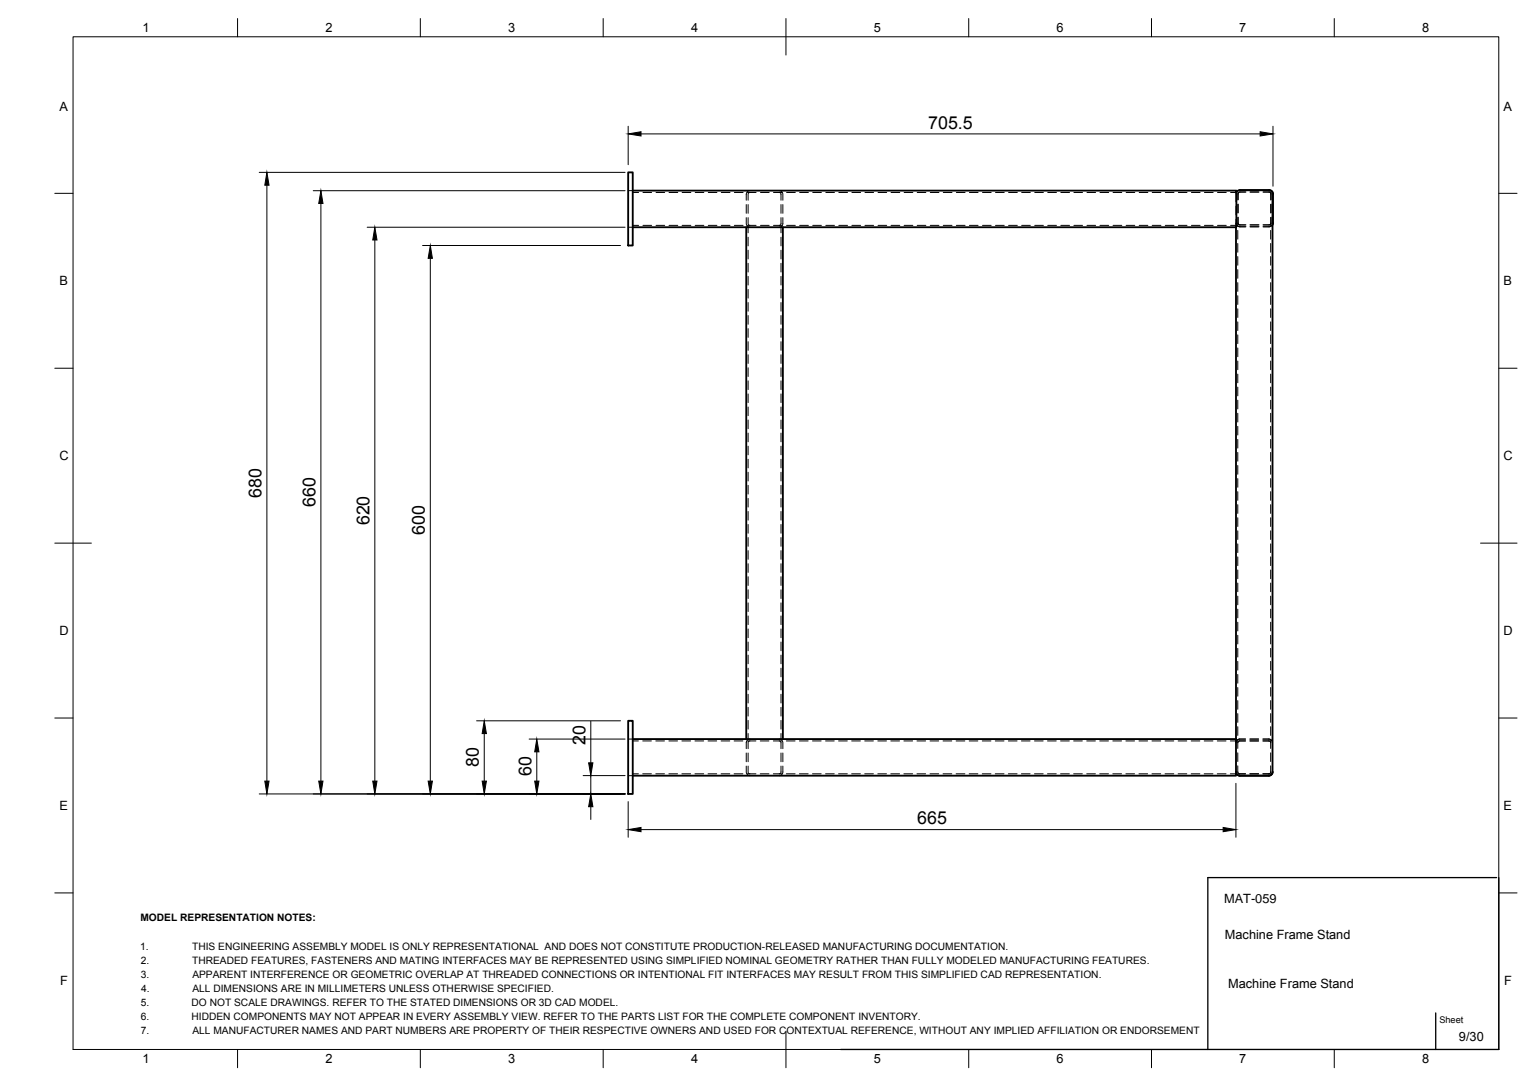
ISO-10303-21;
HEADER;
/* Generated by software containing ST-Developer
 * from STEP Tools, Inc. (www.steptools.com) 
 */

FILE_DESCRIPTION(
/* description */ ('', 'CAx-IF Rec.Pracs.---Representation and Presentation of Product Manufa
cturing Information (PMI)---4.0---2014-10-13'),
/* implementation_level */ '2;1');

FILE_NAME(
/* name */ 'Machine Frame Stand.step',
/* time_stamp */ '2026-10-28T23:00:48+01:00',
/* author */ (''),
/* organization */ (''),
/* preprocessor_version */ 'ST-DEVELOPER v20.2',
/* originating_system */ 'Autodesk Translation Framework v15.17.0.0',
/* authorisation */ '');

FILE_SCHEMA (('AP242_MANAGED_MODEL_BASED_3D_ENGINEERING_MIM_LF { 1 0 10303 442 2 1 4 }'));
ENDSEC;

DATA;
#10=MECHANICAL_DESIGN_GEOMETRIC_PRESENTATION_REPRESENTATION('',(#971,#972,#973,#974,#975,#976,#977,#978,#979,#980,#981,#982,#983,#984,#985),#61811);
#394=ELLIPSE('',#35329,5.65685424949238,4.);
#395=ELLIPSE('',#35330,5.65685424949238,4.);
#396=ELLIPSE('',#35331,5.65685424949238,4.);
#397=ELLIPSE('',#35332,5.65685424949238,4.);
#398=ELLIPSE('',#35333,2.82842712474619,2.);
#399=ELLIPSE('',#35334,2.82842712474619,2.);
#400=ELLIPSE('',#35335,2.82842712474619,2.);
#401=ELLIPSE('',#35336,2.82842712474619,2.);
#402=ELLIPSE('',#35339,2.82842712474716,2.);
#403=ELLIPSE('',#35342,2.82842712474716,2.);
#404=ELLIPSE('',#35344,5.65685424949433,4.);
#405=ELLIPSE('',#35346,5.65685424949433,4.);
#406=ELLIPSE('',#35349,5.65685424949433,4.);
#407=ELLIPSE('',#35350,5.65685424949433,4.);
#408=ELLIPSE('',#35351,2.82842712474716,2.);
#409=ELLIPSE('',#35352,2.82842712474716,2.);
#410=ELLIPSE('',#35363,5.65685424949238,4.);
#411=ELLIPSE('',#35364,5.65685424949238,4.);
#412=ELLIPSE('',#35365,5.65685424949238,4.);
#413=ELLIPSE('',#35366,5.65685424949238,4.);
#414=ELLIPSE('',#35367,2.82842712474619,2.);
#415=ELLIPSE('',#35368,2.82842712474619,2.);
#416=ELLIPSE('',#35369,2.82842712474619,2.);
#417=ELLIPSE('',#35370,2.82842712474619,2.);
#418=ELLIPSE('',#35373,2.82842712474716,2.);
#419=ELLIPSE('',#35376,2.82842712474716,2.);
#420=ELLIPSE('',#35378,5.65685424949433,4.);
#421=ELLIPSE('',#35381,5.65685424949433,4.);
#422=ELLIPSE('',#35384,5.65685424949433,4.);
#423=ELLIPSE('',#35385,5.65685424949433,4.);
#424=ELLIPSE('',#35386,2.82842712474716,2.);
#425=ELLIPSE('',#35387,2.82842712474716,2.);
#426=ELLIPSE('',#35397,5.65685424949043,4.);
#427=ELLIPSE('',#35398,5.65685424949043,4.);
#428=ELLIPSE('',#35399,5.65685424949043,4.);
#429=ELLIPSE('',#35400,5.65685424949043,4.);
#430=ELLIPSE('',#35401,2.82842712474521,2.);
#431=ELLIPSE('',#35402,2.82842712474521,2.);
#432=ELLIPSE('',#35403,2.82842712474521,2.);
#433=ELLIPSE('',#35404,2.82842712474521,2.);
#434=ELLIPSE('',#35407,2.82842712474521,2.);
#435=ELLIPSE('',#35410,2.82842712474521,2.);
#436=ELLIPSE('',#35413,5.65685424949043,4.);
#437=ELLIPSE('',#35416,5.65685424949043,4.);
#438=ELLIPSE('',#35418,5.65685424949043,4.);
#439=ELLIPSE('',#35419,5.65685424949043,4.);
#440=ELLIPSE('',#35420,2.82842712474521,2.);
#441=ELLIPSE('',#35421,2.82842712474521,2.);
#442=ELLIPSE('',#35431,5.65685424949238,4.);
#443=ELLIPSE('',#35432,5.65685424949238,4.);
#444=ELLIPSE('',#35433,5.65685424949238,4.);
#445=ELLIPSE('',#35434,5.65685424949238,4.);
#446=ELLIPSE('',#35435,2.82842712474619,2.);
#447=ELLIPSE('',#35436,2.82842712474619,2.);
#448=ELLIPSE('',#35437,2.82842712474619,2.);
#449=ELLIPSE('',#35438,2.82842712474619,2.);
#450=ELLIPSE('',#35441,2.82842712474619,2.);
#451=ELLIPSE('',#35444,2.82842712474619,2.);
#452=ELLIPSE('',#35447,5.65685424949238,4.);
#453=ELLIPSE('',#35450,5.65685424949238,4.);
#454=ELLIPSE('',#35452,5.65685424949238,4.);
#455=ELLIPSE('',#35453,5.65685424949238,4.);
#456=ELLIPSE('',#35454,2.82842712474619,2.);
#457=ELLIPSE('',#35455,2.82842712474619,2.);
#921=SHAPE_REPRESENTATION_RELATIONSHIP('SRR','None',#61979,#946);
#946=ADVANCED_BREP_SHAPE_REPRESENTATION('',(#1010,#1011,#1012,#1013,#1014,
#1015,#1016,#1017,#1018,#1019,#1020,#1021,#1022,#1023,#1024),#61792);
#971=STYLED_ITEM('',(#62135),#1010);
#972=STYLED_ITEM('',(#62135),#1011);
#973=STYLED_ITEM('',(#62135),#1012);
#974=STYLED_ITEM('',(#62135),#1013);
#975=STYLED_ITEM('',(#62135),#1014);
#976=STYLED_ITEM('',(#62135),#1015);
#977=STYLED_ITEM('',(#62135),#1016);
#978=STYLED_ITEM('',(#62135),#1017);
#979=STYLED_ITEM('',(#62135),#1018);
#980=STYLED_ITEM('',(#62135),#1019);
#981=STYLED_ITEM('',(#62135),#1020);
#982=STYLED_ITEM('',(#62135),#1021);
#983=STYLED_ITEM('',(#62135),#1022);
#984=STYLED_ITEM('',(#62135),#1023);
#985=STYLED_ITEM('',(#62135),#1024);
#1010=MANIFOLD_SOLID_BREP('Body1',#33801);
#1011=MANIFOLD_SOLID_BREP('Body2',#33802);
#1012=MANIFOLD_SOLID_BREP('Body3',#33803);
#1013=MANIFOLD_SOLID_BREP('Body4',#33804);
#1014=MANIFOLD_SOLID_BREP('Body5',#33805);
#1015=MANIFOLD_SOLID_BREP('Body6',#33806);
#1016=MANIFOLD_SOLID_BREP('Body7',#33807);
#1017=MANIFOLD_SOLID_BREP('Body8',#33808);
#1018=MANIFOLD_SOLID_BREP('Body9',#33809);
#1019=MANIFOLD_SOLID_BREP('Body10',#33810);
#1020=MANIFOLD_SOLID_BREP('Body11',#33811);
#1021=MANIFOLD_SOLID_BREP('Body12',#33812);
#1022=MANIFOLD_SOLID_BREP('Body13',#33813);
#1023=MANIFOLD_SOLID_BREP('Body14',#33814);
#1024=MANIFOLD_SOLID_BREP('Body15',#33815);
#1191=CYLINDRICAL_SURFACE('',#35193,2.);
#1192=CYLINDRICAL_SURFACE('',#35197,2.);
#1193=CYLINDRICAL_SURFACE('',#35201,4.);
#1194=CYLINDRICAL_SURFACE('',#35205,4.);
#1195=CYLINDRICAL_SURFACE('',#35209,2.);
#1196=CYLINDRICAL_SURFACE('',#35213,2.);
#1197=CYLINDRICAL_SURFACE('',#35217,4.);
#1198=CYLINDRICAL_SURFACE('',#35221,4.);
#1199=CYLINDRICAL_SURFACE('',#35227,2.);
#1200=CYLINDRICAL_SURFACE('',#35231,2.);
#1201=CYLINDRICAL_SURFACE('',#35235,4.);
#1202=CYLINDRICAL_SURFACE('',#35239,4.);
#1203=CYLINDRICAL_SURFACE('',#35243,2.);
#1204=CYLINDRICAL_SURFACE('',#35247,2.);
#1205=CYLINDRICAL_SURFACE('',#35251,4.);
#1206=CYLINDRICAL_SURFACE('',#35255,4.);
#1207=CYLINDRICAL_SURFACE('',#35261,2.);
#1208=CYLINDRICAL_SURFACE('',#35265,2.);
#1209=CYLINDRICAL_SURFACE('',#35269,4.);
#1210=CYLINDRICAL_SURFACE('',#35273,4.);
#1211=CYLINDRICAL_SURFACE('',#35277,2.);
#1212=CYLINDRICAL_SURFACE('',#35281,2.);
#1213=CYLINDRICAL_SURFACE('',#35285,4.);
#1214=CYLINDRICAL_SURFACE('',#35289,4.);
#1215=CYLINDRICAL_SURFACE('',#35295,2.);
#1216=CYLINDRICAL_SURFACE('',#35299,2.);
#1217=CYLINDRICAL_SURFACE('',#35303,4.);
#1218=CYLINDRICAL_SURFACE('',#35307,4.);
#1219=CYLINDRICAL_SURFACE('',#35311,2.);
#1220=CYLINDRICAL_SURFACE('',#35315,2.);
#1221=CYLINDRICAL_SURFACE('',#35319,4.);
#1222=CYLINDRICAL_SURFACE('',#35323,4.);
#1223=CYLINDRICAL_SURFACE('',#35338,2.);
#1224=CYLINDRICAL_SURFACE('',#35341,2.);
#1225=CYLINDRICAL_SURFACE('',#35343,4.);
#1226=CYLINDRICAL_SURFACE('',#35345,4.);
#1227=CYLINDRICAL_SURFACE('',#35354,4.);
#1228=CYLINDRICAL_SURFACE('',#35355,2.);
#1229=CYLINDRICAL_SURFACE('',#35357,2.);
#1230=CYLINDRICAL_SURFACE('',#35360,4.);
#1231=CYLINDRICAL_SURFACE('',#35372,2.);
#1232=CYLINDRICAL_SURFACE('',#35375,2.);
#1233=CYLINDRICAL_SURFACE('',#35377,4.);
#1234=CYLINDRICAL_SURFACE('',#35380,4.);
#1235=CYLINDRICAL_SURFACE('',#35389,4.);
#1236=CYLINDRICAL_SURFACE('',#35390,2.);
#1237=CYLINDRICAL_SURFACE('',#35392,2.);
#1238=CYLINDRICAL_SURFACE('',#35394,4.);
#1239=CYLINDRICAL_SURFACE('',#35406,2.);
#1240=CYLINDRICAL_SURFACE('',#35409,2.);
#1241=CYLINDRICAL_SURFACE('',#35412,4.);
#1242=CYLINDRICAL_SURFACE('',#35415,4.);
#1243=CYLINDRICAL_SURFACE('',#35424,2.);
#1244=CYLINDRICAL_SURFACE('',#35426,2.);
#1245=CYLINDRICAL_SURFACE('',#35427,4.);
#1246=CYLINDRICAL_SURFACE('',#35429,4.);
#1247=CYLINDRICAL_SURFACE('',#35440,2.);
#1248=CYLINDRICAL_SURFACE('',#35443,2.);
#1249=CYLINDRICAL_SURFACE('',#35446,4.);
#1250=CYLINDRICAL_SURFACE('',#35449,4.);
#1251=CYLINDRICAL_SURFACE('',#35458,2.);
#1252=CYLINDRICAL_SURFACE('',#35460,2.);
#1253=CYLINDRICAL_SURFACE('',#35461,4.);
#1254=CYLINDRICAL_SURFACE('',#35463,4.);
#1255=CYLINDRICAL_SURFACE('',#35465,2.);
#1256=CYLINDRICAL_SURFACE('',#35469,2.);
#1257=CYLINDRICAL_SURFACE('',#35473,4.);
#1258=CYLINDRICAL_SURFACE('',#35477,4.);
#1259=CYLINDRICAL_SURFACE('',#35481,2.);
#1260=CYLINDRICAL_SURFACE('',#35485,2.);
#1261=CYLINDRICAL_SURFACE('',#35489,4.);
#1262=CYLINDRICAL_SURFACE('',#35493,4.);
#1263=CYLINDRICAL_SURFACE('',#35499,2.);
#1264=CYLINDRICAL_SURFACE('',#35503,2.);
#1265=CYLINDRICAL_SURFACE('',#35507,4.);
#1266=CYLINDRICAL_SURFACE('',#35511,4.);
#1267=CYLINDRICAL_SURFACE('',#35515,2.);
#1268=CYLINDRICAL_SURFACE('',#35519,2.);
#1269=CYLINDRICAL_SURFACE('',#35523,4.);
#1270=CYLINDRICAL_SURFACE('',#35527,4.);
#1271=CYLINDRICAL_SURFACE('',#35533,2.);
#1272=CYLINDRICAL_SURFACE('',#35537,2.);
#1273=CYLINDRICAL_SURFACE('',#35541,4.);
#1274=CYLINDRICAL_SURFACE('',#35545,4.);
#1275=CYLINDRICAL_SURFACE('',#35549,2.);
#1276=CYLINDRICAL_SURFACE('',#35553,2.);
#1277=CYLINDRICAL_SURFACE('',#35557,4.);
#1278=CYLINDRICAL_SURFACE('',#35561,4.);
#1279=CYLINDRICAL_SURFACE('',#35566,4.);
#1280=CYLINDRICAL_SURFACE('',#35570,4.);
#1281=CYLINDRICAL_SURFACE('',#35574,4.);
#1282=CYLINDRICAL_SURFACE('',#35578,4.);
#1283=CYLINDRICAL_SURFACE('',#35582,24.0000000000018);
#1284=CYLINDRICAL_SURFACE('',#35586,24.0000000000018);
#1285=CYLINDRICAL_SURFACE('',#35590,24.0000000000018);
#1286=CYLINDRICAL_SURFACE('',#35594,24.0000000000018);
#1287=CYLINDRICAL_SURFACE('',#35600,4.);
#1288=CYLINDRICAL_SURFACE('',#35604,4.);
#1289=CYLINDRICAL_SURFACE('',#35608,4.);
#1290=CYLINDRICAL_SURFACE('',#35612,4.);
#1291=CYLINDRICAL_SURFACE('',#35616,24.0000000000018);
#1292=CYLINDRICAL_SURFACE('',#35620,24.0000000000018);
#1293=CYLINDRICAL_SURFACE('',#35624,24.0000000000018);
#1294=CYLINDRICAL_SURFACE('',#35628,24.0000000000018);
#1295=CYLINDRICAL_SURFACE('',#35634,4.);
#1296=CYLINDRICAL_SURFACE('',#35638,4.);
#1297=CYLINDRICAL_SURFACE('',#35642,4.);
#1298=CYLINDRICAL_SURFACE('',#35646,4.);
#1299=CYLINDRICAL_SURFACE('',#35650,24.0000000000018);
#1300=CYLINDRICAL_SURFACE('',#35654,24.0000000000018);
#1301=CYLINDRICAL_SURFACE('',#35658,24.0000000000018);
#1302=CYLINDRICAL_SURFACE('',#35662,24.0000000000018);
#1303=CYLINDRICAL_SURFACE('',#35668,4.);
#1304=CYLINDRICAL_SURFACE('',#35672,4.);
#1305=CYLINDRICAL_SURFACE('',#35676,4.);
#1306=CYLINDRICAL_SURFACE('',#35680,4.);
#1307=CYLINDRICAL_SURFACE('',#35684,24.0000000000018);
#1308=CYLINDRICAL_SURFACE('',#35688,24.0000000000018);
#1309=CYLINDRICAL_SURFACE('',#35692,24.0000000000018);
#1310=CYLINDRICAL_SURFACE('',#35696,24.0000000000018);
#1978=FACE_BOUND('',#6801,.T.);
#1979=FACE_BOUND('',#6803,.T.);
#1980=FACE_BOUND('',#6821,.T.);
#1981=FACE_BOUND('',#6823,.T.);
#1982=FACE_BOUND('',#6841,.T.);
#1983=FACE_BOUND('',#6843,.T.);
#1984=FACE_BOUND('',#6861,.T.);
#1985=FACE_BOUND('',#6863,.T.);
#1986=FACE_BOUND('',#6865,.T.);
#1987=FACE_BOUND('',#6874,.T.);
#1988=FACE_BOUND('',#6885,.T.);
#1989=FACE_BOUND('',#6895,.T.);
#1990=FACE_BOUND('',#6905,.T.);
#1991=FACE_BOUND('',#6915,.T.);
#1992=FACE_BOUND('',#6925,.T.);
#1993=FACE_BOUND('',#6935,.T.);
#1994=FACE_BOUND('',#6961,.T.);
#1995=FACE_BOUND('',#6963,.T.);
#1996=FACE_BOUND('',#6981,.T.);
#1997=FACE_BOUND('',#6983,.T.);
#1998=FACE_BOUND('',#7001,.T.);
#1999=FACE_BOUND('',#7003,.T.);
#2000=FACE_BOUND('',#7021,.T.);
#2001=FACE_BOUND('',#7023,.T.);
#2002=FACE_BOUND('',#7041,.T.);
#2003=FACE_BOUND('',#7043,.T.);
#2004=FACE_BOUND('',#7061,.T.);
#2005=FACE_BOUND('',#7063,.T.);
#2006=FACE_BOUND('',#7081,.T.);
#2007=FACE_BOUND('',#7083,.T.);
#2744=CIRCLE('',#35194,2.);
#2745=CIRCLE('',#35195,2.);
#2746=CIRCLE('',#35198,2.);
#2747=CIRCLE('',#35199,2.);
#2748=CIRCLE('',#35202,4.);
#2749=CIRCLE('',#35203,4.);
#2750=CIRCLE('',#35206,4.);
#2751=CIRCLE('',#35207,4.);
#2752=CIRCLE('',#35210,2.);
#2753=CIRCLE('',#35211,2.);
#2754=CIRCLE('',#35214,2.);
#2755=CIRCLE('',#35215,2.);
#2756=CIRCLE('',#35218,4.);
#2757=CIRCLE('',#35219,4.);
#2758=CIRCLE('',#35222,4.);
#2759=CIRCLE('',#35223,4.);
#2760=CIRCLE('',#35228,2.);
#2761=CIRCLE('',#35229,2.);
#2762=CIRCLE('',#35232,2.);
#2763=CIRCLE('',#35233,2.);
#2764=CIRCLE('',#35236,4.);
#2765=CIRCLE('',#35237,4.);
#2766=CIRCLE('',#35240,4.);
#2767=CIRCLE('',#35241,4.);
#2768=CIRCLE('',#35244,2.);
#2769=CIRCLE('',#35245,2.);
#2770=CIRCLE('',#35248,2.);
#2771=CIRCLE('',#35249,2.);
#2772=CIRCLE('',#35252,4.);
#2773=CIRCLE('',#35253,4.);
#2774=CIRCLE('',#35256,4.);
#2775=CIRCLE('',#35257,4.);
#2776=CIRCLE('',#35262,2.);
#2777=CIRCLE('',#35263,2.);
#2778=CIRCLE('',#35266,2.);
#2779=CIRCLE('',#35267,2.);
#2780=CIRCLE('',#35270,4.);
#2781=CIRCLE('',#35271,4.);
#2782=CIRCLE('',#35274,4.);
#2783=CIRCLE('',#35275,4.);
#2784=CIRCLE('',#35278,2.);
#2785=CIRCLE('',#35279,2.);
#2786=CIRCLE('',#35282,2.);
#2787=CIRCLE('',#35283,2.);
#2788=CIRCLE('',#35286,4.);
#2789=CIRCLE('',#35287,4.);
#2790=CIRCLE('',#35290,4.);
#2791=CIRCLE('',#35291,4.);
#2792=CIRCLE('',#35296,2.);
#2793=CIRCLE('',#35297,2.);
#2794=CIRCLE('',#35300,2.);
#2795=CIRCLE('',#35301,2.);
#2796=CIRCLE('',#35304,4.);
#2797=CIRCLE('',#35305,4.);
#2798=CIRCLE('',#35308,4.);
#2799=CIRCLE('',#35309,4.);
#2800=CIRCLE('',#35312,2.);
#2801=CIRCLE('',#35313,2.);
#2802=CIRCLE('',#35316,2.);
#2803=CIRCLE('',#35317,2.);
#2804=CIRCLE('',#35320,4.);
#2805=CIRCLE('',#35321,4.);
#2806=CIRCLE('',#35324,4.);
#2807=CIRCLE('',#35325,4.);
#2808=CIRCLE('',#35466,2.);
#2809=CIRCLE('',#35467,2.);
#2810=CIRCLE('',#35470,2.);
#2811=CIRCLE('',#35471,2.);
#2812=CIRCLE('',#35474,4.);
#2813=CIRCLE('',#35475,4.);
#2814=CIRCLE('',#35478,4.);
#2815=CIRCLE('',#35479,4.);
#2816=CIRCLE('',#35482,2.);
#2817=CIRCLE('',#35483,2.);
#2818=CIRCLE('',#35486,2.);
#2819=CIRCLE('',#35487,2.);
#2820=CIRCLE('',#35490,4.);
#2821=CIRCLE('',#35491,4.);
#2822=CIRCLE('',#35494,4.);
#2823=CIRCLE('',#35495,4.);
#2824=CIRCLE('',#35500,2.);
#2825=CIRCLE('',#35501,2.);
#2826=CIRCLE('',#35504,2.);
#2827=CIRCLE('',#35505,2.);
#2828=CIRCLE('',#35508,4.);
#2829=CIRCLE('',#35509,4.);
#2830=CIRCLE('',#35512,4.);
#2831=CIRCLE('',#35513,4.);
#2832=CIRCLE('',#35516,2.);
#2833=CIRCLE('',#35517,2.);
#2834=CIRCLE('',#35520,2.);
#2835=CIRCLE('',#35521,2.);
#2836=CIRCLE('',#35524,4.);
#2837=CIRCLE('',#35525,4.);
#2838=CIRCLE('',#35528,4.);
#2839=CIRCLE('',#35529,4.);
#2840=CIRCLE('',#35534,2.);
#2841=CIRCLE('',#35535,2.);
#2842=CIRCLE('',#35538,2.);
#2843=CIRCLE('',#35539,2.);
#2844=CIRCLE('',#35542,4.);
#2845=CIRCLE('',#35543,4.);
#2846=CIRCLE('',#35546,4.);
#2847=CIRCLE('',#35547,4.);
#2848=CIRCLE('',#35550,2.);
#2849=CIRCLE('',#35551,2.);
#2850=CIRCLE('',#35554,2.);
#2851=CIRCLE('',#35555,2.);
#2852=CIRCLE('',#35558,4.);
#2853=CIRCLE('',#35559,4.);
#2854=CIRCLE('',#35562,4.);
#2855=CIRCLE('',#35563,4.);
#2856=CIRCLE('',#35567,4.);
#2857=CIRCLE('',#35568,4.);
#2858=CIRCLE('',#35571,4.);
#2859=CIRCLE('',#35572,4.);
#2860=CIRCLE('',#35575,4.);
#2861=CIRCLE('',#35576,4.);
#2862=CIRCLE('',#35579,4.);
#2863=CIRCLE('',#35580,4.);
#2864=CIRCLE('',#35583,24.0000000000018);
#2865=CIRCLE('',#35584,24.0000000000018);
#2866=CIRCLE('',#35587,24.0000000000018);
#2867=CIRCLE('',#35588,24.0000000000018);
#2868=CIRCLE('',#35591,24.0000000000018);
#2869=CIRCLE('',#35592,24.0000000000018);
#2870=CIRCLE('',#35595,24.0000000000018);
#2871=CIRCLE('',#35596,24.0000000000018);
#2872=CIRCLE('',#35601,4.);
#2873=CIRCLE('',#35602,4.);
#2874=CIRCLE('',#35605,4.);
#2875=CIRCLE('',#35606,4.);
#2876=CIRCLE('',#35609,4.);
#2877=CIRCLE('',#35610,4.);
#2878=CIRCLE('',#35613,4.);
#2879=CIRCLE('',#35614,4.);
#2880=CIRCLE('',#35617,24.0000000000018);
#2881=CIRCLE('',#35618,24.0000000000018);
#2882=CIRCLE('',#35621,24.0000000000018);
#2883=CIRCLE('',#35622,24.0000000000018);
#2884=CIRCLE('',#35625,24.0000000000018);
#2885=CIRCLE('',#35626,24.0000000000018);
#2886=CIRCLE('',#35629,24.0000000000018);
#2887=CIRCLE('',#35630,24.0000000000018);
#2888=CIRCLE('',#35635,4.);
#2889=CIRCLE('',#35636,4.);
#2890=CIRCLE('',#35639,4.);
#2891=CIRCLE('',#35640,4.);
#2892=CIRCLE('',#35643,4.);
#2893=CIRCLE('',#35644,4.);
#2894=CIRCLE('',#35647,4.);
#2895=CIRCLE('',#35648,4.);
#2896=CIRCLE('',#35651,24.0000000000018);
#2897=CIRCLE('',#35652,24.0000000000018);
#2898=CIRCLE('',#35655,24.0000000000018);
#2899=CIRCLE('',#35656,24.0000000000018);
#2900=CIRCLE('',#35659,24.0000000000018);
#2901=CIRCLE('',#35660,24.0000000000018);
#2902=CIRCLE('',#35663,24.0000000000018);
#2903=CIRCLE('',#35664,24.0000000000018);
#2904=CIRCLE('',#35669,4.);
#2905=CIRCLE('',#35670,4.);
#2906=CIRCLE('',#35673,4.);
#2907=CIRCLE('',#35674,4.);
#2908=CIRCLE('',#35677,4.);
#2909=CIRCLE('',#35678,4.);
#2910=CIRCLE('',#35681,4.);
#2911=CIRCLE('',#35682,4.);
#2912=CIRCLE('',#35685,24.0000000000018);
#2913=CIRCLE('',#35686,24.0000000000018);
#2914=CIRCLE('',#35689,24.0000000000018);
#2915=CIRCLE('',#35690,24.0000000000018);
#2916=CIRCLE('',#35693,24.0000000000018);
#2917=CIRCLE('',#35694,24.0000000000018);
#2918=CIRCLE('',#35697,24.0000000000018);
#2919=CIRCLE('',#35698,24.0000000000018);
#4806=FACE_OUTER_BOUND('',#6784,.T.);
#4807=FACE_OUTER_BOUND('',#6785,.T.);
#4808=FACE_OUTER_BOUND('',#6786,.T.);
#4809=FACE_OUTER_BOUND('',#6787,.T.);
#4810=FACE_OUTER_BOUND('',#6788,.T.);
#4811=FACE_OUTER_BOUND('',#6789,.T.);
#4812=FACE_OUTER_BOUND('',#6790,.T.);
#4813=FACE_OUTER_BOUND('',#6791,.T.);
#4814=FACE_OUTER_BOUND('',#6792,.T.);
#4815=FACE_OUTER_BOUND('',#6793,.T.);
#4816=FACE_OUTER_BOUND('',#6794,.T.);
#4817=FACE_OUTER_BOUND('',#6795,.T.);
#4818=FACE_OUTER_BOUND('',#6796,.T.);
#4819=FACE_OUTER_BOUND('',#6797,.T.);
#4820=FACE_OUTER_BOUND('',#6798,.T.);
#4821=FACE_OUTER_BOUND('',#6799,.T.);
#4822=FACE_OUTER_BOUND('',#6800,.T.);
#4823=FACE_OUTER_BOUND('',#6802,.T.);
#4824=FACE_OUTER_BOUND('',#6804,.T.);
#4825=FACE_OUTER_BOUND('',#6805,.T.);
#4826=FACE_OUTER_BOUND('',#6806,.T.);
#4827=FACE_OUTER_BOUND('',#6807,.T.);
#4828=FACE_OUTER_BOUND('',#6808,.T.);
#4829=FACE_OUTER_BOUND('',#6809,.T.);
#4830=FACE_OUTER_BOUND('',#6810,.T.);
#4831=FACE_OUTER_BOUND('',#6811,.T.);
#4832=FACE_OUTER_BOUND('',#6812,.T.);
#4833=FACE_OUTER_BOUND('',#6813,.T.);
#4834=FACE_OUTER_BOUND('',#6814,.T.);
#4835=FACE_OUTER_BOUND('',#6815,.T.);
#4836=FACE_OUTER_BOUND('',#6816,.T.);
#4837=FACE_OUTER_BOUND('',#6817,.T.);
#4838=FACE_OUTER_BOUND('',#6818,.T.);
#4839=FACE_OUTER_BOUND('',#6819,.T.);
#4840=FACE_OUTER_BOUND('',#6820,.T.);
#4841=FACE_OUTER_BOUND('',#6822,.T.);
#4842=FACE_OUTER_BOUND('',#6824,.T.);
#4843=FACE_OUTER_BOUND('',#6825,.T.);
#4844=FACE_OUTER_BOUND('',#6826,.T.);
#4845=FACE_OUTER_BOUND('',#6827,.T.);
#4846=FACE_OUTER_BOUND('',#6828,.T.);
#4847=FACE_OUTER_BOUND('',#6829,.T.);
#4848=FACE_OUTER_BOUND('',#6830,.T.);
#4849=FACE_OUTER_BOUND('',#6831,.T.);
#4850=FACE_OUTER_BOUND('',#6832,.T.);
#4851=FACE_OUTER_BOUND('',#6833,.T.);
#4852=FACE_OUTER_BOUND('',#6834,.T.);
#4853=FACE_OUTER_BOUND('',#6835,.T.);
#4854=FACE_OUTER_BOUND('',#6836,.T.);
#4855=FACE_OUTER_BOUND('',#6837,.T.);
#4856=FACE_OUTER_BOUND('',#6838,.T.);
#4857=FACE_OUTER_BOUND('',#6839,.T.);
#4858=FACE_OUTER_BOUND('',#6840,.T.);
#4859=FACE_OUTER_BOUND('',#6842,.T.);
#4860=FACE_OUTER_BOUND('',#6844,.T.);
#4861=FACE_OUTER_BOUND('',#6845,.T.);
#4862=FACE_OUTER_BOUND('',#6846,.T.);
#4863=FACE_OUTER_BOUND('',#6847,.T.);
#4864=FACE_OUTER_BOUND('',#6848,.T.);
#4865=FACE_OUTER_BOUND('',#6849,.T.);
#4866=FACE_OUTER_BOUND('',#6850,.T.);
#4867=FACE_OUTER_BOUND('',#6851,.T.);
#4868=FACE_OUTER_BOUND('',#6852,.T.);
#4869=FACE_OUTER_BOUND('',#6853,.T.);
#4870=FACE_OUTER_BOUND('',#6854,.T.);
#4871=FACE_OUTER_BOUND('',#6855,.T.);
#4872=FACE_OUTER_BOUND('',#6856,.T.);
#4873=FACE_OUTER_BOUND('',#6857,.T.);
#4874=FACE_OUTER_BOUND('',#6858,.T.);
#4875=FACE_OUTER_BOUND('',#6859,.T.);
#4876=FACE_OUTER_BOUND('',#6860,.T.);
#4877=FACE_OUTER_BOUND('',#6862,.T.);
#4878=FACE_OUTER_BOUND('',#6864,.T.);
#4879=FACE_OUTER_BOUND('',#6866,.T.);
#4880=FACE_OUTER_BOUND('',#6867,.T.);
#4881=FACE_OUTER_BOUND('',#6868,.T.);
#4882=FACE_OUTER_BOUND('',#6869,.T.);
#4883=FACE_OUTER_BOUND('',#6870,.T.);
#4884=FACE_OUTER_BOUND('',#6871,.T.);
#4885=FACE_OUTER_BOUND('',#6872,.T.);
#4886=FACE_OUTER_BOUND('',#6873,.T.);
#4887=FACE_OUTER_BOUND('',#6875,.T.);
#4888=FACE_OUTER_BOUND('',#6876,.T.);
#4889=FACE_OUTER_BOUND('',#6877,.T.);
#4890=FACE_OUTER_BOUND('',#6878,.T.);
#4891=FACE_OUTER_BOUND('',#6879,.T.);
#4892=FACE_OUTER_BOUND('',#6880,.T.);
#4893=FACE_OUTER_BOUND('',#6881,.T.);
#4894=FACE_OUTER_BOUND('',#6882,.T.);
#4895=FACE_OUTER_BOUND('',#6883,.T.);
#4896=FACE_OUTER_BOUND('',#6884,.T.);
#4897=FACE_OUTER_BOUND('',#6886,.T.);
#4898=FACE_OUTER_BOUND('',#6887,.T.);
#4899=FACE_OUTER_BOUND('',#6888,.T.);
#4900=FACE_OUTER_BOUND('',#6889,.T.);
#4901=FACE_OUTER_BOUND('',#6890,.T.);
#4902=FACE_OUTER_BOUND('',#6891,.T.);
#4903=FACE_OUTER_BOUND('',#6892,.T.);
#4904=FACE_OUTER_BOUND('',#6893,.T.);
#4905=FACE_OUTER_BOUND('',#6894,.T.);
#4906=FACE_OUTER_BOUND('',#6896,.T.);
#4907=FACE_OUTER_BOUND('',#6897,.T.);
#4908=FACE_OUTER_BOUND('',#6898,.T.);
#4909=FACE_OUTER_BOUND('',#6899,.T.);
#4910=FACE_OUTER_BOUND('',#6900,.T.);
#4911=FACE_OUTER_BOUND('',#6901,.T.);
#4912=FACE_OUTER_BOUND('',#6902,.T.);
#4913=FACE_OUTER_BOUND('',#6903,.T.);
#4914=FACE_OUTER_BOUND('',#6904,.T.);
#4915=FACE_OUTER_BOUND('',#6906,.T.);
#4916=FACE_OUTER_BOUND('',#6907,.T.);
#4917=FACE_OUTER_BOUND('',#6908,.T.);
#4918=FACE_OUTER_BOUND('',#6909,.T.);
#4919=FACE_OUTER_BOUND('',#6910,.T.);
#4920=FACE_OUTER_BOUND('',#6911,.T.);
#4921=FACE_OUTER_BOUND('',#6912,.T.);
#4922=FACE_OUTER_BOUND('',#6913,.T.);
#4923=FACE_OUTER_BOUND('',#6914,.T.);
#4924=FACE_OUTER_BOUND('',#6916,.T.);
#4925=FACE_OUTER_BOUND('',#6917,.T.);
#4926=FACE_OUTER_BOUND('',#6918,.T.);
#4927=FACE_OUTER_BOUND('',#6919,.T.);
#4928=FACE_OUTER_BOUND('',#6920,.T.);
#4929=FACE_OUTER_BOUND('',#6921,.T.);
#4930=FACE_OUTER_BOUND('',#6922,.T.);
#4931=FACE_OUTER_BOUND('',#6923,.T.);
#4932=FACE_OUTER_BOUND('',#6924,.T.);
#4933=FACE_OUTER_BOUND('',#6926,.T.);
#4934=FACE_OUTER_BOUND('',#6927,.T.);
#4935=FACE_OUTER_BOUND('',#6928,.T.);
#4936=FACE_OUTER_BOUND('',#6929,.T.);
#4937=FACE_OUTER_BOUND('',#6930,.T.);
#4938=FACE_OUTER_BOUND('',#6931,.T.);
#4939=FACE_OUTER_BOUND('',#6932,.T.);
#4940=FACE_OUTER_BOUND('',#6933,.T.);
#4941=FACE_OUTER_BOUND('',#6934,.T.);
#4942=FACE_OUTER_BOUND('',#6936,.T.);
#4943=FACE_OUTER_BOUND('',#6937,.T.);
#4944=FACE_OUTER_BOUND('',#6938,.T.);
#4945=FACE_OUTER_BOUND('',#6939,.T.);
#4946=FACE_OUTER_BOUND('',#6940,.T.);
#4947=FACE_OUTER_BOUND('',#6941,.T.);
#4948=FACE_OUTER_BOUND('',#6942,.T.);
#4949=FACE_OUTER_BOUND('',#6943,.T.);
#4950=FACE_OUTER_BOUND('',#6944,.T.);
#4951=FACE_OUTER_BOUND('',#6945,.T.);
#4952=FACE_OUTER_BOUND('',#6946,.T.);
#4953=FACE_OUTER_BOUND('',#6947,.T.);
#4954=FACE_OUTER_BOUND('',#6948,.T.);
#4955=FACE_OUTER_BOUND('',#6949,.T.);
#4956=FACE_OUTER_BOUND('',#6950,.T.);
#4957=FACE_OUTER_BOUND('',#6951,.T.);
#4958=FACE_OUTER_BOUND('',#6952,.T.);
#4959=FACE_OUTER_BOUND('',#6953,.T.);
#4960=FACE_OUTER_BOUND('',#6954,.T.);
#4961=FACE_OUTER_BOUND('',#6955,.T.);
#4962=FACE_OUTER_BOUND('',#6956,.T.);
#4963=FACE_OUTER_BOUND('',#6957,.T.);
#4964=FACE_OUTER_BOUND('',#6958,.T.);
#4965=FACE_OUTER_BOUND('',#6959,.T.);
#4966=FACE_OUTER_BOUND('',#6960,.T.);
#4967=FACE_OUTER_BOUND('',#6962,.T.);
#4968=FACE_OUTER_BOUND('',#6964,.T.);
#4969=FACE_OUTER_BOUND('',#6965,.T.);
#4970=FACE_OUTER_BOUND('',#6966,.T.);
#4971=FACE_OUTER_BOUND('',#6967,.T.);
#4972=FACE_OUTER_BOUND('',#6968,.T.);
#4973=FACE_OUTER_BOUND('',#6969,.T.);
#4974=FACE_OUTER_BOUND('',#6970,.T.);
#4975=FACE_OUTER_BOUND('',#6971,.T.);
#4976=FACE_OUTER_BOUND('',#6972,.T.);
#4977=FACE_OUTER_BOUND('',#6973,.T.);
#4978=FACE_OUTER_BOUND('',#6974,.T.);
#4979=FACE_OUTER_BOUND('',#6975,.T.);
#4980=FACE_OUTER_BOUND('',#6976,.T.);
#4981=FACE_OUTER_BOUND('',#6977,.T.);
#4982=FACE_OUTER_BOUND('',#6978,.T.);
#4983=FACE_OUTER_BOUND('',#6979,.T.);
#4984=FACE_OUTER_BOUND('',#6980,.T.);
#4985=FACE_OUTER_BOUND('',#6982,.T.);
#4986=FACE_OUTER_BOUND('',#6984,.T.);
#4987=FACE_OUTER_BOUND('',#6985,.T.);
#4988=FACE_OUTER_BOUND('',#6986,.T.);
#4989=FACE_OUTER_BOUND('',#6987,.T.);
#4990=FACE_OUTER_BOUND('',#6988,.T.);
#4991=FACE_OUTER_BOUND('',#6989,.T.);
#4992=FACE_OUTER_BOUND('',#6990,.T.);
#4993=FACE_OUTER_BOUND('',#6991,.T.);
#4994=FACE_OUTER_BOUND('',#6992,.T.);
#4995=FACE_OUTER_BOUND('',#6993,.T.);
#4996=FACE_OUTER_BOUND('',#6994,.T.);
#4997=FACE_OUTER_BOUND('',#6995,.T.);
#4998=FACE_OUTER_BOUND('',#6996,.T.);
#4999=FACE_OUTER_BOUND('',#6997,.T.);
#5000=FACE_OUTER_BOUND('',#6998,.T.);
#5001=FACE_OUTER_BOUND('',#6999,.T.);
#5002=FACE_OUTER_BOUND('',#7000,.T.);
#5003=FACE_OUTER_BOUND('',#7002,.T.);
#5004=FACE_OUTER_BOUND('',#7004,.T.);
#5005=FACE_OUTER_BOUND('',#7005,.T.);
#5006=FACE_OUTER_BOUND('',#7006,.T.);
#5007=FACE_OUTER_BOUND('',#7007,.T.);
#5008=FACE_OUTER_BOUND('',#7008,.T.);
#5009=FACE_OUTER_BOUND('',#7009,.T.);
#5010=FACE_OUTER_BOUND('',#7010,.T.);
#5011=FACE_OUTER_BOUND('',#7011,.T.);
#5012=FACE_OUTER_BOUND('',#7012,.T.);
#5013=FACE_OUTER_BOUND('',#7013,.T.);
#5014=FACE_OUTER_BOUND('',#7014,.T.);
#5015=FACE_OUTER_BOUND('',#7015,.T.);
#5016=FACE_OUTER_BOUND('',#7016,.T.);
#5017=FACE_OUTER_BOUND('',#7017,.T.);
#5018=FACE_OUTER_BOUND('',#7018,.T.);
#5019=FACE_OUTER_BOUND('',#7019,.T.);
#5020=FACE_OUTER_BOUND('',#7020,.T.);
#5021=FACE_OUTER_BOUND('',#7022,.T.);
#5022=FACE_OUTER_BOUND('',#7024,.T.);
#5023=FACE_OUTER_BOUND('',#7025,.T.);
#5024=FACE_OUTER_BOUND('',#7026,.T.);
#5025=FACE_OUTER_BOUND('',#7027,.T.);
#5026=FACE_OUTER_BOUND('',#7028,.T.);
#5027=FACE_OUTER_BOUND('',#7029,.T.);
#5028=FACE_OUTER_BOUND('',#7030,.T.);
#5029=FACE_OUTER_BOUND('',#7031,.T.);
#5030=FACE_OUTER_BOUND('',#7032,.T.);
#5031=FACE_OUTER_BOUND('',#7033,.T.);
#5032=FACE_OUTER_BOUND('',#7034,.T.);
#5033=FACE_OUTER_BOUND('',#7035,.T.);
#5034=FACE_OUTER_BOUND('',#7036,.T.);
#5035=FACE_OUTER_BOUND('',#7037,.T.);
#5036=FACE_OUTER_BOUND('',#7038,.T.);
#5037=FACE_OUTER_BOUND('',#7039,.T.);
#5038=FACE_OUTER_BOUND('',#7040,.T.);
#5039=FACE_OUTER_BOUND('',#7042,.T.);
#5040=FACE_OUTER_BOUND('',#7044,.T.);
#5041=FACE_OUTER_BOUND('',#7045,.T.);
#5042=FACE_OUTER_BOUND('',#7046,.T.);
#5043=FACE_OUTER_BOUND('',#7047,.T.);
#5044=FACE_OUTER_BOUND('',#7048,.T.);
#5045=FACE_OUTER_BOUND('',#7049,.T.);
#5046=FACE_OUTER_BOUND('',#7050,.T.);
#5047=FACE_OUTER_BOUND('',#7051,.T.);
#5048=FACE_OUTER_BOUND('',#7052,.T.);
#5049=FACE_OUTER_BOUND('',#7053,.T.);
#5050=FACE_OUTER_BOUND('',#7054,.T.);
#5051=FACE_OUTER_BOUND('',#7055,.T.);
#5052=FACE_OUTER_BOUND('',#7056,.T.);
#5053=FACE_OUTER_BOUND('',#7057,.T.);
#5054=FACE_OUTER_BOUND('',#7058,.T.);
#5055=FACE_OUTER_BOUND('',#7059,.T.);
#5056=FACE_OUTER_BOUND('',#7060,.T.);
#5057=FACE_OUTER_BOUND('',#7062,.T.);
#5058=FACE_OUTER_BOUND('',#7064,.T.);
#5059=FACE_OUTER_BOUND('',#7065,.T.);
#5060=FACE_OUTER_BOUND('',#7066,.T.);
#5061=FACE_OUTER_BOUND('',#7067,.T.);
#5062=FACE_OUTER_BOUND('',#7068,.T.);
#5063=FACE_OUTER_BOUND('',#7069,.T.);
#5064=FACE_OUTER_BOUND('',#7070,.T.);
#5065=FACE_OUTER_BOUND('',#7071,.T.);
#5066=FACE_OUTER_BOUND('',#7072,.T.);
#5067=FACE_OUTER_BOUND('',#7073,.T.);
#5068=FACE_OUTER_BOUND('',#7074,.T.);
#5069=FACE_OUTER_BOUND('',#7075,.T.);
#5070=FACE_OUTER_BOUND('',#7076,.T.);
#5071=FACE_OUTER_BOUND('',#7077,.T.);
#5072=FACE_OUTER_BOUND('',#7078,.T.);
#5073=FACE_OUTER_BOUND('',#7079,.T.);
#5074=FACE_OUTER_BOUND('',#7080,.T.);
#5075=FACE_OUTER_BOUND('',#7082,.T.);
#6784=EDGE_LOOP('',(#24214,#24215,#24216,#24217));
#6785=EDGE_LOOP('',(#24218,#24219,#24220,#24221));
#6786=EDGE_LOOP('',(#24222,#24223,#24224,#24225));
#6787=EDGE_LOOP('',(#24226,#24227,#24228,#24229));
#6788=EDGE_LOOP('',(#24230,#24231,#24232,#24233));
#6789=EDGE_LOOP('',(#24234,#24235,#24236,#24237));
#6790=EDGE_LOOP('',(#24238,#24239,#24240,#24241));
#6791=EDGE_LOOP('',(#24242,#24243,#24244,#24245));
#6792=EDGE_LOOP('',(#24246,#24247,#24248,#24249));
#6793=EDGE_LOOP('',(#24250,#24251,#24252,#24253));
#6794=EDGE_LOOP('',(#24254,#24255,#24256,#24257));
#6795=EDGE_LOOP('',(#24258,#24259,#24260,#24261));
#6796=EDGE_LOOP('',(#24262,#24263,#24264,#24265));
#6797=EDGE_LOOP('',(#24266,#24267,#24268,#24269));
#6798=EDGE_LOOP('',(#24270,#24271,#24272,#24273));
#6799=EDGE_LOOP('',(#24274,#24275,#24276,#24277));
#6800=EDGE_LOOP('',(#24278,#24279,#24280,#24281,#24282,#24283,#24284,#24285));
#6801=EDGE_LOOP('',(#24286,#24287,#24288,#24289,#24290,#24291,#24292,#24293));
#6802=EDGE_LOOP('',(#24294,#24295,#24296,#24297,#24298,#24299,#24300,#24301));
#6803=EDGE_LOOP('',(#24302,#24303,#24304,#24305,#24306,#24307,#24308,#24309));
#6804=EDGE_LOOP('',(#24310,#24311,#24312,#24313));
#6805=EDGE_LOOP('',(#24314,#24315,#24316,#24317));
#6806=EDGE_LOOP('',(#24318,#24319,#24320,#24321));
#6807=EDGE_LOOP('',(#24322,#24323,#24324,#24325));
#6808=EDGE_LOOP('',(#24326,#24327,#24328,#24329));
#6809=EDGE_LOOP('',(#24330,#24331,#24332,#24333));
#6810=EDGE_LOOP('',(#24334,#24335,#24336,#24337));
#6811=EDGE_LOOP('',(#24338,#24339,#24340,#24341));
#6812=EDGE_LOOP('',(#24342,#24343,#24344,#24345));
#6813=EDGE_LOOP('',(#24346,#24347,#24348,#24349));
#6814=EDGE_LOOP('',(#24350,#24351,#24352,#24353));
#6815=EDGE_LOOP('',(#24354,#24355,#24356,#24357));
#6816=EDGE_LOOP('',(#24358,#24359,#24360,#24361));
#6817=EDGE_LOOP('',(#24362,#24363,#24364,#24365));
#6818=EDGE_LOOP('',(#24366,#24367,#24368,#24369));
#6819=EDGE_LOOP('',(#24370,#24371,#24372,#24373));
#6820=EDGE_LOOP('',(#24374,#24375,#24376,#24377,#24378,#24379,#24380,#24381));
#6821=EDGE_LOOP('',(#24382,#24383,#24384,#24385,#24386,#24387,#24388,#24389));
#6822=EDGE_LOOP('',(#24390,#24391,#24392,#24393,#24394,#24395,#24396,#24397));
#6823=EDGE_LOOP('',(#24398,#24399,#24400,#24401,#24402,#24403,#24404,#24405));
#6824=EDGE_LOOP('',(#24406,#24407,#24408,#24409));
#6825=EDGE_LOOP('',(#24410,#24411,#24412,#24413));
#6826=EDGE_LOOP('',(#24414,#24415,#24416,#24417));
#6827=EDGE_LOOP('',(#24418,#24419,#24420,#24421));
#6828=EDGE_LOOP('',(#24422,#24423,#24424,#24425));
#6829=EDGE_LOOP('',(#24426,#24427,#24428,#24429));
#6830=EDGE_LOOP('',(#24430,#24431,#24432,#24433));
#6831=EDGE_LOOP('',(#24434,#24435,#24436,#24437));
#6832=EDGE_LOOP('',(#24438,#24439,#24440,#24441));
#6833=EDGE_LOOP('',(#24442,#24443,#24444,#24445));
#6834=EDGE_LOOP('',(#24446,#24447,#24448,#24449));
#6835=EDGE_LOOP('',(#24450,#24451,#24452,#24453));
#6836=EDGE_LOOP('',(#24454,#24455,#24456,#24457));
#6837=EDGE_LOOP('',(#24458,#24459,#24460,#24461));
#6838=EDGE_LOOP('',(#24462,#24463,#24464,#24465));
#6839=EDGE_LOOP('',(#24466,#24467,#24468,#24469));
#6840=EDGE_LOOP('',(#24470,#24471,#24472,#24473,#24474,#24475,#24476,#24477));
#6841=EDGE_LOOP('',(#24478,#24479,#24480,#24481,#24482,#24483,#24484,#24485));
#6842=EDGE_LOOP('',(#24486,#24487,#24488,#24489,#24490,#24491,#24492,#24493));
#6843=EDGE_LOOP('',(#24494,#24495,#24496,#24497,#24498,#24499,#24500,#24501));
#6844=EDGE_LOOP('',(#24502,#24503,#24504,#24505));
#6845=EDGE_LOOP('',(#24506,#24507,#24508,#24509));
#6846=EDGE_LOOP('',(#24510,#24511,#24512,#24513));
#6847=EDGE_LOOP('',(#24514,#24515,#24516,#24517));
#6848=EDGE_LOOP('',(#24518,#24519,#24520,#24521));
#6849=EDGE_LOOP('',(#24522,#24523,#24524,#24525));
#6850=EDGE_LOOP('',(#24526,#24527,#24528,#24529));
#6851=EDGE_LOOP('',(#24530,#24531,#24532,#24533));
#6852=EDGE_LOOP('',(#24534,#24535,#24536,#24537));
#6853=EDGE_LOOP('',(#24538,#24539,#24540,#24541));
#6854=EDGE_LOOP('',(#24542,#24543,#24544,#24545));
#6855=EDGE_LOOP('',(#24546,#24547,#24548,#24549));
#6856=EDGE_LOOP('',(#24550,#24551,#24552,#24553));
#6857=EDGE_LOOP('',(#24554,#24555,#24556,#24557));
#6858=EDGE_LOOP('',(#24558,#24559,#24560,#24561));
#6859=EDGE_LOOP('',(#24562,#24563,#24564,#24565));
#6860=EDGE_LOOP('',(#24566,#24567,#24568,#24569,#24570,#24571,#24572,#24573));
#6861=EDGE_LOOP('',(#24574,#24575,#24576,#24577,#24578,#24579,#24580,#24581));
#6862=EDGE_LOOP('',(#24582,#24583,#24584,#24585,#24586,#24587,#24588,#24589));
#6863=EDGE_LOOP('',(#24590,#24591,#24592,#24593,#24594,#24595,#24596,#24597));
#6864=EDGE_LOOP('',(#24598,#24599,#24600,#24601,#24602,#24603,#24604,#24605));
#6865=EDGE_LOOP('',(#24606,#24607,#24608,#24609,#24610,#24611,#24612,#24613));
#6866=EDGE_LOOP('',(#24614,#24615,#24616,#24617));
#6867=EDGE_LOOP('',(#24618,#24619,#24620,#24621));
#6868=EDGE_LOOP('',(#24622,#24623,#24624,#24625));
#6869=EDGE_LOOP('',(#24626,#24627,#24628,#24629));
#6870=EDGE_LOOP('',(#24630,#24631,#24632,#24633));
#6871=EDGE_LOOP('',(#24634,#24635,#24636,#24637));
#6872=EDGE_LOOP('',(#24638,#24639,#24640,#24641));
#6873=EDGE_LOOP('',(#24642,#24643,#24644,#24645,#24646,#24647,#24648,#24649));
#6874=EDGE_LOOP('',(#24650,#24651,#24652,#24653,#24654,#24655,#24656,#24657));
#6875=EDGE_LOOP('',(#24658,#24659,#24660,#24661));
#6876=EDGE_LOOP('',(#24662,#24663,#24664,#24665));
#6877=EDGE_LOOP('',(#24666,#24667,#24668,#24669));
#6878=EDGE_LOOP('',(#24670,#24671,#24672,#24673));
#6879=EDGE_LOOP('',(#24674,#24675,#24676,#24677));
#6880=EDGE_LOOP('',(#24678,#24679,#24680,#24681));
#6881=EDGE_LOOP('',(#24682,#24683,#24684,#24685));
#6882=EDGE_LOOP('',(#24686,#24687,#24688,#24689));
#6883=EDGE_LOOP('',(#24690,#24691,#24692,#24693));
#6884=EDGE_LOOP('',(#24694,#24695,#24696,#24697,#24698,#24699,#24700,#24701));
#6885=EDGE_LOOP('',(#24702,#24703,#24704,#24705,#24706,#24707,#24708,#24709));
#6886=EDGE_LOOP('',(#24710,#24711,#24712,#24713));
#6887=EDGE_LOOP('',(#24714,#24715,#24716,#24717));
#6888=EDGE_LOOP('',(#24718,#24719,#24720,#24721));
#6889=EDGE_LOOP('',(#24722,#24723,#24724,#24725));
#6890=EDGE_LOOP('',(#24726,#24727,#24728,#24729));
#6891=EDGE_LOOP('',(#24730,#24731,#24732,#24733));
#6892=EDGE_LOOP('',(#24734,#24735,#24736,#24737));
#6893=EDGE_LOOP('',(#24738,#24739,#24740,#24741));
#6894=EDGE_LOOP('',(#24742,#24743,#24744,#24745,#24746,#24747,#24748,#24749));
#6895=EDGE_LOOP('',(#24750,#24751,#24752,#24753,#24754,#24755,#24756,#24757));
#6896=EDGE_LOOP('',(#24758,#24759,#24760,#24761));
#6897=EDGE_LOOP('',(#24762,#24763,#24764,#24765));
#6898=EDGE_LOOP('',(#24766,#24767,#24768,#24769));
#6899=EDGE_LOOP('',(#24770,#24771,#24772,#24773));
#6900=EDGE_LOOP('',(#24774,#24775,#24776,#24777));
#6901=EDGE_LOOP('',(#24778,#24779,#24780,#24781));
#6902=EDGE_LOOP('',(#24782,#24783,#24784,#24785));
#6903=EDGE_LOOP('',(#24786,#24787,#24788,#24789));
#6904=EDGE_LOOP('',(#24790,#24791,#24792,#24793,#24794,#24795,#24796,#24797));
#6905=EDGE_LOOP('',(#24798,#24799,#24800,#24801,#24802,#24803,#24804,#24805));
#6906=EDGE_LOOP('',(#24806,#24807,#24808,#24809));
#6907=EDGE_LOOP('',(#24810,#24811,#24812,#24813));
#6908=EDGE_LOOP('',(#24814,#24815,#24816,#24817));
#6909=EDGE_LOOP('',(#24818,#24819,#24820,#24821));
#6910=EDGE_LOOP('',(#24822,#24823,#24824,#24825));
#6911=EDGE_LOOP('',(#24826,#24827,#24828,#24829));
#6912=EDGE_LOOP('',(#24830,#24831,#24832,#24833));
#6913=EDGE_LOOP('',(#24834,#24835,#24836,#24837));
#6914=EDGE_LOOP('',(#24838,#24839,#24840,#24841,#24842,#24843,#24844,#24845));
#6915=EDGE_LOOP('',(#24846,#24847,#24848,#24849,#24850,#24851,#24852,#24853));
#6916=EDGE_LOOP('',(#24854,#24855,#24856,#24857));
#6917=EDGE_LOOP('',(#24858,#24859,#24860,#24861));
#6918=EDGE_LOOP('',(#24862,#24863,#24864,#24865));
#6919=EDGE_LOOP('',(#24866,#24867,#24868,#24869));
#6920=EDGE_LOOP('',(#24870,#24871,#24872,#24873));
#6921=EDGE_LOOP('',(#24874,#24875,#24876,#24877));
#6922=EDGE_LOOP('',(#24878,#24879,#24880,#24881));
#6923=EDGE_LOOP('',(#24882,#24883,#24884,#24885));
#6924=EDGE_LOOP('',(#24886,#24887,#24888,#24889,#24890,#24891,#24892,#24893));
#6925=EDGE_LOOP('',(#24894,#24895,#24896,#24897,#24898,#24899,#24900,#24901));
#6926=EDGE_LOOP('',(#24902,#24903,#24904,#24905));
#6927=EDGE_LOOP('',(#24906,#24907,#24908,#24909));
#6928=EDGE_LOOP('',(#24910,#24911,#24912,#24913));
#6929=EDGE_LOOP('',(#24914,#24915,#24916,#24917));
#6930=EDGE_LOOP('',(#24918,#24919,#24920,#24921));
#6931=EDGE_LOOP('',(#24922,#24923,#24924,#24925));
#6932=EDGE_LOOP('',(#24926,#24927,#24928,#24929));
#6933=EDGE_LOOP('',(#24930,#24931,#24932,#24933));
#6934=EDGE_LOOP('',(#24934,#24935,#24936,#24937,#24938,#24939,#24940,#24941));
#6935=EDGE_LOOP('',(#24942,#24943,#24944,#24945,#24946,#24947,#24948,#24949));
#6936=EDGE_LOOP('',(#24950,#24951,#24952,#24953));
#6937=EDGE_LOOP('',(#24954,#24955,#24956,#24957));
#6938=EDGE_LOOP('',(#24958,#24959,#24960,#24961));
#6939=EDGE_LOOP('',(#24962,#24963,#24964,#24965));
#6940=EDGE_LOOP('',(#24966,#24967,#24968,#24969));
#6941=EDGE_LOOP('',(#24970,#24971,#24972,#24973));
#6942=EDGE_LOOP('',(#24974,#24975,#24976,#24977));
#6943=EDGE_LOOP('',(#24978,#24979,#24980,#24981));
#6944=EDGE_LOOP('',(#24982,#24983,#24984,#24985));
#6945=EDGE_LOOP('',(#24986,#24987,#24988,#24989));
#6946=EDGE_LOOP('',(#24990,#24991,#24992,#24993));
#6947=EDGE_LOOP('',(#24994,#24995,#24996,#24997));
#6948=EDGE_LOOP('',(#24998,#24999,#25000,#25001));
#6949=EDGE_LOOP('',(#25002,#25003,#25004,#25005));
#6950=EDGE_LOOP('',(#25006,#25007,#25008,#25009));
#6951=EDGE_LOOP('',(#25010,#25011,#25012,#25013));
#6952=EDGE_LOOP('',(#25014,#25015,#25016,#25017));
#6953=EDGE_LOOP('',(#25018,#25019,#25020,#25021));
#6954=EDGE_LOOP('',(#25022,#25023,#25024,#25025));
#6955=EDGE_LOOP('',(#25026,#25027,#25028,#25029));
#6956=EDGE_LOOP('',(#25030,#25031,#25032,#25033));
#6957=EDGE_LOOP('',(#25034,#25035,#25036,#25037));
#6958=EDGE_LOOP('',(#25038,#25039,#25040,#25041));
#6959=EDGE_LOOP('',(#25042,#25043,#25044,#25045));
#6960=EDGE_LOOP('',(#25046,#25047,#25048,#25049,#25050,#25051,#25052,#25053));
#6961=EDGE_LOOP('',(#25054,#25055,#25056,#25057,#25058,#25059,#25060,#25061));
#6962=EDGE_LOOP('',(#25062,#25063,#25064,#25065,#25066,#25067,#25068,#25069));
#6963=EDGE_LOOP('',(#25070,#25071,#25072,#25073,#25074,#25075,#25076,#25077));
#6964=EDGE_LOOP('',(#25078,#25079,#25080,#25081));
#6965=EDGE_LOOP('',(#25082,#25083,#25084,#25085));
#6966=EDGE_LOOP('',(#25086,#25087,#25088,#25089));
#6967=EDGE_LOOP('',(#25090,#25091,#25092,#25093));
#6968=EDGE_LOOP('',(#25094,#25095,#25096,#25097));
#6969=EDGE_LOOP('',(#25098,#25099,#25100,#25101));
#6970=EDGE_LOOP('',(#25102,#25103,#25104,#25105));
#6971=EDGE_LOOP('',(#25106,#25107,#25108,#25109));
#6972=EDGE_LOOP('',(#25110,#25111,#25112,#25113));
#6973=EDGE_LOOP('',(#25114,#25115,#25116,#25117));
#6974=EDGE_LOOP('',(#25118,#25119,#25120,#25121));
#6975=EDGE_LOOP('',(#25122,#25123,#25124,#25125));
#6976=EDGE_LOOP('',(#25126,#25127,#25128,#25129));
#6977=EDGE_LOOP('',(#25130,#25131,#25132,#25133));
#6978=EDGE_LOOP('',(#25134,#25135,#25136,#25137));
#6979=EDGE_LOOP('',(#25138,#25139,#25140,#25141));
#6980=EDGE_LOOP('',(#25142,#25143,#25144,#25145,#25146,#25147,#25148,#25149));
#6981=EDGE_LOOP('',(#25150,#25151,#25152,#25153,#25154,#25155,#25156,#25157));
#6982=EDGE_LOOP('',(#25158,#25159,#25160,#25161,#25162,#25163,#25164,#25165));
#6983=EDGE_LOOP('',(#25166,#25167,#25168,#25169,#25170,#25171,#25172,#25173));
#6984=EDGE_LOOP('',(#25174,#25175,#25176,#25177));
#6985=EDGE_LOOP('',(#25178,#25179,#25180,#25181));
#6986=EDGE_LOOP('',(#25182,#25183,#25184,#25185));
#6987=EDGE_LOOP('',(#25186,#25187,#25188,#25189));
#6988=EDGE_LOOP('',(#25190,#25191,#25192,#25193));
#6989=EDGE_LOOP('',(#25194,#25195,#25196,#25197));
#6990=EDGE_LOOP('',(#25198,#25199,#25200,#25201));
#6991=EDGE_LOOP('',(#25202,#25203,#25204,#25205));
#6992=EDGE_LOOP('',(#25206,#25207,#25208,#25209));
#6993=EDGE_LOOP('',(#25210,#25211,#25212,#25213));
#6994=EDGE_LOOP('',(#25214,#25215,#25216,#25217));
#6995=EDGE_LOOP('',(#25218,#25219,#25220,#25221));
#6996=EDGE_LOOP('',(#25222,#25223,#25224,#25225));
#6997=EDGE_LOOP('',(#25226,#25227,#25228,#25229));
#6998=EDGE_LOOP('',(#25230,#25231,#25232,#25233));
#6999=EDGE_LOOP('',(#25234,#25235,#25236,#25237));
#7000=EDGE_LOOP('',(#25238,#25239,#25240,#25241,#25242,#25243,#25244,#25245));
#7001=EDGE_LOOP('',(#25246,#25247,#25248,#25249,#25250,#25251,#25252,#25253));
#7002=EDGE_LOOP('',(#25254,#25255,#25256,#25257,#25258,#25259,#25260,#25261));
#7003=EDGE_LOOP('',(#25262,#25263,#25264,#25265,#25266,#25267,#25268,#25269));
#7004=EDGE_LOOP('',(#25270,#25271,#25272,#25273));
#7005=EDGE_LOOP('',(#25274,#25275,#25276,#25277));
#7006=EDGE_LOOP('',(#25278,#25279,#25280,#25281));
#7007=EDGE_LOOP('',(#25282,#25283,#25284,#25285));
#7008=EDGE_LOOP('',(#25286,#25287,#25288,#25289));
#7009=EDGE_LOOP('',(#25290,#25291,#25292,#25293));
#7010=EDGE_LOOP('',(#25294,#25295,#25296,#25297));
#7011=EDGE_LOOP('',(#25298,#25299,#25300,#25301));
#7012=EDGE_LOOP('',(#25302,#25303,#25304,#25305));
#7013=EDGE_LOOP('',(#25306,#25307,#25308,#25309));
#7014=EDGE_LOOP('',(#25310,#25311,#25312,#25313));
#7015=EDGE_LOOP('',(#25314,#25315,#25316,#25317));
#7016=EDGE_LOOP('',(#25318,#25319,#25320,#25321));
#7017=EDGE_LOOP('',(#25322,#25323,#25324,#25325));
#7018=EDGE_LOOP('',(#25326,#25327,#25328,#25329));
#7019=EDGE_LOOP('',(#25330,#25331,#25332,#25333));
#7020=EDGE_LOOP('',(#25334,#25335,#25336,#25337,#25338,#25339,#25340,#25341));
#7021=EDGE_LOOP('',(#25342,#25343,#25344,#25345,#25346,#25347,#25348,#25349));
#7022=EDGE_LOOP('',(#25350,#25351,#25352,#25353,#25354,#25355,#25356,#25357));
#7023=EDGE_LOOP('',(#25358,#25359,#25360,#25361,#25362,#25363,#25364,#25365));
#7024=EDGE_LOOP('',(#25366,#25367,#25368,#25369));
#7025=EDGE_LOOP('',(#25370,#25371,#25372,#25373));
#7026=EDGE_LOOP('',(#25374,#25375,#25376,#25377));
#7027=EDGE_LOOP('',(#25378,#25379,#25380,#25381));
#7028=EDGE_LOOP('',(#25382,#25383,#25384,#25385));
#7029=EDGE_LOOP('',(#25386,#25387,#25388,#25389));
#7030=EDGE_LOOP('',(#25390,#25391,#25392,#25393));
#7031=EDGE_LOOP('',(#25394,#25395,#25396,#25397));
#7032=EDGE_LOOP('',(#25398,#25399,#25400,#25401));
#7033=EDGE_LOOP('',(#25402,#25403,#25404,#25405));
#7034=EDGE_LOOP('',(#25406,#25407,#25408,#25409));
#7035=EDGE_LOOP('',(#25410,#25411,#25412,#25413));
#7036=EDGE_LOOP('',(#25414,#25415,#25416,#25417));
#7037=EDGE_LOOP('',(#25418,#25419,#25420,#25421));
#7038=EDGE_LOOP('',(#25422,#25423,#25424,#25425));
#7039=EDGE_LOOP('',(#25426,#25427,#25428,#25429));
#7040=EDGE_LOOP('',(#25430,#25431,#25432,#25433,#25434,#25435,#25436,#25437));
#7041=EDGE_LOOP('',(#25438,#25439,#25440,#25441,#25442,#25443,#25444,#25445));
#7042=EDGE_LOOP('',(#25446,#25447,#25448,#25449,#25450,#25451,#25452,#25453));
#7043=EDGE_LOOP('',(#25454,#25455,#25456,#25457,#25458,#25459,#25460,#25461));
#7044=EDGE_LOOP('',(#25462,#25463,#25464,#25465));
#7045=EDGE_LOOP('',(#25466,#25467,#25468,#25469));
#7046=EDGE_LOOP('',(#25470,#25471,#25472,#25473));
#7047=EDGE_LOOP('',(#25474,#25475,#25476,#25477));
#7048=EDGE_LOOP('',(#25478,#25479,#25480,#25481));
#7049=EDGE_LOOP('',(#25482,#25483,#25484,#25485));
#7050=EDGE_LOOP('',(#25486,#25487,#25488,#25489));
#7051=EDGE_LOOP('',(#25490,#25491,#25492,#25493));
#7052=EDGE_LOOP('',(#25494,#25495,#25496,#25497));
#7053=EDGE_LOOP('',(#25498,#25499,#25500,#25501));
#7054=EDGE_LOOP('',(#25502,#25503,#25504,#25505));
#7055=EDGE_LOOP('',(#25506,#25507,#25508,#25509));
#7056=EDGE_LOOP('',(#25510,#25511,#25512,#25513));
#7057=EDGE_LOOP('',(#25514,#25515,#25516,#25517));
#7058=EDGE_LOOP('',(#25518,#25519,#25520,#25521));
#7059=EDGE_LOOP('',(#25522,#25523,#25524,#25525));
#7060=EDGE_LOOP('',(#25526,#25527,#25528,#25529,#25530,#25531,#25532,#25533));
#7061=EDGE_LOOP('',(#25534,#25535,#25536,#25537,#25538,#25539,#25540,#25541));
#7062=EDGE_LOOP('',(#25542,#25543,#25544,#25545,#25546,#25547,#25548,#25549));
#7063=EDGE_LOOP('',(#25550,#25551,#25552,#25553,#25554,#25555,#25556,#25557));
#7064=EDGE_LOOP('',(#25558,#25559,#25560,#25561));
#7065=EDGE_LOOP('',(#25562,#25563,#25564,#25565));
#7066=EDGE_LOOP('',(#25566,#25567,#25568,#25569));
#7067=EDGE_LOOP('',(#25570,#25571,#25572,#25573));
#7068=EDGE_LOOP('',(#25574,#25575,#25576,#25577));
#7069=EDGE_LOOP('',(#25578,#25579,#25580,#25581));
#7070=EDGE_LOOP('',(#25582,#25583,#25584,#25585));
#7071=EDGE_LOOP('',(#25586,#25587,#25588,#25589));
#7072=EDGE_LOOP('',(#25590,#25591,#25592,#25593));
#7073=EDGE_LOOP('',(#25594,#25595,#25596,#25597));
#7074=EDGE_LOOP('',(#25598,#25599,#25600,#25601));
#7075=EDGE_LOOP('',(#25602,#25603,#25604,#25605));
#7076=EDGE_LOOP('',(#25606,#25607,#25608,#25609));
#7077=EDGE_LOOP('',(#25610,#25611,#25612,#25613));
#7078=EDGE_LOOP('',(#25614,#25615,#25616,#25617));
#7079=EDGE_LOOP('',(#25618,#25619,#25620,#25621));
#7080=EDGE_LOOP('',(#25622,#25623,#25624,#25625,#25626,#25627,#25628,#25629));
#7081=EDGE_LOOP('',(#25630,#25631,#25632,#25633,#25634,#25635,#25636,#25637));
#7082=EDGE_LOOP('',(#25638,#25639,#25640,#25641,#25642,#25643,#25644,#25645));
#7083=EDGE_LOOP('',(#25646,#25647,#25648,#25649,#25650,#25651,#25652,#25653));
#9101=LINE('',#53785,#11648);
#9102=LINE('',#53787,#11649);
#9103=LINE('',#53789,#11650);
#9104=LINE('',#53790,#11651);
#9105=LINE('',#53795,#11652);
#9106=LINE('',#53799,#11653);
#9107=LINE('',#53801,#11654);
#9108=LINE('',#53802,#11655);
#9109=LINE('',#53807,#11656);
#9110=LINE('',#53812,#11657);
#9111=LINE('',#53814,#11658);
#9112=LINE('',#53816,#11659);
#9113=LINE('',#53817,#11660);
#9114=LINE('',#53822,#11661);
#9115=LINE('',#53826,#11662);
#9116=LINE('',#53828,#11663);
#9117=LINE('',#53829,#11664);
#9118=LINE('',#53834,#11665);
#9119=LINE('',#53838,#11666);
#9120=LINE('',#53840,#11667);
#9121=LINE('',#53841,#11668);
#9122=LINE('',#53847,#11669);
#9123=LINE('',#53850,#11670);
#9124=LINE('',#53852,#11671);
#9125=LINE('',#53853,#11672);
#9126=LINE('',#53859,#11673);
#9127=LINE('',#53861,#11674);
#9128=LINE('',#53862,#11675);
#9129=LINE('',#53867,#11676);
#9130=LINE('',#53871,#11677);
#9131=LINE('',#53873,#11678);
#9132=LINE('',#53874,#11679);
#9133=LINE('',#53883,#11680);
#9134=LINE('',#53885,#11681);
#9135=LINE('',#53887,#11682);
#9136=LINE('',#53888,#11683);
#9137=LINE('',#53893,#11684);
#9138=LINE('',#53897,#11685);
#9139=LINE('',#53899,#11686);
#9140=LINE('',#53900,#11687);
#9141=LINE('',#53905,#11688);
#9142=LINE('',#53910,#11689);
#9143=LINE('',#53912,#11690);
#9144=LINE('',#53914,#11691);
#9145=LINE('',#53915,#11692);
#9146=LINE('',#53920,#11693);
#9147=LINE('',#53924,#11694);
#9148=LINE('',#53926,#11695);
#9149=LINE('',#53927,#11696);
#9150=LINE('',#53932,#11697);
#9151=LINE('',#53936,#11698);
#9152=LINE('',#53938,#11699);
#9153=LINE('',#53939,#11700);
#9154=LINE('',#53945,#11701);
#9155=LINE('',#53948,#11702);
#9156=LINE('',#53950,#11703);
#9157=LINE('',#53951,#11704);
#9158=LINE('',#53957,#11705);
#9159=LINE('',#53959,#11706);
#9160=LINE('',#53960,#11707);
#9161=LINE('',#53965,#11708);
#9162=LINE('',#53969,#11709);
#9163=LINE('',#53971,#11710);
#9164=LINE('',#53972,#11711);
#9165=LINE('',#53981,#11712);
#9166=LINE('',#53983,#11713);
#9167=LINE('',#53985,#11714);
#9168=LINE('',#53986,#11715);
#9169=LINE('',#53991,#11716);
#9170=LINE('',#53995,#11717);
#9171=LINE('',#53997,#11718);
#9172=LINE('',#53998,#11719);
#9173=LINE('',#54003,#11720);
#9174=LINE('',#54008,#11721);
#9175=LINE('',#54010,#11722);
#9176=LINE('',#54012,#11723);
#9177=LINE('',#54013,#11724);
#9178=LINE('',#54018,#11725);
#9179=LINE('',#54022,#11726);
#9180=LINE('',#54024,#11727);
#9181=LINE('',#54025,#11728);
#9182=LINE('',#54030,#11729);
#9183=LINE('',#54034,#11730);
#9184=LINE('',#54036,#11731);
#9185=LINE('',#54037,#11732);
#9186=LINE('',#54043,#11733);
#9187=LINE('',#54046,#11734);
#9188=LINE('',#54048,#11735);
#9189=LINE('',#54049,#11736);
#9190=LINE('',#54055,#11737);
#9191=LINE('',#54057,#11738);
#9192=LINE('',#54058,#11739);
#9193=LINE('',#54063,#11740);
#9194=LINE('',#54067,#11741);
#9195=LINE('',#54069,#11742);
#9196=LINE('',#54070,#11743);
#9197=LINE('',#54079,#11744);
#9198=LINE('',#54081,#11745);
#9199=LINE('',#54083,#11746);
#9200=LINE('',#54084,#11747);
#9201=LINE('',#54089,#11748);
#9202=LINE('',#54093,#11749);
#9203=LINE('',#54095,#11750);
#9204=LINE('',#54096,#11751);
#9205=LINE('',#54101,#11752);
#9206=LINE('',#54106,#11753);
#9207=LINE('',#54108,#11754);
#9208=LINE('',#54110,#11755);
#9209=LINE('',#54111,#11756);
#9210=LINE('',#54116,#11757);
#9211=LINE('',#54120,#11758);
#9212=LINE('',#54122,#11759);
#9213=LINE('',#54123,#11760);
#9214=LINE('',#54128,#11761);
#9215=LINE('',#54132,#11762);
#9216=LINE('',#54134,#11763);
#9217=LINE('',#54135,#11764);
#9218=LINE('',#54141,#11765);
#9219=LINE('',#54144,#11766);
#9220=LINE('',#54146,#11767);
#9221=LINE('',#54147,#11768);
#9222=LINE('',#54153,#11769);
#9223=LINE('',#54155,#11770);
#9224=LINE('',#54156,#11771);
#9225=LINE('',#54161,#11772);
#9226=LINE('',#54165,#11773);
#9227=LINE('',#54167,#11774);
#9228=LINE('',#54168,#11775);
#9229=LINE('',#54179,#11776);
#9230=LINE('',#54183,#11777);
#9231=LINE('',#54187,#11778);
#9232=LINE('',#54190,#11779);
#9233=LINE('',#54193,#11780);
#9234=LINE('',#54197,#11781);
#9235=LINE('',#54201,#11782);
#9236=LINE('',#54205,#11783);
#9237=LINE('',#54209,#11784);
#9238=LINE('',#54211,#11785);
#9239=LINE('',#54212,#11786);
#9240=LINE('',#54215,#11787);
#9241=LINE('',#54219,#11788);
#9242=LINE('',#54220,#11789);
#9243=LINE('',#54223,#11790);
#9244=LINE('',#54227,#11791);
#9245=LINE('',#54230,#11792);
#9246=LINE('',#54233,#11793);
#9247=LINE('',#54236,#11794);
#9248=LINE('',#54239,#11795);
#9249=LINE('',#54240,#11796);
#9250=LINE('',#54242,#11797);
#9251=LINE('',#54246,#11798);
#9252=LINE('',#54249,#11799);
#9253=LINE('',#54251,#11800);
#9254=LINE('',#54255,#11801);
#9255=LINE('',#54258,#11802);
#9256=LINE('',#54260,#11803);
#9257=LINE('',#54262,#11804);
#9258=LINE('',#54264,#11805);
#9259=LINE('',#54268,#11806);
#9260=LINE('',#54270,#11807);
#9261=LINE('',#54277,#11808);
#9262=LINE('',#54281,#11809);
#9263=LINE('',#54285,#11810);
#9264=LINE('',#54288,#11811);
#9265=LINE('',#54291,#11812);
#9266=LINE('',#54295,#11813);
#9267=LINE('',#54299,#11814);
#9268=LINE('',#54303,#11815);
#9269=LINE('',#54307,#11816);
#9270=LINE('',#54309,#11817);
#9271=LINE('',#54310,#11818);
#9272=LINE('',#54313,#11819);
#9273=LINE('',#54317,#11820);
#9274=LINE('',#54318,#11821);
#9275=LINE('',#54321,#11822);
#9276=LINE('',#54325,#11823);
#9277=LINE('',#54328,#11824);
#9278=LINE('',#54331,#11825);
#9279=LINE('',#54332,#11826);
#9280=LINE('',#54335,#11827);
#9281=LINE('',#54339,#11828);
#9282=LINE('',#54340,#11829);
#9283=LINE('',#54345,#11830);
#9284=LINE('',#54348,#11831);
#9285=LINE('',#54350,#11832);
#9286=LINE('',#54354,#11833);
#9287=LINE('',#54357,#11834);
#9288=LINE('',#54359,#11835);
#9289=LINE('',#54361,#11836);
#9290=LINE('',#54363,#11837);
#9291=LINE('',#54366,#11838);
#9292=LINE('',#54368,#11839);
#9293=LINE('',#54373,#11840);
#9294=LINE('',#54377,#11841);
#9295=LINE('',#54381,#11842);
#9296=LINE('',#54385,#11843);
#9297=LINE('',#54389,#11844);
#9298=LINE('',#54393,#11845);
#9299=LINE('',#54397,#11846);
#9300=LINE('',#54401,#11847);
#9301=LINE('',#54405,#11848);
#9302=LINE('',#54407,#11849);
#9303=LINE('',#54408,#11850);
#9304=LINE('',#54411,#11851);
#9305=LINE('',#54415,#11852);
#9306=LINE('',#54416,#11853);
#9307=LINE('',#54419,#11854);
#9308=LINE('',#54423,#11855);
#9309=LINE('',#54425,#11856);
#9310=LINE('',#54426,#11857);
#9311=LINE('',#54429,#11858);
#9312=LINE('',#54433,#11859);
#9313=LINE('',#54434,#11860);
#9314=LINE('',#54437,#11861);
#9315=LINE('',#54441,#11862);
#9316=LINE('',#54445,#11863);
#9317=LINE('',#54448,#11864);
#9318=LINE('',#54452,#11865);
#9319=LINE('',#54455,#11866);
#9320=LINE('',#54457,#11867);
#9321=LINE('',#54459,#11868);
#9322=LINE('',#54461,#11869);
#9323=LINE('',#54464,#11870);
#9324=LINE('',#54466,#11871);
#9325=LINE('',#54471,#11872);
#9326=LINE('',#54475,#11873);
#9327=LINE('',#54479,#11874);
#9328=LINE('',#54483,#11875);
#9329=LINE('',#54487,#11876);
#9330=LINE('',#54491,#11877);
#9331=LINE('',#54495,#11878);
#9332=LINE('',#54499,#11879);
#9333=LINE('',#54503,#11880);
#9334=LINE('',#54505,#11881);
#9335=LINE('',#54506,#11882);
#9336=LINE('',#54509,#11883);
#9337=LINE('',#54513,#11884);
#9338=LINE('',#54514,#11885);
#9339=LINE('',#54517,#11886);
#9340=LINE('',#54521,#11887);
#9341=LINE('',#54523,#11888);
#9342=LINE('',#54524,#11889);
#9343=LINE('',#54527,#11890);
#9344=LINE('',#54531,#11891);
#9345=LINE('',#54532,#11892);
#9346=LINE('',#54535,#11893);
#9347=LINE('',#54539,#11894);
#9348=LINE('',#54543,#11895);
#9349=LINE('',#54546,#11896);
#9350=LINE('',#54550,#11897);
#9351=LINE('',#54553,#11898);
#9352=LINE('',#54555,#11899);
#9353=LINE('',#54557,#11900);
#9354=LINE('',#54559,#11901);
#9355=LINE('',#54562,#11902);
#9356=LINE('',#54564,#11903);
#9357=LINE('',#54569,#11904);
#9358=LINE('',#54571,#11905);
#9359=LINE('',#54573,#11906);
#9360=LINE('',#54574,#11907);
#9361=LINE('',#54579,#11908);
#9362=LINE('',#54583,#11909);
#9363=LINE('',#54585,#11910);
#9364=LINE('',#54586,#11911);
#9365=LINE('',#54591,#11912);
#9366=LINE('',#54596,#11913);
#9367=LINE('',#54598,#11914);
#9368=LINE('',#54600,#11915);
#9369=LINE('',#54601,#11916);
#9370=LINE('',#54606,#11917);
#9371=LINE('',#54610,#11918);
#9372=LINE('',#54612,#11919);
#9373=LINE('',#54613,#11920);
#9374=LINE('',#54618,#11921);
#9375=LINE('',#54622,#11922);
#9376=LINE('',#54624,#11923);
#9377=LINE('',#54625,#11924);
#9378=LINE('',#54631,#11925);
#9379=LINE('',#54634,#11926);
#9380=LINE('',#54636,#11927);
#9381=LINE('',#54637,#11928);
#9382=LINE('',#54643,#11929);
#9383=LINE('',#54645,#11930);
#9384=LINE('',#54646,#11931);
#9385=LINE('',#54651,#11932);
#9386=LINE('',#54655,#11933);
#9387=LINE('',#54657,#11934);
#9388=LINE('',#54658,#11935);
#9389=LINE('',#54667,#11936);
#9390=LINE('',#54669,#11937);
#9391=LINE('',#54671,#11938);
#9392=LINE('',#54672,#11939);
#9393=LINE('',#54677,#11940);
#9394=LINE('',#54681,#11941);
#9395=LINE('',#54683,#11942);
#9396=LINE('',#54684,#11943);
#9397=LINE('',#54689,#11944);
#9398=LINE('',#54694,#11945);
#9399=LINE('',#54696,#11946);
#9400=LINE('',#54698,#11947);
#9401=LINE('',#54699,#11948);
#9402=LINE('',#54704,#11949);
#9403=LINE('',#54708,#11950);
#9404=LINE('',#54710,#11951);
#9405=LINE('',#54711,#11952);
#9406=LINE('',#54716,#11953);
#9407=LINE('',#54720,#11954);
#9408=LINE('',#54722,#11955);
#9409=LINE('',#54723,#11956);
#9410=LINE('',#54729,#11957);
#9411=LINE('',#54732,#11958);
#9412=LINE('',#54734,#11959);
#9413=LINE('',#54735,#11960);
#9414=LINE('',#54741,#11961);
#9415=LINE('',#54743,#11962);
#9416=LINE('',#54744,#11963);
#9417=LINE('',#54749,#11964);
#9418=LINE('',#54753,#11965);
#9419=LINE('',#54755,#11966);
#9420=LINE('',#54756,#11967);
#9421=LINE('',#54765,#11968);
#9422=LINE('',#54767,#11969);
#9423=LINE('',#54769,#11970);
#9424=LINE('',#54770,#11971);
#9425=LINE('',#54775,#11972);
#9426=LINE('',#54779,#11973);
#9427=LINE('',#54781,#11974);
#9428=LINE('',#54782,#11975);
#9429=LINE('',#54787,#11976);
#9430=LINE('',#54792,#11977);
#9431=LINE('',#54794,#11978);
#9432=LINE('',#54796,#11979);
#9433=LINE('',#54797,#11980);
#9434=LINE('',#54802,#11981);
#9435=LINE('',#54806,#11982);
#9436=LINE('',#54808,#11983);
#9437=LINE('',#54809,#11984);
#9438=LINE('',#54814,#11985);
#9439=LINE('',#54818,#11986);
#9440=LINE('',#54820,#11987);
#9441=LINE('',#54821,#11988);
#9442=LINE('',#54827,#11989);
#9443=LINE('',#54830,#11990);
#9444=LINE('',#54832,#11991);
#9445=LINE('',#54833,#11992);
#9446=LINE('',#54839,#11993);
#9447=LINE('',#54841,#11994);
#9448=LINE('',#54842,#11995);
#9449=LINE('',#54847,#11996);
#9450=LINE('',#54851,#11997);
#9451=LINE('',#54853,#11998);
#9452=LINE('',#54854,#11999);
#9453=LINE('',#54865,#12000);
#9454=LINE('',#54868,#12001);
#9455=LINE('',#54871,#12002);
#9456=LINE('',#54873,#12003);
#9457=LINE('',#54874,#12004);
#9458=LINE('',#54879,#12005);
#9459=LINE('',#54883,#12006);
#9460=LINE('',#54885,#12007);
#9461=LINE('',#54886,#12008);
#9462=LINE('',#54891,#12009);
#9463=LINE('',#54895,#12010);
#9464=LINE('',#54897,#12011);
#9465=LINE('',#54898,#12012);
#9466=LINE('',#54903,#12013);
#9467=LINE('',#54906,#12014);
#9468=LINE('',#54907,#12015);
#9469=LINE('',#54913,#12016);
#9470=LINE('',#54916,#12017);
#9471=LINE('',#54919,#12018);
#9472=LINE('',#54921,#12019);
#9473=LINE('',#54922,#12020);
#9474=LINE('',#54928,#12021);
#9475=LINE('',#54931,#12022);
#9476=LINE('',#54933,#12023);
#9477=LINE('',#54934,#12024);
#9478=LINE('',#54940,#12025);
#9479=LINE('',#54943,#12026);
#9480=LINE('',#54945,#12027);
#9481=LINE('',#54946,#12028);
#9482=LINE('',#54952,#12029);
#9483=LINE('',#54954,#12030);
#9484=LINE('',#54955,#12031);
#9485=LINE('',#54963,#12032);
#9486=LINE('',#54966,#12033);
#9487=LINE('',#54969,#12034);
#9488=LINE('',#54971,#12035);
#9489=LINE('',#54972,#12036);
#9490=LINE('',#54977,#12037);
#9491=LINE('',#54981,#12038);
#9492=LINE('',#54983,#12039);
#9493=LINE('',#54984,#12040);
#9494=LINE('',#54989,#12041);
#9495=LINE('',#54993,#12042);
#9496=LINE('',#54995,#12043);
#9497=LINE('',#54996,#12044);
#9498=LINE('',#55001,#12045);
#9499=LINE('',#55004,#12046);
#9500=LINE('',#55005,#12047);
#9501=LINE('',#55011,#12048);
#9502=LINE('',#55014,#12049);
#9503=LINE('',#55017,#12050);
#9504=LINE('',#55019,#12051);
#9505=LINE('',#55020,#12052);
#9506=LINE('',#55026,#12053);
#9507=LINE('',#55029,#12054);
#9508=LINE('',#55031,#12055);
#9509=LINE('',#55032,#12056);
#9510=LINE('',#55038,#12057);
#9511=LINE('',#55041,#12058);
#9512=LINE('',#55043,#12059);
#9513=LINE('',#55044,#12060);
#9514=LINE('',#55050,#12061);
#9515=LINE('',#55052,#12062);
#9516=LINE('',#55053,#12063);
#9517=LINE('',#55061,#12064);
#9518=LINE('',#55064,#12065);
#9519=LINE('',#55067,#12066);
#9520=LINE('',#55069,#12067);
#9521=LINE('',#55070,#12068);
#9522=LINE('',#55075,#12069);
#9523=LINE('',#55079,#12070);
#9524=LINE('',#55081,#12071);
#9525=LINE('',#55082,#12072);
#9526=LINE('',#55087,#12073);
#9527=LINE('',#55091,#12074);
#9528=LINE('',#55093,#12075);
#9529=LINE('',#55094,#12076);
#9530=LINE('',#55099,#12077);
#9531=LINE('',#55102,#12078);
#9532=LINE('',#55103,#12079);
#9533=LINE('',#55109,#12080);
#9534=LINE('',#55112,#12081);
#9535=LINE('',#55115,#12082);
#9536=LINE('',#55117,#12083);
#9537=LINE('',#55118,#12084);
#9538=LINE('',#55124,#12085);
#9539=LINE('',#55127,#12086);
#9540=LINE('',#55129,#12087);
#9541=LINE('',#55130,#12088);
#9542=LINE('',#55136,#12089);
#9543=LINE('',#55139,#12090);
#9544=LINE('',#55141,#12091);
#9545=LINE('',#55142,#12092);
#9546=LINE('',#55148,#12093);
#9547=LINE('',#55150,#12094);
#9548=LINE('',#55151,#12095);
#9549=LINE('',#55159,#12096);
#9550=LINE('',#55162,#12097);
#9551=LINE('',#55165,#12098);
#9552=LINE('',#55167,#12099);
#9553=LINE('',#55168,#12100);
#9554=LINE('',#55173,#12101);
#9555=LINE('',#55177,#12102);
#9556=LINE('',#55179,#12103);
#9557=LINE('',#55180,#12104);
#9558=LINE('',#55185,#12105);
#9559=LINE('',#55189,#12106);
#9560=LINE('',#55191,#12107);
#9561=LINE('',#55192,#12108);
#9562=LINE('',#55197,#12109);
#9563=LINE('',#55200,#12110);
#9564=LINE('',#55201,#12111);
#9565=LINE('',#55207,#12112);
#9566=LINE('',#55210,#12113);
#9567=LINE('',#55213,#12114);
#9568=LINE('',#55215,#12115);
#9569=LINE('',#55216,#12116);
#9570=LINE('',#55222,#12117);
#9571=LINE('',#55225,#12118);
#9572=LINE('',#55227,#12119);
#9573=LINE('',#55228,#12120);
#9574=LINE('',#55234,#12121);
#9575=LINE('',#55237,#12122);
#9576=LINE('',#55239,#12123);
#9577=LINE('',#55240,#12124);
#9578=LINE('',#55246,#12125);
#9579=LINE('',#55248,#12126);
#9580=LINE('',#55249,#12127);
#11648=VECTOR('',#41083,10.);
#11649=VECTOR('',#41084,10.);
#11650=VECTOR('',#41085,10.);
#11651=VECTOR('',#41086,10.);
#11652=VECTOR('',#41091,10.);
#11653=VECTOR('',#41096,10.);
#11654=VECTOR('',#41097,10.);
#11655=VECTOR('',#41098,10.);
#11656=VECTOR('',#41103,10.);
#11657=VECTOR('',#41108,10.);
#11658=VECTOR('',#41109,10.);
#11659=VECTOR('',#41110,10.);
#11660=VECTOR('',#41111,10.);
#11661=VECTOR('',#41116,10.);
#11662=VECTOR('',#41121,10.);
#11663=VECTOR('',#41122,10.);
#11664=VECTOR('',#41123,10.);
#11665=VECTOR('',#41128,10.);
#11666=VECTOR('',#41133,10.);
#11667=VECTOR('',#41134,10.);
#11668=VECTOR('',#41135,10.);
#11669=VECTOR('',#41142,10.);
#11670=VECTOR('',#41145,10.);
#11671=VECTOR('',#41146,10.);
#11672=VECTOR('',#41147,10.);
#11673=VECTOR('',#41156,10.);
#11674=VECTOR('',#41157,10.);
#11675=VECTOR('',#41158,10.);
#11676=VECTOR('',#41163,10.);
#11677=VECTOR('',#41168,10.);
#11678=VECTOR('',#41169,10.);
#11679=VECTOR('',#41170,10.);
#11680=VECTOR('',#41183,10.);
#11681=VECTOR('',#41184,10.);
#11682=VECTOR('',#41185,10.);
#11683=VECTOR('',#41186,10.);
#11684=VECTOR('',#41191,10.);
#11685=VECTOR('',#41196,10.);
#11686=VECTOR('',#41197,10.);
#11687=VECTOR('',#41198,10.);
#11688=VECTOR('',#41203,10.);
#11689=VECTOR('',#41208,10.);
#11690=VECTOR('',#41209,10.);
#11691=VECTOR('',#41210,10.);
#11692=VECTOR('',#41211,10.);
#11693=VECTOR('',#41216,10.);
#11694=VECTOR('',#41221,10.);
#11695=VECTOR('',#41222,10.);
#11696=VECTOR('',#41223,10.);
#11697=VECTOR('',#41228,10.);
#11698=VECTOR('',#41233,10.);
#11699=VECTOR('',#41234,10.);
#11700=VECTOR('',#41235,10.);
#11701=VECTOR('',#41242,10.);
#11702=VECTOR('',#41245,10.);
#11703=VECTOR('',#41246,10.);
#11704=VECTOR('',#41247,10.);
#11705=VECTOR('',#41256,10.);
#11706=VECTOR('',#41257,10.);
#11707=VECTOR('',#41258,10.);
#11708=VECTOR('',#41263,10.);
#11709=VECTOR('',#41268,10.);
#11710=VECTOR('',#41269,10.);
#11711=VECTOR('',#41270,10.);
#11712=VECTOR('',#41283,10.);
#11713=VECTOR('',#41284,10.);
#11714=VECTOR('',#41285,10.);
#11715=VECTOR('',#41286,10.);
#11716=VECTOR('',#41291,10.);
#11717=VECTOR('',#41296,10.);
#11718=VECTOR('',#41297,10.);
#11719=VECTOR('',#41298,10.);
#11720=VECTOR('',#41303,10.);
#11721=VECTOR('',#41308,10.);
#11722=VECTOR('',#41309,10.);
#11723=VECTOR('',#41310,10.);
#11724=VECTOR('',#41311,10.);
#11725=VECTOR('',#41316,10.);
#11726=VECTOR('',#41321,10.);
#11727=VECTOR('',#41322,10.);
#11728=VECTOR('',#41323,10.);
#11729=VECTOR('',#41328,10.);
#11730=VECTOR('',#41333,10.);
#11731=VECTOR('',#41334,10.);
#11732=VECTOR('',#41335,10.);
#11733=VECTOR('',#41342,10.);
#11734=VECTOR('',#41345,10.);
#11735=VECTOR('',#41346,10.);
#11736=VECTOR('',#41347,10.);
#11737=VECTOR('',#41356,10.);
#11738=VECTOR('',#41357,10.);
#11739=VECTOR('',#41358,10.);
#11740=VECTOR('',#41363,10.);
#11741=VECTOR('',#41368,10.);
#11742=VECTOR('',#41369,10.);
#11743=VECTOR('',#41370,10.);
#11744=VECTOR('',#41383,10.);
#11745=VECTOR('',#41384,10.);
#11746=VECTOR('',#41385,10.);
#11747=VECTOR('',#41386,10.);
#11748=VECTOR('',#41391,10.);
#11749=VECTOR('',#41396,10.);
#11750=VECTOR('',#41397,10.);
#11751=VECTOR('',#41398,10.);
#11752=VECTOR('',#41403,10.);
#11753=VECTOR('',#41408,10.);
#11754=VECTOR('',#41409,10.);
#11755=VECTOR('',#41410,10.);
#11756=VECTOR('',#41411,10.);
#11757=VECTOR('',#41416,10.);
#11758=VECTOR('',#41421,10.);
#11759=VECTOR('',#41422,10.);
#11760=VECTOR('',#41423,10.);
#11761=VECTOR('',#41428,10.);
#11762=VECTOR('',#41433,10.);
#11763=VECTOR('',#41434,10.);
#11764=VECTOR('',#41435,10.);
#11765=VECTOR('',#41442,10.);
#11766=VECTOR('',#41445,10.);
#11767=VECTOR('',#41446,10.);
#11768=VECTOR('',#41447,10.);
#11769=VECTOR('',#41456,10.);
#11770=VECTOR('',#41457,10.);
#11771=VECTOR('',#41458,10.);
#11772=VECTOR('',#41463,10.);
#11773=VECTOR('',#41468,10.);
#11774=VECTOR('',#41469,10.);
#11775=VECTOR('',#41470,10.);
#11776=VECTOR('',#41485,10.);
#11777=VECTOR('',#41488,10.);
#11778=VECTOR('',#41491,10.);
#11779=VECTOR('',#41494,10.);
#11780=VECTOR('',#41495,10.);
#11781=VECTOR('',#41498,10.);
#11782=VECTOR('',#41501,10.);
#11783=VECTOR('',#41504,10.);
#11784=VECTOR('',#41509,10.);
#11785=VECTOR('',#41510,10.);
#11786=VECTOR('',#41511,10.);
#11787=VECTOR('',#41514,10.);
#11788=VECTOR('',#41519,10.);
#11789=VECTOR('',#41520,10.);
#11790=VECTOR('',#41523,10.);
#11791=VECTOR('',#41528,10.);
#11792=VECTOR('',#41531,10.);
#11793=VECTOR('',#41534,10.);
#11794=VECTOR('',#41537,10.);
#11795=VECTOR('',#41540,10.);
#11796=VECTOR('',#41541,10.);
#11797=VECTOR('',#41544,10.);
#11798=VECTOR('',#41547,10.);
#11799=VECTOR('',#41550,10.);
#11800=VECTOR('',#41551,10.);
#11801=VECTOR('',#41554,10.);
#11802=VECTOR('',#41559,10.);
#11803=VECTOR('',#41562,10.);
#11804=VECTOR('',#41565,10.);
#11805=VECTOR('',#41568,10.);
#11806=VECTOR('',#41575,10.);
#11807=VECTOR('',#41578,10.);
#11808=VECTOR('',#41585,10.);
#11809=VECTOR('',#41588,10.);
#11810=VECTOR('',#41591,10.);
#11811=VECTOR('',#41594,10.);
#11812=VECTOR('',#41595,10.);
#11813=VECTOR('',#41598,10.);
#11814=VECTOR('',#41601,10.);
#11815=VECTOR('',#41604,10.);
#11816=VECTOR('',#41609,10.);
#11817=VECTOR('',#41610,10.);
#11818=VECTOR('',#41611,10.);
#11819=VECTOR('',#41614,10.);
#11820=VECTOR('',#41619,10.);
#11821=VECTOR('',#41620,10.);
#11822=VECTOR('',#41623,10.);
#11823=VECTOR('',#41628,10.);
#11824=VECTOR('',#41631,10.);
#11825=VECTOR('',#41634,10.);
#11826=VECTOR('',#41635,10.);
#11827=VECTOR('',#41638,10.);
#11828=VECTOR('',#41643,10.);
#11829=VECTOR('',#41644,10.);
#11830=VECTOR('',#41649,10.);
#11831=VECTOR('',#41652,10.);
#11832=VECTOR('',#41653,10.);
#11833=VECTOR('',#41656,10.);
#11834=VECTOR('',#41661,10.);
#11835=VECTOR('',#41664,10.);
#11836=VECTOR('',#41667,10.);
#11837=VECTOR('',#41670,10.);
#11838=VECTOR('',#41675,10.);
#11839=VECTOR('',#41678,10.);
#11840=VECTOR('',#41683,10.);
#11841=VECTOR('',#41686,10.);
#11842=VECTOR('',#41689,10.);
#11843=VECTOR('',#41692,10.);
#11844=VECTOR('',#41695,10.);
#11845=VECTOR('',#41698,10.);
#11846=VECTOR('',#41701,10.);
#11847=VECTOR('',#41704,10.);
#11848=VECTOR('',#41709,10.);
#11849=VECTOR('',#41710,10.);
#11850=VECTOR('',#41711,10.);
#11851=VECTOR('',#41714,10.);
#11852=VECTOR('',#41719,10.);
#11853=VECTOR('',#41720,10.);
#11854=VECTOR('',#41723,10.);
#11855=VECTOR('',#41728,10.);
#11856=VECTOR('',#41729,10.);
#11857=VECTOR('',#41730,10.);
#11858=VECTOR('',#41733,10.);
#11859=VECTOR('',#41738,10.);
#11860=VECTOR('',#41739,10.);
#11861=VECTOR('',#41742,10.);
#11862=VECTOR('',#41747,10.);
#11863=VECTOR('',#41750,10.);
#11864=VECTOR('',#41753,10.);
#11865=VECTOR('',#41756,10.);
#11866=VECTOR('',#41761,10.);
#11867=VECTOR('',#41764,10.);
#11868=VECTOR('',#41767,10.);
#11869=VECTOR('',#41770,10.);
#11870=VECTOR('',#41775,10.);
#11871=VECTOR('',#41778,10.);
#11872=VECTOR('',#41783,10.);
#11873=VECTOR('',#41786,10.);
#11874=VECTOR('',#41789,10.);
#11875=VECTOR('',#41792,10.);
#11876=VECTOR('',#41795,10.);
#11877=VECTOR('',#41798,10.);
#11878=VECTOR('',#41801,10.);
#11879=VECTOR('',#41804,10.);
#11880=VECTOR('',#41809,10.);
#11881=VECTOR('',#41810,10.);
#11882=VECTOR('',#41811,10.);
#11883=VECTOR('',#41814,10.);
#11884=VECTOR('',#41819,10.);
#11885=VECTOR('',#41820,10.);
#11886=VECTOR('',#41823,10.);
#11887=VECTOR('',#41828,10.);
#11888=VECTOR('',#41829,10.);
#11889=VECTOR('',#41830,10.);
#11890=VECTOR('',#41833,10.);
#11891=VECTOR('',#41838,10.);
#11892=VECTOR('',#41839,10.);
#11893=VECTOR('',#41842,10.);
#11894=VECTOR('',#41847,10.);
#11895=VECTOR('',#41850,10.);
#11896=VECTOR('',#41853,10.);
#11897=VECTOR('',#41856,10.);
#11898=VECTOR('',#41861,10.);
#11899=VECTOR('',#41864,10.);
#11900=VECTOR('',#41867,10.);
#11901=VECTOR('',#41870,10.);
#11902=VECTOR('',#41875,10.);
#11903=VECTOR('',#41878,10.);
#11904=VECTOR('',#41883,10.);
#11905=VECTOR('',#41884,10.);
#11906=VECTOR('',#41885,10.);
#11907=VECTOR('',#41886,10.);
#11908=VECTOR('',#41891,10.);
#11909=VECTOR('',#41896,10.);
#11910=VECTOR('',#41897,10.);
#11911=VECTOR('',#41898,10.);
#11912=VECTOR('',#41903,10.);
#11913=VECTOR('',#41908,10.);
#11914=VECTOR('',#41909,10.);
#11915=VECTOR('',#41910,10.);
#11916=VECTOR('',#41911,10.);
#11917=VECTOR('',#41916,10.);
#11918=VECTOR('',#41921,10.);
#11919=VECTOR('',#41922,10.);
#11920=VECTOR('',#41923,10.);
#11921=VECTOR('',#41928,10.);
#11922=VECTOR('',#41933,10.);
#11923=VECTOR('',#41934,10.);
#11924=VECTOR('',#41935,10.);
#11925=VECTOR('',#41942,10.);
#11926=VECTOR('',#41945,10.);
#11927=VECTOR('',#41946,10.);
#11928=VECTOR('',#41947,10.);
#11929=VECTOR('',#41956,10.);
#11930=VECTOR('',#41957,10.);
#11931=VECTOR('',#41958,10.);
#11932=VECTOR('',#41963,10.);
#11933=VECTOR('',#41968,10.);
#11934=VECTOR('',#41969,10.);
#11935=VECTOR('',#41970,10.);
#11936=VECTOR('',#41983,10.);
#11937=VECTOR('',#41984,10.);
#11938=VECTOR('',#41985,10.);
#11939=VECTOR('',#41986,10.);
#11940=VECTOR('',#41991,10.);
#11941=VECTOR('',#41996,10.);
#11942=VECTOR('',#41997,10.);
#11943=VECTOR('',#41998,10.);
#11944=VECTOR('',#42003,10.);
#11945=VECTOR('',#42008,10.);
#11946=VECTOR('',#42009,10.);
#11947=VECTOR('',#42010,10.);
#11948=VECTOR('',#42011,10.);
#11949=VECTOR('',#42016,10.);
#11950=VECTOR('',#42021,10.);
#11951=VECTOR('',#42022,10.);
#11952=VECTOR('',#42023,10.);
#11953=VECTOR('',#42028,10.);
#11954=VECTOR('',#42033,10.);
#11955=VECTOR('',#42034,10.);
#11956=VECTOR('',#42035,10.);
#11957=VECTOR('',#42042,10.);
#11958=VECTOR('',#42045,10.);
#11959=VECTOR('',#42046,10.);
#11960=VECTOR('',#42047,10.);
#11961=VECTOR('',#42056,10.);
#11962=VECTOR('',#42057,10.);
#11963=VECTOR('',#42058,10.);
#11964=VECTOR('',#42063,10.);
#11965=VECTOR('',#42068,10.);
#11966=VECTOR('',#42069,10.);
#11967=VECTOR('',#42070,10.);
#11968=VECTOR('',#42083,10.);
#11969=VECTOR('',#42084,10.);
#11970=VECTOR('',#42085,10.);
#11971=VECTOR('',#42086,10.);
#11972=VECTOR('',#42091,10.);
#11973=VECTOR('',#42096,10.);
#11974=VECTOR('',#42097,10.);
#11975=VECTOR('',#42098,10.);
#11976=VECTOR('',#42103,10.);
#11977=VECTOR('',#42108,10.);
#11978=VECTOR('',#42109,10.);
#11979=VECTOR('',#42110,10.);
#11980=VECTOR('',#42111,10.);
#11981=VECTOR('',#42116,10.);
#11982=VECTOR('',#42121,10.);
#11983=VECTOR('',#42122,10.);
#11984=VECTOR('',#42123,10.);
#11985=VECTOR('',#42128,10.);
#11986=VECTOR('',#42133,10.);
#11987=VECTOR('',#42134,10.);
#11988=VECTOR('',#42135,10.);
#11989=VECTOR('',#42142,10.);
#11990=VECTOR('',#42145,10.);
#11991=VECTOR('',#42146,10.);
#11992=VECTOR('',#42147,10.);
#11993=VECTOR('',#42156,10.);
#11994=VECTOR('',#42157,10.);
#11995=VECTOR('',#42158,10.);
#11996=VECTOR('',#42163,10.);
#11997=VECTOR('',#42168,10.);
#11998=VECTOR('',#42169,10.);
#11999=VECTOR('',#42170,10.);
#12000=VECTOR('',#42185,10.);
#12001=VECTOR('',#42188,10.);
#12002=VECTOR('',#42191,10.);
#12003=VECTOR('',#42192,10.);
#12004=VECTOR('',#42193,10.);
#12005=VECTOR('',#42198,10.);
#12006=VECTOR('',#42203,10.);
#12007=VECTOR('',#42204,10.);
#12008=VECTOR('',#42205,10.);
#12009=VECTOR('',#42210,10.);
#12010=VECTOR('',#42215,10.);
#12011=VECTOR('',#42216,10.);
#12012=VECTOR('',#42217,10.);
#12013=VECTOR('',#42222,10.);
#12014=VECTOR('',#42227,10.);
#12015=VECTOR('',#42228,10.);
#12016=VECTOR('',#42233,10.);
#12017=VECTOR('',#42236,10.);
#12018=VECTOR('',#42239,10.);
#12019=VECTOR('',#42240,10.);
#12020=VECTOR('',#42241,10.);
#12021=VECTOR('',#42248,10.);
#12022=VECTOR('',#42251,10.);
#12023=VECTOR('',#42252,10.);
#12024=VECTOR('',#42253,10.);
#12025=VECTOR('',#42260,10.);
#12026=VECTOR('',#42263,10.);
#12027=VECTOR('',#42264,10.);
#12028=VECTOR('',#42265,10.);
#12029=VECTOR('',#42272,10.);
#12030=VECTOR('',#42275,10.);
#12031=VECTOR('',#42276,10.);
#12032=VECTOR('',#42285,10.);
#12033=VECTOR('',#42288,10.);
#12034=VECTOR('',#42291,10.);
#12035=VECTOR('',#42292,10.);
#12036=VECTOR('',#42293,10.);
#12037=VECTOR('',#42298,10.);
#12038=VECTOR('',#42303,10.);
#12039=VECTOR('',#42304,10.);
#12040=VECTOR('',#42305,10.);
#12041=VECTOR('',#42310,10.);
#12042=VECTOR('',#42315,10.);
#12043=VECTOR('',#42316,10.);
#12044=VECTOR('',#42317,10.);
#12045=VECTOR('',#42322,10.);
#12046=VECTOR('',#42327,10.);
#12047=VECTOR('',#42328,10.);
#12048=VECTOR('',#42333,10.);
#12049=VECTOR('',#42336,10.);
#12050=VECTOR('',#42339,10.);
#12051=VECTOR('',#42340,10.);
#12052=VECTOR('',#42341,10.);
#12053=VECTOR('',#42348,10.);
#12054=VECTOR('',#42351,10.);
#12055=VECTOR('',#42352,10.);
#12056=VECTOR('',#42353,10.);
#12057=VECTOR('',#42360,10.);
#12058=VECTOR('',#42363,10.);
#12059=VECTOR('',#42364,10.);
#12060=VECTOR('',#42365,10.);
#12061=VECTOR('',#42372,10.);
#12062=VECTOR('',#42375,10.);
#12063=VECTOR('',#42376,10.);
#12064=VECTOR('',#42385,10.);
#12065=VECTOR('',#42388,10.);
#12066=VECTOR('',#42391,10.);
#12067=VECTOR('',#42392,10.);
#12068=VECTOR('',#42393,10.);
#12069=VECTOR('',#42398,10.);
#12070=VECTOR('',#42403,10.);
#12071=VECTOR('',#42404,10.);
#12072=VECTOR('',#42405,10.);
#12073=VECTOR('',#42410,10.);
#12074=VECTOR('',#42415,10.);
#12075=VECTOR('',#42416,10.);
#12076=VECTOR('',#42417,10.);
#12077=VECTOR('',#42422,10.);
#12078=VECTOR('',#42427,10.);
#12079=VECTOR('',#42428,10.);
#12080=VECTOR('',#42433,10.);
#12081=VECTOR('',#42436,10.);
#12082=VECTOR('',#42439,10.);
#12083=VECTOR('',#42440,10.);
#12084=VECTOR('',#42441,10.);
#12085=VECTOR('',#42448,10.);
#12086=VECTOR('',#42451,10.);
#12087=VECTOR('',#42452,10.);
#12088=VECTOR('',#42453,10.);
#12089=VECTOR('',#42460,10.);
#12090=VECTOR('',#42463,10.);
#12091=VECTOR('',#42464,10.);
#12092=VECTOR('',#42465,10.);
#12093=VECTOR('',#42472,10.);
#12094=VECTOR('',#42475,10.);
#12095=VECTOR('',#42476,10.);
#12096=VECTOR('',#42485,10.);
#12097=VECTOR('',#42488,10.);
#12098=VECTOR('',#42491,10.);
#12099=VECTOR('',#42492,10.);
#12100=VECTOR('',#42493,10.);
#12101=VECTOR('',#42498,10.);
#12102=VECTOR('',#42503,10.);
#12103=VECTOR('',#42504,10.);
#12104=VECTOR('',#42505,10.);
#12105=VECTOR('',#42510,10.);
#12106=VECTOR('',#42515,10.);
#12107=VECTOR('',#42516,10.);
#12108=VECTOR('',#42517,10.);
#12109=VECTOR('',#42522,10.);
#12110=VECTOR('',#42527,10.);
#12111=VECTOR('',#42528,10.);
#12112=VECTOR('',#42533,10.);
#12113=VECTOR('',#42536,10.);
#12114=VECTOR('',#42539,10.);
#12115=VECTOR('',#42540,10.);
#12116=VECTOR('',#42541,10.);
#12117=VECTOR('',#42548,10.);
#12118=VECTOR('',#42551,10.);
#12119=VECTOR('',#42552,10.);
#12120=VECTOR('',#42553,10.);
#12121=VECTOR('',#42560,10.);
#12122=VECTOR('',#42563,10.);
#12123=VECTOR('',#42564,10.);
#12124=VECTOR('',#42565,10.);
#12125=VECTOR('',#42572,10.);
#12126=VECTOR('',#42575,10.);
#12127=VECTOR('',#42576,10.);
#14322=VERTEX_POINT('',#53783);
#14323=VERTEX_POINT('',#53784);
#14324=VERTEX_POINT('',#53786);
#14325=VERTEX_POINT('',#53788);
#14326=VERTEX_POINT('',#53792);
#14327=VERTEX_POINT('',#53794);
#14328=VERTEX_POINT('',#53798);
#14329=VERTEX_POINT('',#53800);
#14330=VERTEX_POINT('',#53804);
#14331=VERTEX_POINT('',#53806);
#14332=VERTEX_POINT('',#53810);
#14333=VERTEX_POINT('',#53811);
#14334=VERTEX_POINT('',#53813);
#14335=VERTEX_POINT('',#53815);
#14336=VERTEX_POINT('',#53819);
#14337=VERTEX_POINT('',#53821);
#14338=VERTEX_POINT('',#53825);
#14339=VERTEX_POINT('',#53827);
#14340=VERTEX_POINT('',#53831);
#14341=VERTEX_POINT('',#53833);
#14342=VERTEX_POINT('',#53837);
#14343=VERTEX_POINT('',#53839);
#14344=VERTEX_POINT('',#53843);
#14345=VERTEX_POINT('',#53845);
#14346=VERTEX_POINT('',#53849);
#14347=VERTEX_POINT('',#53851);
#14348=VERTEX_POINT('',#53858);
#14349=VERTEX_POINT('',#53860);
#14350=VERTEX_POINT('',#53864);
#14351=VERTEX_POINT('',#53866);
#14352=VERTEX_POINT('',#53870);
#14353=VERTEX_POINT('',#53872);
#14354=VERTEX_POINT('',#53881);
#14355=VERTEX_POINT('',#53882);
#14356=VERTEX_POINT('',#53884);
#14357=VERTEX_POINT('',#53886);
#14358=VERTEX_POINT('',#53890);
#14359=VERTEX_POINT('',#53892);
#14360=VERTEX_POINT('',#53896);
#14361=VERTEX_POINT('',#53898);
#14362=VERTEX_POINT('',#53902);
#14363=VERTEX_POINT('',#53904);
#14364=VERTEX_POINT('',#53908);
#14365=VERTEX_POINT('',#53909);
#14366=VERTEX_POINT('',#53911);
#14367=VERTEX_POINT('',#53913);
#14368=VERTEX_POINT('',#53917);
#14369=VERTEX_POINT('',#53919);
#14370=VERTEX_POINT('',#53923);
#14371=VERTEX_POINT('',#53925);
#14372=VERTEX_POINT('',#53929);
#14373=VERTEX_POINT('',#53931);
#14374=VERTEX_POINT('',#53935);
#14375=VERTEX_POINT('',#53937);
#14376=VERTEX_POINT('',#53941);
#14377=VERTEX_POINT('',#53943);
#14378=VERTEX_POINT('',#53947);
#14379=VERTEX_POINT('',#53949);
#14380=VERTEX_POINT('',#53956);
#14381=VERTEX_POINT('',#53958);
#14382=VERTEX_POINT('',#53962);
#14383=VERTEX_POINT('',#53964);
#14384=VERTEX_POINT('',#53968);
#14385=VERTEX_POINT('',#53970);
#14386=VERTEX_POINT('',#53979);
#14387=VERTEX_POINT('',#53980);
#14388=VERTEX_POINT('',#53982);
#14389=VERTEX_POINT('',#53984);
#14390=VERTEX_POINT('',#53988);
#14391=VERTEX_POINT('',#53990);
#14392=VERTEX_POINT('',#53994);
#14393=VERTEX_POINT('',#53996);
#14394=VERTEX_POINT('',#54000);
#14395=VERTEX_POINT('',#54002);
#14396=VERTEX_POINT('',#54006);
#14397=VERTEX_POINT('',#54007);
#14398=VERTEX_POINT('',#54009);
#14399=VERTEX_POINT('',#54011);
#14400=VERTEX_POINT('',#54015);
#14401=VERTEX_POINT('',#54017);
#14402=VERTEX_POINT('',#54021);
#14403=VERTEX_POINT('',#54023);
#14404=VERTEX_POINT('',#54027);
#14405=VERTEX_POINT('',#54029);
#14406=VERTEX_POINT('',#54033);
#14407=VERTEX_POINT('',#54035);
#14408=VERTEX_POINT('',#54039);
#14409=VERTEX_POINT('',#54041);
#14410=VERTEX_POINT('',#54045);
#14411=VERTEX_POINT('',#54047);
#14412=VERTEX_POINT('',#54054);
#14413=VERTEX_POINT('',#54056);
#14414=VERTEX_POINT('',#54060);
#14415=VERTEX_POINT('',#54062);
#14416=VERTEX_POINT('',#54066);
#14417=VERTEX_POINT('',#54068);
#14418=VERTEX_POINT('',#54077);
#14419=VERTEX_POINT('',#54078);
#14420=VERTEX_POINT('',#54080);
#14421=VERTEX_POINT('',#54082);
#14422=VERTEX_POINT('',#54086);
#14423=VERTEX_POINT('',#54088);
#14424=VERTEX_POINT('',#54092);
#14425=VERTEX_POINT('',#54094);
#14426=VERTEX_POINT('',#54098);
#14427=VERTEX_POINT('',#54100);
#14428=VERTEX_POINT('',#54104);
#14429=VERTEX_POINT('',#54105);
#14430=VERTEX_POINT('',#54107);
#14431=VERTEX_POINT('',#54109);
#14432=VERTEX_POINT('',#54113);
#14433=VERTEX_POINT('',#54115);
#14434=VERTEX_POINT('',#54119);
#14435=VERTEX_POINT('',#54121);
#14436=VERTEX_POINT('',#54125);
#14437=VERTEX_POINT('',#54127);
#14438=VERTEX_POINT('',#54131);
#14439=VERTEX_POINT('',#54133);
#14440=VERTEX_POINT('',#54137);
#14441=VERTEX_POINT('',#54139);
#14442=VERTEX_POINT('',#54143);
#14443=VERTEX_POINT('',#54145);
#14444=VERTEX_POINT('',#54152);
#14445=VERTEX_POINT('',#54154);
#14446=VERTEX_POINT('',#54158);
#14447=VERTEX_POINT('',#54160);
#14448=VERTEX_POINT('',#54164);
#14449=VERTEX_POINT('',#54166);
#14450=VERTEX_POINT('',#54175);
#14451=VERTEX_POINT('',#54176);
#14452=VERTEX_POINT('',#54178);
#14453=VERTEX_POINT('',#54180);
#14454=VERTEX_POINT('',#54182);
#14455=VERTEX_POINT('',#54184);
#14456=VERTEX_POINT('',#54186);
#14457=VERTEX_POINT('',#54188);
#14458=VERTEX_POINT('',#54191);
#14459=VERTEX_POINT('',#54192);
#14460=VERTEX_POINT('',#54194);
#14461=VERTEX_POINT('',#54196);
#14462=VERTEX_POINT('',#54198);
#14463=VERTEX_POINT('',#54200);
#14464=VERTEX_POINT('',#54202);
#14465=VERTEX_POINT('',#54204);
#14466=VERTEX_POINT('',#54208);
#14467=VERTEX_POINT('',#54210);
#14468=VERTEX_POINT('',#54214);
#14469=VERTEX_POINT('',#54218);
#14470=VERTEX_POINT('',#54222);
#14471=VERTEX_POINT('',#54226);
#14472=VERTEX_POINT('',#54228);
#14473=VERTEX_POINT('',#54232);
#14474=VERTEX_POINT('',#54234);
#14475=VERTEX_POINT('',#54238);
#14476=VERTEX_POINT('',#54243);
#14477=VERTEX_POINT('',#54245);
#14478=VERTEX_POINT('',#54247);
#14479=VERTEX_POINT('',#54250);
#14480=VERTEX_POINT('',#54252);
#14481=VERTEX_POINT('',#54254);
#14482=VERTEX_POINT('',#54273);
#14483=VERTEX_POINT('',#54274);
#14484=VERTEX_POINT('',#54276);
#14485=VERTEX_POINT('',#54278);
#14486=VERTEX_POINT('',#54280);
#14487=VERTEX_POINT('',#54282);
#14488=VERTEX_POINT('',#54284);
#14489=VERTEX_POINT('',#54286);
#14490=VERTEX_POINT('',#54289);
#14491=VERTEX_POINT('',#54290);
#14492=VERTEX_POINT('',#54292);
#14493=VERTEX_POINT('',#54294);
#14494=VERTEX_POINT('',#54296);
#14495=VERTEX_POINT('',#54298);
#14496=VERTEX_POINT('',#54300);
#14497=VERTEX_POINT('',#54302);
#14498=VERTEX_POINT('',#54306);
#14499=VERTEX_POINT('',#54308);
#14500=VERTEX_POINT('',#54312);
#14501=VERTEX_POINT('',#54316);
#14502=VERTEX_POINT('',#54320);
#14503=VERTEX_POINT('',#54324);
#14504=VERTEX_POINT('',#54326);
#14505=VERTEX_POINT('',#54330);
#14506=VERTEX_POINT('',#54334);
#14507=VERTEX_POINT('',#54338);
#14508=VERTEX_POINT('',#54342);
#14509=VERTEX_POINT('',#54344);
#14510=VERTEX_POINT('',#54346);
#14511=VERTEX_POINT('',#54349);
#14512=VERTEX_POINT('',#54351);
#14513=VERTEX_POINT('',#54353);
#14514=VERTEX_POINT('',#54371);
#14515=VERTEX_POINT('',#54372);
#14516=VERTEX_POINT('',#54374);
#14517=VERTEX_POINT('',#54376);
#14518=VERTEX_POINT('',#54378);
#14519=VERTEX_POINT('',#54380);
#14520=VERTEX_POINT('',#54382);
#14521=VERTEX_POINT('',#54384);
#14522=VERTEX_POINT('',#54387);
#14523=VERTEX_POINT('',#54388);
#14524=VERTEX_POINT('',#54390);
#14525=VERTEX_POINT('',#54392);
#14526=VERTEX_POINT('',#54394);
#14527=VERTEX_POINT('',#54396);
#14528=VERTEX_POINT('',#54398);
#14529=VERTEX_POINT('',#54400);
#14530=VERTEX_POINT('',#54404);
#14531=VERTEX_POINT('',#54406);
#14532=VERTEX_POINT('',#54410);
#14533=VERTEX_POINT('',#54414);
#14534=VERTEX_POINT('',#54418);
#14535=VERTEX_POINT('',#54422);
#14536=VERTEX_POINT('',#54424);
#14537=VERTEX_POINT('',#54428);
#14538=VERTEX_POINT('',#54432);
#14539=VERTEX_POINT('',#54436);
#14540=VERTEX_POINT('',#54440);
#14541=VERTEX_POINT('',#54442);
#14542=VERTEX_POINT('',#54444);
#14543=VERTEX_POINT('',#54447);
#14544=VERTEX_POINT('',#54449);
#14545=VERTEX_POINT('',#54451);
#14546=VERTEX_POINT('',#54469);
#14547=VERTEX_POINT('',#54470);
#14548=VERTEX_POINT('',#54472);
#14549=VERTEX_POINT('',#54474);
#14550=VERTEX_POINT('',#54476);
#14551=VERTEX_POINT('',#54478);
#14552=VERTEX_POINT('',#54480);
#14553=VERTEX_POINT('',#54482);
#14554=VERTEX_POINT('',#54485);
#14555=VERTEX_POINT('',#54486);
#14556=VERTEX_POINT('',#54488);
#14557=VERTEX_POINT('',#54490);
#14558=VERTEX_POINT('',#54492);
#14559=VERTEX_POINT('',#54494);
#14560=VERTEX_POINT('',#54496);
#14561=VERTEX_POINT('',#54498);
#14562=VERTEX_POINT('',#54502);
#14563=VERTEX_POINT('',#54504);
#14564=VERTEX_POINT('',#54508);
#14565=VERTEX_POINT('',#54512);
#14566=VERTEX_POINT('',#54516);
#14567=VERTEX_POINT('',#54520);
#14568=VERTEX_POINT('',#54522);
#14569=VERTEX_POINT('',#54526);
#14570=VERTEX_POINT('',#54530);
#14571=VERTEX_POINT('',#54534);
#14572=VERTEX_POINT('',#54538);
#14573=VERTEX_POINT('',#54540);
#14574=VERTEX_POINT('',#54542);
#14575=VERTEX_POINT('',#54545);
#14576=VERTEX_POINT('',#54547);
#14577=VERTEX_POINT('',#54549);
#14578=VERTEX_POINT('',#54567);
#14579=VERTEX_POINT('',#54568);
#14580=VERTEX_POINT('',#54570);
#14581=VERTEX_POINT('',#54572);
#14582=VERTEX_POINT('',#54576);
#14583=VERTEX_POINT('',#54578);
#14584=VERTEX_POINT('',#54582);
#14585=VERTEX_POINT('',#54584);
#14586=VERTEX_POINT('',#54588);
#14587=VERTEX_POINT('',#54590);
#14588=VERTEX_POINT('',#54594);
#14589=VERTEX_POINT('',#54595);
#14590=VERTEX_POINT('',#54597);
#14591=VERTEX_POINT('',#54599);
#14592=VERTEX_POINT('',#54603);
#14593=VERTEX_POINT('',#54605);
#14594=VERTEX_POINT('',#54609);
#14595=VERTEX_POINT('',#54611);
#14596=VERTEX_POINT('',#54615);
#14597=VERTEX_POINT('',#54617);
#14598=VERTEX_POINT('',#54621);
#14599=VERTEX_POINT('',#54623);
#14600=VERTEX_POINT('',#54627);
#14601=VERTEX_POINT('',#54629);
#14602=VERTEX_POINT('',#54633);
#14603=VERTEX_POINT('',#54635);
#14604=VERTEX_POINT('',#54642);
#14605=VERTEX_POINT('',#54644);
#14606=VERTEX_POINT('',#54648);
#14607=VERTEX_POINT('',#54650);
#14608=VERTEX_POINT('',#54654);
#14609=VERTEX_POINT('',#54656);
#14610=VERTEX_POINT('',#54665);
#14611=VERTEX_POINT('',#54666);
#14612=VERTEX_POINT('',#54668);
#14613=VERTEX_POINT('',#54670);
#14614=VERTEX_POINT('',#54674);
#14615=VERTEX_POINT('',#54676);
#14616=VERTEX_POINT('',#54680);
#14617=VERTEX_POINT('',#54682);
#14618=VERTEX_POINT('',#54686);
#14619=VERTEX_POINT('',#54688);
#14620=VERTEX_POINT('',#54692);
#14621=VERTEX_POINT('',#54693);
#14622=VERTEX_POINT('',#54695);
#14623=VERTEX_POINT('',#54697);
#14624=VERTEX_POINT('',#54701);
#14625=VERTEX_POINT('',#54703);
#14626=VERTEX_POINT('',#54707);
#14627=VERTEX_POINT('',#54709);
#14628=VERTEX_POINT('',#54713);
#14629=VERTEX_POINT('',#54715);
#14630=VERTEX_POINT('',#54719);
#14631=VERTEX_POINT('',#54721);
#14632=VERTEX_POINT('',#54725);
#14633=VERTEX_POINT('',#54727);
#14634=VERTEX_POINT('',#54731);
#14635=VERTEX_POINT('',#54733);
#14636=VERTEX_POINT('',#54740);
#14637=VERTEX_POINT('',#54742);
#14638=VERTEX_POINT('',#54746);
#14639=VERTEX_POINT('',#54748);
#14640=VERTEX_POINT('',#54752);
#14641=VERTEX_POINT('',#54754);
#14642=VERTEX_POINT('',#54763);
#14643=VERTEX_POINT('',#54764);
#14644=VERTEX_POINT('',#54766);
#14645=VERTEX_POINT('',#54768);
#14646=VERTEX_POINT('',#54772);
#14647=VERTEX_POINT('',#54774);
#14648=VERTEX_POINT('',#54778);
#14649=VERTEX_POINT('',#54780);
#14650=VERTEX_POINT('',#54784);
#14651=VERTEX_POINT('',#54786);
#14652=VERTEX_POINT('',#54790);
#14653=VERTEX_POINT('',#54791);
#14654=VERTEX_POINT('',#54793);
#14655=VERTEX_POINT('',#54795);
#14656=VERTEX_POINT('',#54799);
#14657=VERTEX_POINT('',#54801);
#14658=VERTEX_POINT('',#54805);
#14659=VERTEX_POINT('',#54807);
#14660=VERTEX_POINT('',#54811);
#14661=VERTEX_POINT('',#54813);
#14662=VERTEX_POINT('',#54817);
#14663=VERTEX_POINT('',#54819);
#14664=VERTEX_POINT('',#54823);
#14665=VERTEX_POINT('',#54825);
#14666=VERTEX_POINT('',#54829);
#14667=VERTEX_POINT('',#54831);
#14668=VERTEX_POINT('',#54838);
#14669=VERTEX_POINT('',#54840);
#14670=VERTEX_POINT('',#54844);
#14671=VERTEX_POINT('',#54846);
#14672=VERTEX_POINT('',#54850);
#14673=VERTEX_POINT('',#54852);
#14674=VERTEX_POINT('',#54861);
#14675=VERTEX_POINT('',#54862);
#14676=VERTEX_POINT('',#54864);
#14677=VERTEX_POINT('',#54866);
#14678=VERTEX_POINT('',#54870);
#14679=VERTEX_POINT('',#54872);
#14680=VERTEX_POINT('',#54876);
#14681=VERTEX_POINT('',#54878);
#14682=VERTEX_POINT('',#54882);
#14683=VERTEX_POINT('',#54884);
#14684=VERTEX_POINT('',#54888);
#14685=VERTEX_POINT('',#54890);
#14686=VERTEX_POINT('',#54894);
#14687=VERTEX_POINT('',#54896);
#14688=VERTEX_POINT('',#54900);
#14689=VERTEX_POINT('',#54902);
#14690=VERTEX_POINT('',#54909);
#14691=VERTEX_POINT('',#54910);
#14692=VERTEX_POINT('',#54912);
#14693=VERTEX_POINT('',#54914);
#14694=VERTEX_POINT('',#54918);
#14695=VERTEX_POINT('',#54920);
#14696=VERTEX_POINT('',#54924);
#14697=VERTEX_POINT('',#54926);
#14698=VERTEX_POINT('',#54930);
#14699=VERTEX_POINT('',#54932);
#14700=VERTEX_POINT('',#54936);
#14701=VERTEX_POINT('',#54938);
#14702=VERTEX_POINT('',#54942);
#14703=VERTEX_POINT('',#54944);
#14704=VERTEX_POINT('',#54948);
#14705=VERTEX_POINT('',#54950);
#14706=VERTEX_POINT('',#54959);
#14707=VERTEX_POINT('',#54960);
#14708=VERTEX_POINT('',#54962);
#14709=VERTEX_POINT('',#54964);
#14710=VERTEX_POINT('',#54968);
#14711=VERTEX_POINT('',#54970);
#14712=VERTEX_POINT('',#54974);
#14713=VERTEX_POINT('',#54976);
#14714=VERTEX_POINT('',#54980);
#14715=VERTEX_POINT('',#54982);
#14716=VERTEX_POINT('',#54986);
#14717=VERTEX_POINT('',#54988);
#14718=VERTEX_POINT('',#54992);
#14719=VERTEX_POINT('',#54994);
#14720=VERTEX_POINT('',#54998);
#14721=VERTEX_POINT('',#55000);
#14722=VERTEX_POINT('',#55007);
#14723=VERTEX_POINT('',#55008);
#14724=VERTEX_POINT('',#55010);
#14725=VERTEX_POINT('',#55012);
#14726=VERTEX_POINT('',#55016);
#14727=VERTEX_POINT('',#55018);
#14728=VERTEX_POINT('',#55022);
#14729=VERTEX_POINT('',#55024);
#14730=VERTEX_POINT('',#55028);
#14731=VERTEX_POINT('',#55030);
#14732=VERTEX_POINT('',#55034);
#14733=VERTEX_POINT('',#55036);
#14734=VERTEX_POINT('',#55040);
#14735=VERTEX_POINT('',#55042);
#14736=VERTEX_POINT('',#55046);
#14737=VERTEX_POINT('',#55048);
#14738=VERTEX_POINT('',#55057);
#14739=VERTEX_POINT('',#55058);
#14740=VERTEX_POINT('',#55060);
#14741=VERTEX_POINT('',#55062);
#14742=VERTEX_POINT('',#55066);
#14743=VERTEX_POINT('',#55068);
#14744=VERTEX_POINT('',#55072);
#14745=VERTEX_POINT('',#55074);
#14746=VERTEX_POINT('',#55078);
#14747=VERTEX_POINT('',#55080);
#14748=VERTEX_POINT('',#55084);
#14749=VERTEX_POINT('',#55086);
#14750=VERTEX_POINT('',#55090);
#14751=VERTEX_POINT('',#55092);
#14752=VERTEX_POINT('',#55096);
#14753=VERTEX_POINT('',#55098);
#14754=VERTEX_POINT('',#55105);
#14755=VERTEX_POINT('',#55106);
#14756=VERTEX_POINT('',#55108);
#14757=VERTEX_POINT('',#55110);
#14758=VERTEX_POINT('',#55114);
#14759=VERTEX_POINT('',#55116);
#14760=VERTEX_POINT('',#55120);
#14761=VERTEX_POINT('',#55122);
#14762=VERTEX_POINT('',#55126);
#14763=VERTEX_POINT('',#55128);
#14764=VERTEX_POINT('',#55132);
#14765=VERTEX_POINT('',#55134);
#14766=VERTEX_POINT('',#55138);
#14767=VERTEX_POINT('',#55140);
#14768=VERTEX_POINT('',#55144);
#14769=VERTEX_POINT('',#55146);
#14770=VERTEX_POINT('',#55155);
#14771=VERTEX_POINT('',#55156);
#14772=VERTEX_POINT('',#55158);
#14773=VERTEX_POINT('',#55160);
#14774=VERTEX_POINT('',#55164);
#14775=VERTEX_POINT('',#55166);
#14776=VERTEX_POINT('',#55170);
#14777=VERTEX_POINT('',#55172);
#14778=VERTEX_POINT('',#55176);
#14779=VERTEX_POINT('',#55178);
#14780=VERTEX_POINT('',#55182);
#14781=VERTEX_POINT('',#55184);
#14782=VERTEX_POINT('',#55188);
#14783=VERTEX_POINT('',#55190);
#14784=VERTEX_POINT('',#55194);
#14785=VERTEX_POINT('',#55196);
#14786=VERTEX_POINT('',#55203);
#14787=VERTEX_POINT('',#55204);
#14788=VERTEX_POINT('',#55206);
#14789=VERTEX_POINT('',#55208);
#14790=VERTEX_POINT('',#55212);
#14791=VERTEX_POINT('',#55214);
#14792=VERTEX_POINT('',#55218);
#14793=VERTEX_POINT('',#55220);
#14794=VERTEX_POINT('',#55224);
#14795=VERTEX_POINT('',#55226);
#14796=VERTEX_POINT('',#55230);
#14797=VERTEX_POINT('',#55232);
#14798=VERTEX_POINT('',#55236);
#14799=VERTEX_POINT('',#55238);
#14800=VERTEX_POINT('',#55242);
#14801=VERTEX_POINT('',#55244);
#18009=EDGE_CURVE('',#14322,#14323,#9101,.T.);
#18010=EDGE_CURVE('',#14324,#14323,#9102,.T.);
#18011=EDGE_CURVE('',#14325,#14324,#9103,.T.);
#18012=EDGE_CURVE('',#14325,#14322,#9104,.T.);
#18013=EDGE_CURVE('',#14323,#14326,#2744,.T.);
#18014=EDGE_CURVE('',#14327,#14326,#9105,.T.);
#18015=EDGE_CURVE('',#14324,#14327,#2745,.T.);
#18016=EDGE_CURVE('',#14326,#14328,#9106,.T.);
#18017=EDGE_CURVE('',#14329,#14328,#9107,.T.);
#18018=EDGE_CURVE('',#14327,#14329,#9108,.T.);
#18019=EDGE_CURVE('',#14328,#14330,#2746,.T.);
#18020=EDGE_CURVE('',#14331,#14330,#9109,.T.);
#18021=EDGE_CURVE('',#14329,#14331,#2747,.T.);
#18022=EDGE_CURVE('',#14332,#14333,#9110,.T.);
#18023=EDGE_CURVE('',#14334,#14333,#9111,.T.);
#18024=EDGE_CURVE('',#14335,#14334,#9112,.T.);
#18025=EDGE_CURVE('',#14335,#14332,#9113,.T.);
#18026=EDGE_CURVE('',#14333,#14336,#2748,.T.);
#18027=EDGE_CURVE('',#14337,#14336,#9114,.T.);
#18028=EDGE_CURVE('',#14334,#14337,#2749,.T.);
#18029=EDGE_CURVE('',#14336,#14338,#9115,.T.);
#18030=EDGE_CURVE('',#14339,#14338,#9116,.T.);
#18031=EDGE_CURVE('',#14337,#14339,#9117,.T.);
#18032=EDGE_CURVE('',#14338,#14340,#2750,.T.);
#18033=EDGE_CURVE('',#14341,#14340,#9118,.T.);
#18034=EDGE_CURVE('',#14339,#14341,#2751,.T.);
#18035=EDGE_CURVE('',#14330,#14342,#9119,.T.);
#18036=EDGE_CURVE('',#14343,#14342,#9120,.T.);
#18037=EDGE_CURVE('',#14331,#14343,#9121,.T.);
#18038=EDGE_CURVE('',#14344,#14322,#2752,.T.);
#18039=EDGE_CURVE('',#14345,#14325,#2753,.T.);
#18040=EDGE_CURVE('',#14345,#14344,#9122,.T.);
#18041=EDGE_CURVE('',#14346,#14344,#9123,.T.);
#18042=EDGE_CURVE('',#14347,#14345,#9124,.T.);
#18043=EDGE_CURVE('',#14347,#14346,#9125,.T.);
#18044=EDGE_CURVE('',#14342,#14346,#2754,.T.);
#18045=EDGE_CURVE('',#14343,#14347,#2755,.T.);
#18046=EDGE_CURVE('',#14340,#14348,#9126,.T.);
#18047=EDGE_CURVE('',#14349,#14348,#9127,.T.);
#18048=EDGE_CURVE('',#14341,#14349,#9128,.T.);
#18049=EDGE_CURVE('',#14348,#14350,#2756,.T.);
#18050=EDGE_CURVE('',#14351,#14350,#9129,.T.);
#18051=EDGE_CURVE('',#14349,#14351,#2757,.T.);
#18052=EDGE_CURVE('',#14350,#14352,#9130,.T.);
#18053=EDGE_CURVE('',#14353,#14352,#9131,.T.);
#18054=EDGE_CURVE('',#14351,#14353,#9132,.T.);
#18055=EDGE_CURVE('',#14352,#14332,#2758,.T.);
#18056=EDGE_CURVE('',#14353,#14335,#2759,.T.);
#18057=EDGE_CURVE('',#14354,#14355,#9133,.T.);
#18058=EDGE_CURVE('',#14356,#14355,#9134,.T.);
#18059=EDGE_CURVE('',#14357,#14356,#9135,.T.);
#18060=EDGE_CURVE('',#14357,#14354,#9136,.T.);
#18061=EDGE_CURVE('',#14355,#14358,#2760,.T.);
#18062=EDGE_CURVE('',#14359,#14358,#9137,.T.);
#18063=EDGE_CURVE('',#14356,#14359,#2761,.T.);
#18064=EDGE_CURVE('',#14358,#14360,#9138,.T.);
#18065=EDGE_CURVE('',#14361,#14360,#9139,.T.);
#18066=EDGE_CURVE('',#14359,#14361,#9140,.T.);
#18067=EDGE_CURVE('',#14360,#14362,#2762,.T.);
#18068=EDGE_CURVE('',#14363,#14362,#9141,.T.);
#18069=EDGE_CURVE('',#14361,#14363,#2763,.T.);
#18070=EDGE_CURVE('',#14364,#14365,#9142,.T.);
#18071=EDGE_CURVE('',#14366,#14365,#9143,.T.);
#18072=EDGE_CURVE('',#14367,#14366,#9144,.T.);
#18073=EDGE_CURVE('',#14367,#14364,#9145,.T.);
#18074=EDGE_CURVE('',#14365,#14368,#2764,.T.);
#18075=EDGE_CURVE('',#14369,#14368,#9146,.T.);
#18076=EDGE_CURVE('',#14366,#14369,#2765,.T.);
#18077=EDGE_CURVE('',#14368,#14370,#9147,.T.);
#18078=EDGE_CURVE('',#14371,#14370,#9148,.T.);
#18079=EDGE_CURVE('',#14369,#14371,#9149,.T.);
#18080=EDGE_CURVE('',#14370,#14372,#2766,.T.);
#18081=EDGE_CURVE('',#14373,#14372,#9150,.T.);
#18082=EDGE_CURVE('',#14371,#14373,#2767,.T.);
#18083=EDGE_CURVE('',#14362,#14374,#9151,.T.);
#18084=EDGE_CURVE('',#14375,#14374,#9152,.T.);
#18085=EDGE_CURVE('',#14363,#14375,#9153,.T.);
#18086=EDGE_CURVE('',#14376,#14354,#2768,.T.);
#18087=EDGE_CURVE('',#14377,#14357,#2769,.T.);
#18088=EDGE_CURVE('',#14377,#14376,#9154,.T.);
#18089=EDGE_CURVE('',#14378,#14376,#9155,.T.);
#18090=EDGE_CURVE('',#14379,#14377,#9156,.T.);
#18091=EDGE_CURVE('',#14379,#14378,#9157,.T.);
#18092=EDGE_CURVE('',#14374,#14378,#2770,.T.);
#18093=EDGE_CURVE('',#14375,#14379,#2771,.T.);
#18094=EDGE_CURVE('',#14372,#14380,#9158,.T.);
#18095=EDGE_CURVE('',#14381,#14380,#9159,.T.);
#18096=EDGE_CURVE('',#14373,#14381,#9160,.T.);
#18097=EDGE_CURVE('',#14380,#14382,#2772,.T.);
#18098=EDGE_CURVE('',#14383,#14382,#9161,.T.);
#18099=EDGE_CURVE('',#14381,#14383,#2773,.T.);
#18100=EDGE_CURVE('',#14382,#14384,#9162,.T.);
#18101=EDGE_CURVE('',#14385,#14384,#9163,.T.);
#18102=EDGE_CURVE('',#14383,#14385,#9164,.T.);
#18103=EDGE_CURVE('',#14384,#14364,#2774,.T.);
#18104=EDGE_CURVE('',#14385,#14367,#2775,.T.);
#18105=EDGE_CURVE('',#14386,#14387,#9165,.T.);
#18106=EDGE_CURVE('',#14388,#14387,#9166,.T.);
#18107=EDGE_CURVE('',#14389,#14388,#9167,.T.);
#18108=EDGE_CURVE('',#14389,#14386,#9168,.T.);
#18109=EDGE_CURVE('',#14387,#14390,#2776,.T.);
#18110=EDGE_CURVE('',#14391,#14390,#9169,.T.);
#18111=EDGE_CURVE('',#14388,#14391,#2777,.T.);
#18112=EDGE_CURVE('',#14390,#14392,#9170,.T.);
#18113=EDGE_CURVE('',#14393,#14392,#9171,.T.);
#18114=EDGE_CURVE('',#14391,#14393,#9172,.T.);
#18115=EDGE_CURVE('',#14392,#14394,#2778,.T.);
#18116=EDGE_CURVE('',#14395,#14394,#9173,.T.);
#18117=EDGE_CURVE('',#14393,#14395,#2779,.T.);
#18118=EDGE_CURVE('',#14396,#14397,#9174,.T.);
#18119=EDGE_CURVE('',#14398,#14397,#9175,.T.);
#18120=EDGE_CURVE('',#14399,#14398,#9176,.T.);
#18121=EDGE_CURVE('',#14399,#14396,#9177,.T.);
#18122=EDGE_CURVE('',#14397,#14400,#2780,.T.);
#18123=EDGE_CURVE('',#14401,#14400,#9178,.T.);
#18124=EDGE_CURVE('',#14398,#14401,#2781,.T.);
#18125=EDGE_CURVE('',#14400,#14402,#9179,.T.);
#18126=EDGE_CURVE('',#14403,#14402,#9180,.T.);
#18127=EDGE_CURVE('',#14401,#14403,#9181,.T.);
#18128=EDGE_CURVE('',#14402,#14404,#2782,.T.);
#18129=EDGE_CURVE('',#14405,#14404,#9182,.T.);
#18130=EDGE_CURVE('',#14403,#14405,#2783,.T.);
#18131=EDGE_CURVE('',#14394,#14406,#9183,.T.);
#18132=EDGE_CURVE('',#14407,#14406,#9184,.T.);
#18133=EDGE_CURVE('',#14395,#14407,#9185,.T.);
#18134=EDGE_CURVE('',#14408,#14386,#2784,.T.);
#18135=EDGE_CURVE('',#14409,#14389,#2785,.T.);
#18136=EDGE_CURVE('',#14409,#14408,#9186,.T.);
#18137=EDGE_CURVE('',#14410,#14408,#9187,.T.);
#18138=EDGE_CURVE('',#14411,#14409,#9188,.T.);
#18139=EDGE_CURVE('',#14411,#14410,#9189,.T.);
#18140=EDGE_CURVE('',#14406,#14410,#2786,.T.);
#18141=EDGE_CURVE('',#14407,#14411,#2787,.T.);
#18142=EDGE_CURVE('',#14404,#14412,#9190,.T.);
#18143=EDGE_CURVE('',#14413,#14412,#9191,.T.);
#18144=EDGE_CURVE('',#14405,#14413,#9192,.T.);
#18145=EDGE_CURVE('',#14412,#14414,#2788,.T.);
#18146=EDGE_CURVE('',#14415,#14414,#9193,.T.);
#18147=EDGE_CURVE('',#14413,#14415,#2789,.T.);
#18148=EDGE_CURVE('',#14414,#14416,#9194,.T.);
#18149=EDGE_CURVE('',#14417,#14416,#9195,.T.);
#18150=EDGE_CURVE('',#14415,#14417,#9196,.T.);
#18151=EDGE_CURVE('',#14416,#14396,#2790,.T.);
#18152=EDGE_CURVE('',#14417,#14399,#2791,.T.);
#18153=EDGE_CURVE('',#14418,#14419,#9197,.T.);
#18154=EDGE_CURVE('',#14420,#14419,#9198,.T.);
#18155=EDGE_CURVE('',#14421,#14420,#9199,.T.);
#18156=EDGE_CURVE('',#14421,#14418,#9200,.T.);
#18157=EDGE_CURVE('',#14419,#14422,#2792,.T.);
#18158=EDGE_CURVE('',#14423,#14422,#9201,.T.);
#18159=EDGE_CURVE('',#14420,#14423,#2793,.T.);
#18160=EDGE_CURVE('',#14422,#14424,#9202,.T.);
#18161=EDGE_CURVE('',#14425,#14424,#9203,.T.);
#18162=EDGE_CURVE('',#14423,#14425,#9204,.T.);
#18163=EDGE_CURVE('',#14424,#14426,#2794,.T.);
#18164=EDGE_CURVE('',#14427,#14426,#9205,.T.);
#18165=EDGE_CURVE('',#14425,#14427,#2795,.T.);
#18166=EDGE_CURVE('',#14428,#14429,#9206,.T.);
#18167=EDGE_CURVE('',#14430,#14429,#9207,.T.);
#18168=EDGE_CURVE('',#14431,#14430,#9208,.T.);
#18169=EDGE_CURVE('',#14431,#14428,#9209,.T.);
#18170=EDGE_CURVE('',#14429,#14432,#2796,.T.);
#18171=EDGE_CURVE('',#14433,#14432,#9210,.T.);
#18172=EDGE_CURVE('',#14430,#14433,#2797,.T.);
#18173=EDGE_CURVE('',#14432,#14434,#9211,.T.);
#18174=EDGE_CURVE('',#14435,#14434,#9212,.T.);
#18175=EDGE_CURVE('',#14433,#14435,#9213,.T.);
#18176=EDGE_CURVE('',#14434,#14436,#2798,.T.);
#18177=EDGE_CURVE('',#14437,#14436,#9214,.T.);
#18178=EDGE_CURVE('',#14435,#14437,#2799,.T.);
#18179=EDGE_CURVE('',#14426,#14438,#9215,.T.);
#18180=EDGE_CURVE('',#14439,#14438,#9216,.T.);
#18181=EDGE_CURVE('',#14427,#14439,#9217,.T.);
#18182=EDGE_CURVE('',#14440,#14418,#2800,.T.);
#18183=EDGE_CURVE('',#14441,#14421,#2801,.T.);
#18184=EDGE_CURVE('',#14441,#14440,#9218,.T.);
#18185=EDGE_CURVE('',#14442,#14440,#9219,.T.);
#18186=EDGE_CURVE('',#14443,#14441,#9220,.T.);
#18187=EDGE_CURVE('',#14443,#14442,#9221,.T.);
#18188=EDGE_CURVE('',#14438,#14442,#2802,.T.);
#18189=EDGE_CURVE('',#14439,#14443,#2803,.T.);
#18190=EDGE_CURVE('',#14436,#14444,#9222,.T.);
#18191=EDGE_CURVE('',#14445,#14444,#9223,.T.);
#18192=EDGE_CURVE('',#14437,#14445,#9224,.T.);
#18193=EDGE_CURVE('',#14444,#14446,#2804,.T.);
#18194=EDGE_CURVE('',#14447,#14446,#9225,.T.);
#18195=EDGE_CURVE('',#14445,#14447,#2805,.T.);
#18196=EDGE_CURVE('',#14446,#14448,#9226,.T.);
#18197=EDGE_CURVE('',#14449,#14448,#9227,.T.);
#18198=EDGE_CURVE('',#14447,#14449,#9228,.T.);
#18199=EDGE_CURVE('',#14448,#14428,#2806,.T.);
#18200=EDGE_CURVE('',#14449,#14431,#2807,.T.);
#18201=EDGE_CURVE('',#14450,#14451,#394,.T.);
#18202=EDGE_CURVE('',#14452,#14450,#9229,.T.);
#18203=EDGE_CURVE('',#14453,#14452,#395,.T.);
#18204=EDGE_CURVE('',#14453,#14454,#9230,.T.);
#18205=EDGE_CURVE('',#14455,#14454,#396,.T.);
#18206=EDGE_CURVE('',#14456,#14455,#9231,.T.);
#18207=EDGE_CURVE('',#14457,#14456,#397,.T.);
#18208=EDGE_CURVE('',#14451,#14457,#9232,.T.);
#18209=EDGE_CURVE('',#14458,#14459,#9233,.T.);
#18210=EDGE_CURVE('',#14460,#14458,#398,.T.);
#18211=EDGE_CURVE('',#14461,#14460,#9234,.T.);
#18212=EDGE_CURVE('',#14462,#14461,#399,.T.);
#18213=EDGE_CURVE('',#14463,#14462,#9235,.T.);
#18214=EDGE_CURVE('',#14464,#14463,#400,.T.);
#18215=EDGE_CURVE('',#14465,#14464,#9236,.T.);
#18216=EDGE_CURVE('',#14459,#14465,#401,.T.);
#18217=EDGE_CURVE('',#14462,#14466,#9237,.T.);
#18218=EDGE_CURVE('',#14466,#14467,#9238,.T.);
#18219=EDGE_CURVE('',#14463,#14467,#9239,.T.);
#18220=EDGE_CURVE('',#14461,#14468,#9240,.T.);
#18221=EDGE_CURVE('',#14468,#14466,#402,.T.);
#18222=EDGE_CURVE('',#14460,#14469,#9241,.T.);
#18223=EDGE_CURVE('',#14469,#14468,#9242,.T.);
#18224=EDGE_CURVE('',#14458,#14470,#9243,.T.);
#18225=EDGE_CURVE('',#14470,#14469,#403,.T.);
#18226=EDGE_CURVE('',#14454,#14471,#9244,.T.);
#18227=EDGE_CURVE('',#14471,#14472,#404,.T.);
#18228=EDGE_CURVE('',#14455,#14472,#9245,.T.);
#18229=EDGE_CURVE('',#14452,#14473,#9246,.T.);
#18230=EDGE_CURVE('',#14473,#14474,#405,.T.);
#18231=EDGE_CURVE('',#14453,#14474,#9247,.T.);
#18232=EDGE_CURVE('',#14450,#14475,#9248,.T.);
#18233=EDGE_CURVE('',#14475,#14473,#9249,.T.);
#18234=EDGE_CURVE('',#14474,#14471,#9250,.T.);
#18235=EDGE_CURVE('',#14476,#14475,#406,.T.);
#18236=EDGE_CURVE('',#14477,#14476,#9251,.T.);
#18237=EDGE_CURVE('',#14478,#14477,#407,.T.);
#18238=EDGE_CURVE('',#14472,#14478,#9252,.T.);
#18239=EDGE_CURVE('',#14479,#14470,#9253,.T.);
#18240=EDGE_CURVE('',#14480,#14479,#408,.T.);
#18241=EDGE_CURVE('',#14481,#14480,#9254,.T.);
#18242=EDGE_CURVE('',#14467,#14481,#409,.T.);
#18243=EDGE_CURVE('',#14459,#14479,#9255,.T.);
#18244=EDGE_CURVE('',#14451,#14476,#9256,.T.);
#18245=EDGE_CURVE('',#14464,#14481,#9257,.T.);
#18246=EDGE_CURVE('',#14465,#14480,#9258,.T.);
#18247=EDGE_CURVE('',#14456,#14478,#9259,.T.);
#18248=EDGE_CURVE('',#14457,#14477,#9260,.T.);
#18249=EDGE_CURVE('',#14482,#14483,#410,.T.);
#18250=EDGE_CURVE('',#14484,#14482,#9261,.T.);
#18251=EDGE_CURVE('',#14485,#14484,#411,.T.);
#18252=EDGE_CURVE('',#14486,#14485,#9262,.T.);
#18253=EDGE_CURVE('',#14487,#14486,#412,.T.);
#18254=EDGE_CURVE('',#14488,#14487,#9263,.T.);
#18255=EDGE_CURVE('',#14489,#14488,#413,.T.);
#18256=EDGE_CURVE('',#14489,#14483,#9264,.T.);
#18257=EDGE_CURVE('',#14490,#14491,#9265,.T.);
#18258=EDGE_CURVE('',#14492,#14490,#414,.T.);
#18259=EDGE_CURVE('',#14493,#14492,#9266,.T.);
#18260=EDGE_CURVE('',#14494,#14493,#415,.T.);
#18261=EDGE_CURVE('',#14495,#14494,#9267,.T.);
#18262=EDGE_CURVE('',#14496,#14495,#416,.T.);
#18263=EDGE_CURVE('',#14497,#14496,#9268,.T.);
#18264=EDGE_CURVE('',#14491,#14497,#417,.T.);
#18265=EDGE_CURVE('',#14494,#14498,#9269,.T.);
#18266=EDGE_CURVE('',#14498,#14499,#9270,.T.);
#18267=EDGE_CURVE('',#14495,#14499,#9271,.T.);
#18268=EDGE_CURVE('',#14493,#14500,#9272,.T.);
#18269=EDGE_CURVE('',#14500,#14498,#418,.T.);
#18270=EDGE_CURVE('',#14492,#14501,#9273,.T.);
#18271=EDGE_CURVE('',#14501,#14500,#9274,.T.);
#18272=EDGE_CURVE('',#14490,#14502,#9275,.T.);
#18273=EDGE_CURVE('',#14502,#14501,#419,.T.);
#18274=EDGE_CURVE('',#14486,#14503,#9276,.T.);
#18275=EDGE_CURVE('',#14503,#14504,#420,.T.);
#18276=EDGE_CURVE('',#14487,#14504,#9277,.T.);
#18277=EDGE_CURVE('',#14485,#14505,#9278,.T.);
#18278=EDGE_CURVE('',#14505,#14503,#9279,.T.);
#18279=EDGE_CURVE('',#14484,#14506,#9280,.T.);
#18280=EDGE_CURVE('',#14506,#14505,#421,.T.);
#18281=EDGE_CURVE('',#14482,#14507,#9281,.T.);
#18282=EDGE_CURVE('',#14507,#14506,#9282,.T.);
#18283=EDGE_CURVE('',#14508,#14507,#422,.T.);
#18284=EDGE_CURVE('',#14509,#14508,#9283,.T.);
#18285=EDGE_CURVE('',#14510,#14509,#423,.T.);
#18286=EDGE_CURVE('',#14504,#14510,#9284,.T.);
#18287=EDGE_CURVE('',#14511,#14502,#9285,.T.);
#18288=EDGE_CURVE('',#14512,#14511,#424,.T.);
#18289=EDGE_CURVE('',#14513,#14512,#9286,.T.);
#18290=EDGE_CURVE('',#14499,#14513,#425,.T.);
#18291=EDGE_CURVE('',#14491,#14511,#9287,.T.);
#18292=EDGE_CURVE('',#14483,#14508,#9288,.T.);
#18293=EDGE_CURVE('',#14496,#14513,#9289,.T.);
#18294=EDGE_CURVE('',#14497,#14512,#9290,.T.);
#18295=EDGE_CURVE('',#14488,#14510,#9291,.T.);
#18296=EDGE_CURVE('',#14489,#14509,#9292,.T.);
#18297=EDGE_CURVE('',#14514,#14515,#9293,.T.);
#18298=EDGE_CURVE('',#14516,#14514,#426,.T.);
#18299=EDGE_CURVE('',#14517,#14516,#9294,.T.);
#18300=EDGE_CURVE('',#14518,#14517,#427,.T.);
#18301=EDGE_CURVE('',#14519,#14518,#9295,.T.);
#18302=EDGE_CURVE('',#14520,#14519,#428,.T.);
#18303=EDGE_CURVE('',#14521,#14520,#9296,.T.);
#18304=EDGE_CURVE('',#14515,#14521,#429,.T.);
#18305=EDGE_CURVE('',#14522,#14523,#9297,.T.);
#18306=EDGE_CURVE('',#14524,#14522,#430,.T.);
#18307=EDGE_CURVE('',#14525,#14524,#9298,.T.);
#18308=EDGE_CURVE('',#14526,#14525,#431,.T.);
#18309=EDGE_CURVE('',#14527,#14526,#9299,.T.);
#18310=EDGE_CURVE('',#14528,#14527,#432,.T.);
#18311=EDGE_CURVE('',#14529,#14528,#9300,.T.);
#18312=EDGE_CURVE('',#14523,#14529,#433,.T.);
#18313=EDGE_CURVE('',#14526,#14530,#9301,.T.);
#18314=EDGE_CURVE('',#14530,#14531,#9302,.T.);
#18315=EDGE_CURVE('',#14527,#14531,#9303,.T.);
#18316=EDGE_CURVE('',#14525,#14532,#9304,.T.);
#18317=EDGE_CURVE('',#14532,#14530,#434,.T.);
#18318=EDGE_CURVE('',#14524,#14533,#9305,.T.);
#18319=EDGE_CURVE('',#14533,#14532,#9306,.T.);
#18320=EDGE_CURVE('',#14522,#14534,#9307,.T.);
#18321=EDGE_CURVE('',#14534,#14533,#435,.T.);
#18322=EDGE_CURVE('',#14518,#14535,#9308,.T.);
#18323=EDGE_CURVE('',#14535,#14536,#9309,.T.);
#18324=EDGE_CURVE('',#14519,#14536,#9310,.T.);
#18325=EDGE_CURVE('',#14517,#14537,#9311,.T.);
#18326=EDGE_CURVE('',#14537,#14535,#436,.T.);
#18327=EDGE_CURVE('',#14538,#14516,#9312,.T.);
#18328=EDGE_CURVE('',#14538,#14537,#9313,.T.);
#18329=EDGE_CURVE('',#14514,#14539,#9314,.T.);
#18330=EDGE_CURVE('',#14539,#14538,#437,.T.);
#18331=EDGE_CURVE('',#14540,#14539,#9315,.T.);
#18332=EDGE_CURVE('',#14541,#14540,#438,.T.);
#18333=EDGE_CURVE('',#14541,#14542,#9316,.T.);
#18334=EDGE_CURVE('',#14536,#14542,#439,.T.);
#18335=EDGE_CURVE('',#14543,#14534,#9317,.T.);
#18336=EDGE_CURVE('',#14544,#14543,#440,.T.);
#18337=EDGE_CURVE('',#14545,#14544,#9318,.T.);
#18338=EDGE_CURVE('',#14531,#14545,#441,.T.);
#18339=EDGE_CURVE('',#14523,#14543,#9319,.T.);
#18340=EDGE_CURVE('',#14515,#14540,#9320,.T.);
#18341=EDGE_CURVE('',#14528,#14545,#9321,.T.);
#18342=EDGE_CURVE('',#14544,#14529,#9322,.T.);
#18343=EDGE_CURVE('',#14521,#14541,#9323,.T.);
#18344=EDGE_CURVE('',#14520,#14542,#9324,.T.);
#18345=EDGE_CURVE('',#14546,#14547,#9325,.T.);
#18346=EDGE_CURVE('',#14548,#14546,#442,.T.);
#18347=EDGE_CURVE('',#14549,#14548,#9326,.T.);
#18348=EDGE_CURVE('',#14550,#14549,#443,.T.);
#18349=EDGE_CURVE('',#14551,#14550,#9327,.T.);
#18350=EDGE_CURVE('',#14552,#14551,#444,.T.);
#18351=EDGE_CURVE('',#14552,#14553,#9328,.T.);
#18352=EDGE_CURVE('',#14547,#14553,#445,.T.);
#18353=EDGE_CURVE('',#14554,#14555,#9329,.T.);
#18354=EDGE_CURVE('',#14556,#14554,#446,.T.);
#18355=EDGE_CURVE('',#14557,#14556,#9330,.T.);
#18356=EDGE_CURVE('',#14558,#14557,#447,.T.);
#18357=EDGE_CURVE('',#14559,#14558,#9331,.T.);
#18358=EDGE_CURVE('',#14560,#14559,#448,.T.);
#18359=EDGE_CURVE('',#14561,#14560,#9332,.T.);
#18360=EDGE_CURVE('',#14555,#14561,#449,.T.);
#18361=EDGE_CURVE('',#14558,#14562,#9333,.T.);
#18362=EDGE_CURVE('',#14562,#14563,#9334,.T.);
#18363=EDGE_CURVE('',#14559,#14563,#9335,.T.);
#18364=EDGE_CURVE('',#14557,#14564,#9336,.T.);
#18365=EDGE_CURVE('',#14564,#14562,#450,.T.);
#18366=EDGE_CURVE('',#14556,#14565,#9337,.T.);
#18367=EDGE_CURVE('',#14565,#14564,#9338,.T.);
#18368=EDGE_CURVE('',#14554,#14566,#9339,.T.);
#18369=EDGE_CURVE('',#14566,#14565,#451,.T.);
#18370=EDGE_CURVE('',#14550,#14567,#9340,.T.);
#18371=EDGE_CURVE('',#14567,#14568,#9341,.T.);
#18372=EDGE_CURVE('',#14551,#14568,#9342,.T.);
#18373=EDGE_CURVE('',#14549,#14569,#9343,.T.);
#18374=EDGE_CURVE('',#14569,#14567,#452,.T.);
#18375=EDGE_CURVE('',#14548,#14570,#9344,.T.);
#18376=EDGE_CURVE('',#14570,#14569,#9345,.T.);
#18377=EDGE_CURVE('',#14546,#14571,#9346,.T.);
#18378=EDGE_CURVE('',#14571,#14570,#453,.T.);
#18379=EDGE_CURVE('',#14572,#14571,#9347,.T.);
#18380=EDGE_CURVE('',#14573,#14572,#454,.T.);
#18381=EDGE_CURVE('',#14574,#14573,#9348,.T.);
#18382=EDGE_CURVE('',#14568,#14574,#455,.T.);
#18383=EDGE_CURVE('',#14575,#14566,#9349,.T.);
#18384=EDGE_CURVE('',#14576,#14575,#456,.T.);
#18385=EDGE_CURVE('',#14577,#14576,#9350,.T.);
#18386=EDGE_CURVE('',#14563,#14577,#457,.T.);
#18387=EDGE_CURVE('',#14555,#14575,#9351,.T.);
#18388=EDGE_CURVE('',#14547,#14572,#9352,.T.);
#18389=EDGE_CURVE('',#14560,#14577,#9353,.T.);
#18390=EDGE_CURVE('',#14561,#14576,#9354,.T.);
#18391=EDGE_CURVE('',#14552,#14574,#9355,.T.);
#18392=EDGE_CURVE('',#14553,#14573,#9356,.T.);
#18393=EDGE_CURVE('',#14578,#14579,#9357,.T.);
#18394=EDGE_CURVE('',#14580,#14579,#9358,.T.);
#18395=EDGE_CURVE('',#14581,#14580,#9359,.T.);
#18396=EDGE_CURVE('',#14581,#14578,#9360,.T.);
#18397=EDGE_CURVE('',#14579,#14582,#2808,.T.);
#18398=EDGE_CURVE('',#14583,#14582,#9361,.T.);
#18399=EDGE_CURVE('',#14580,#14583,#2809,.T.);
#18400=EDGE_CURVE('',#14582,#14584,#9362,.T.);
#18401=EDGE_CURVE('',#14585,#14584,#9363,.T.);
#18402=EDGE_CURVE('',#14583,#14585,#9364,.T.);
#18403=EDGE_CURVE('',#14584,#14586,#2810,.T.);
#18404=EDGE_CURVE('',#14587,#14586,#9365,.T.);
#18405=EDGE_CURVE('',#14585,#14587,#2811,.T.);
#18406=EDGE_CURVE('',#14588,#14589,#9366,.T.);
#18407=EDGE_CURVE('',#14590,#14589,#9367,.T.);
#18408=EDGE_CURVE('',#14591,#14590,#9368,.T.);
#18409=EDGE_CURVE('',#14591,#14588,#9369,.T.);
#18410=EDGE_CURVE('',#14589,#14592,#2812,.T.);
#18411=EDGE_CURVE('',#14593,#14592,#9370,.T.);
#18412=EDGE_CURVE('',#14590,#14593,#2813,.T.);
#18413=EDGE_CURVE('',#14592,#14594,#9371,.T.);
#18414=EDGE_CURVE('',#14595,#14594,#9372,.T.);
#18415=EDGE_CURVE('',#14593,#14595,#9373,.T.);
#18416=EDGE_CURVE('',#14594,#14596,#2814,.T.);
#18417=EDGE_CURVE('',#14597,#14596,#9374,.T.);
#18418=EDGE_CURVE('',#14595,#14597,#2815,.T.);
#18419=EDGE_CURVE('',#14586,#14598,#9375,.T.);
#18420=EDGE_CURVE('',#14599,#14598,#9376,.T.);
#18421=EDGE_CURVE('',#14587,#14599,#9377,.T.);
#18422=EDGE_CURVE('',#14600,#14578,#2816,.T.);
#18423=EDGE_CURVE('',#14601,#14581,#2817,.T.);
#18424=EDGE_CURVE('',#14601,#14600,#9378,.T.);
#18425=EDGE_CURVE('',#14602,#14600,#9379,.T.);
#18426=EDGE_CURVE('',#14603,#14601,#9380,.T.);
#18427=EDGE_CURVE('',#14603,#14602,#9381,.T.);
#18428=EDGE_CURVE('',#14598,#14602,#2818,.T.);
#18429=EDGE_CURVE('',#14599,#14603,#2819,.T.);
#18430=EDGE_CURVE('',#14596,#14604,#9382,.T.);
#18431=EDGE_CURVE('',#14605,#14604,#9383,.T.);
#18432=EDGE_CURVE('',#14597,#14605,#9384,.T.);
#18433=EDGE_CURVE('',#14604,#14606,#2820,.T.);
#18434=EDGE_CURVE('',#14607,#14606,#9385,.T.);
#18435=EDGE_CURVE('',#14605,#14607,#2821,.T.);
#18436=EDGE_CURVE('',#14606,#14608,#9386,.T.);
#18437=EDGE_CURVE('',#14609,#14608,#9387,.T.);
#18438=EDGE_CURVE('',#14607,#14609,#9388,.T.);
#18439=EDGE_CURVE('',#14608,#14588,#2822,.T.);
#18440=EDGE_CURVE('',#14609,#14591,#2823,.T.);
#18441=EDGE_CURVE('',#14610,#14611,#9389,.T.);
#18442=EDGE_CURVE('',#14612,#14611,#9390,.T.);
#18443=EDGE_CURVE('',#14613,#14612,#9391,.T.);
#18444=EDGE_CURVE('',#14613,#14610,#9392,.T.);
#18445=EDGE_CURVE('',#14611,#14614,#2824,.T.);
#18446=EDGE_CURVE('',#14615,#14614,#9393,.T.);
#18447=EDGE_CURVE('',#14612,#14615,#2825,.T.);
#18448=EDGE_CURVE('',#14614,#14616,#9394,.T.);
#18449=EDGE_CURVE('',#14617,#14616,#9395,.T.);
#18450=EDGE_CURVE('',#14615,#14617,#9396,.T.);
#18451=EDGE_CURVE('',#14616,#14618,#2826,.T.);
#18452=EDGE_CURVE('',#14619,#14618,#9397,.T.);
#18453=EDGE_CURVE('',#14617,#14619,#2827,.T.);
#18454=EDGE_CURVE('',#14620,#14621,#9398,.T.);
#18455=EDGE_CURVE('',#14622,#14621,#9399,.T.);
#18456=EDGE_CURVE('',#14623,#14622,#9400,.T.);
#18457=EDGE_CURVE('',#14623,#14620,#9401,.T.);
#18458=EDGE_CURVE('',#14621,#14624,#2828,.T.);
#18459=EDGE_CURVE('',#14625,#14624,#9402,.T.);
#18460=EDGE_CURVE('',#14622,#14625,#2829,.T.);
#18461=EDGE_CURVE('',#14624,#14626,#9403,.T.);
#18462=EDGE_CURVE('',#14627,#14626,#9404,.T.);
#18463=EDGE_CURVE('',#14625,#14627,#9405,.T.);
#18464=EDGE_CURVE('',#14626,#14628,#2830,.T.);
#18465=EDGE_CURVE('',#14629,#14628,#9406,.T.);
#18466=EDGE_CURVE('',#14627,#14629,#2831,.T.);
#18467=EDGE_CURVE('',#14618,#14630,#9407,.T.);
#18468=EDGE_CURVE('',#14631,#14630,#9408,.T.);
#18469=EDGE_CURVE('',#14619,#14631,#9409,.T.);
#18470=EDGE_CURVE('',#14632,#14610,#2832,.T.);
#18471=EDGE_CURVE('',#14633,#14613,#2833,.T.);
#18472=EDGE_CURVE('',#14633,#14632,#9410,.T.);
#18473=EDGE_CURVE('',#14634,#14632,#9411,.T.);
#18474=EDGE_CURVE('',#14635,#14633,#9412,.T.);
#18475=EDGE_CURVE('',#14635,#14634,#9413,.T.);
#18476=EDGE_CURVE('',#14630,#14634,#2834,.T.);
#18477=EDGE_CURVE('',#14631,#14635,#2835,.T.);
#18478=EDGE_CURVE('',#14628,#14636,#9414,.T.);
#18479=EDGE_CURVE('',#14637,#14636,#9415,.T.);
#18480=EDGE_CURVE('',#14629,#14637,#9416,.T.);
#18481=EDGE_CURVE('',#14636,#14638,#2836,.T.);
#18482=EDGE_CURVE('',#14639,#14638,#9417,.T.);
#18483=EDGE_CURVE('',#14637,#14639,#2837,.T.);
#18484=EDGE_CURVE('',#14638,#14640,#9418,.T.);
#18485=EDGE_CURVE('',#14641,#14640,#9419,.T.);
#18486=EDGE_CURVE('',#14639,#14641,#9420,.T.);
#18487=EDGE_CURVE('',#14640,#14620,#2838,.T.);
#18488=EDGE_CURVE('',#14641,#14623,#2839,.T.);
#18489=EDGE_CURVE('',#14642,#14643,#9421,.T.);
#18490=EDGE_CURVE('',#14644,#14643,#9422,.T.);
#18491=EDGE_CURVE('',#14645,#14644,#9423,.T.);
#18492=EDGE_CURVE('',#14645,#14642,#9424,.T.);
#18493=EDGE_CURVE('',#14643,#14646,#2840,.T.);
#18494=EDGE_CURVE('',#14647,#14646,#9425,.T.);
#18495=EDGE_CURVE('',#14644,#14647,#2841,.T.);
#18496=EDGE_CURVE('',#14646,#14648,#9426,.T.);
#18497=EDGE_CURVE('',#14649,#14648,#9427,.T.);
#18498=EDGE_CURVE('',#14647,#14649,#9428,.T.);
#18499=EDGE_CURVE('',#14648,#14650,#2842,.T.);
#18500=EDGE_CURVE('',#14651,#14650,#9429,.T.);
#18501=EDGE_CURVE('',#14649,#14651,#2843,.T.);
#18502=EDGE_CURVE('',#14652,#14653,#9430,.T.);
#18503=EDGE_CURVE('',#14654,#14653,#9431,.T.);
#18504=EDGE_CURVE('',#14655,#14654,#9432,.T.);
#18505=EDGE_CURVE('',#14655,#14652,#9433,.T.);
#18506=EDGE_CURVE('',#14653,#14656,#2844,.T.);
#18507=EDGE_CURVE('',#14657,#14656,#9434,.T.);
#18508=EDGE_CURVE('',#14654,#14657,#2845,.T.);
#18509=EDGE_CURVE('',#14656,#14658,#9435,.T.);
#18510=EDGE_CURVE('',#14659,#14658,#9436,.T.);
#18511=EDGE_CURVE('',#14657,#14659,#9437,.T.);
#18512=EDGE_CURVE('',#14658,#14660,#2846,.T.);
#18513=EDGE_CURVE('',#14661,#14660,#9438,.T.);
#18514=EDGE_CURVE('',#14659,#14661,#2847,.T.);
#18515=EDGE_CURVE('',#14650,#14662,#9439,.T.);
#18516=EDGE_CURVE('',#14663,#14662,#9440,.T.);
#18517=EDGE_CURVE('',#14651,#14663,#9441,.T.);
#18518=EDGE_CURVE('',#14664,#14642,#2848,.T.);
#18519=EDGE_CURVE('',#14665,#14645,#2849,.T.);
#18520=EDGE_CURVE('',#14665,#14664,#9442,.T.);
#18521=EDGE_CURVE('',#14666,#14664,#9443,.T.);
#18522=EDGE_CURVE('',#14667,#14665,#9444,.T.);
#18523=EDGE_CURVE('',#14667,#14666,#9445,.T.);
#18524=EDGE_CURVE('',#14662,#14666,#2850,.T.);
#18525=EDGE_CURVE('',#14663,#14667,#2851,.T.);
#18526=EDGE_CURVE('',#14660,#14668,#9446,.T.);
#18527=EDGE_CURVE('',#14669,#14668,#9447,.T.);
#18528=EDGE_CURVE('',#14661,#14669,#9448,.T.);
#18529=EDGE_CURVE('',#14668,#14670,#2852,.T.);
#18530=EDGE_CURVE('',#14671,#14670,#9449,.T.);
#18531=EDGE_CURVE('',#14669,#14671,#2853,.T.);
#18532=EDGE_CURVE('',#14670,#14672,#9450,.T.);
#18533=EDGE_CURVE('',#14673,#14672,#9451,.T.);
#18534=EDGE_CURVE('',#14671,#14673,#9452,.T.);
#18535=EDGE_CURVE('',#14672,#14652,#2854,.T.);
#18536=EDGE_CURVE('',#14673,#14655,#2855,.T.);
#18537=EDGE_CURVE('',#14674,#14675,#2856,.T.);
#18538=EDGE_CURVE('',#14674,#14676,#9453,.T.);
#18539=EDGE_CURVE('',#14677,#14676,#2857,.T.);
#18540=EDGE_CURVE('',#14675,#14677,#9454,.T.);
#18541=EDGE_CURVE('',#14678,#14674,#9455,.T.);
#18542=EDGE_CURVE('',#14678,#14679,#9456,.T.);
#18543=EDGE_CURVE('',#14676,#14679,#9457,.T.);
#18544=EDGE_CURVE('',#14680,#14678,#2858,.T.);
#18545=EDGE_CURVE('',#14680,#14681,#9458,.T.);
#18546=EDGE_CURVE('',#14679,#14681,#2859,.T.);
#18547=EDGE_CURVE('',#14682,#14680,#9459,.T.);
#18548=EDGE_CURVE('',#14682,#14683,#9460,.T.);
#18549=EDGE_CURVE('',#14681,#14683,#9461,.T.);
#18550=EDGE_CURVE('',#14684,#14682,#2860,.T.);
#18551=EDGE_CURVE('',#14684,#14685,#9462,.T.);
#18552=EDGE_CURVE('',#14683,#14685,#2861,.T.);
#18553=EDGE_CURVE('',#14686,#14684,#9463,.T.);
#18554=EDGE_CURVE('',#14686,#14687,#9464,.T.);
#18555=EDGE_CURVE('',#14685,#14687,#9465,.T.);
#18556=EDGE_CURVE('',#14688,#14686,#2862,.T.);
#18557=EDGE_CURVE('',#14688,#14689,#9466,.T.);
#18558=EDGE_CURVE('',#14687,#14689,#2863,.T.);
#18559=EDGE_CURVE('',#14675,#14688,#9467,.T.);
#18560=EDGE_CURVE('',#14689,#14677,#9468,.T.);
#18561=EDGE_CURVE('',#14690,#14691,#2864,.T.);
#18562=EDGE_CURVE('',#14690,#14692,#9469,.T.);
#18563=EDGE_CURVE('',#14693,#14692,#2865,.T.);
#18564=EDGE_CURVE('',#14691,#14693,#9470,.T.);
#18565=EDGE_CURVE('',#14691,#14694,#9471,.T.);
#18566=EDGE_CURVE('',#14695,#14693,#9472,.T.);
#18567=EDGE_CURVE('',#14694,#14695,#9473,.T.);
#18568=EDGE_CURVE('',#14694,#14696,#2866,.T.);
#18569=EDGE_CURVE('',#14697,#14695,#2867,.T.);
#18570=EDGE_CURVE('',#14696,#14697,#9474,.T.);
#18571=EDGE_CURVE('',#14696,#14698,#9475,.T.);
#18572=EDGE_CURVE('',#14699,#14697,#9476,.T.);
#18573=EDGE_CURVE('',#14698,#14699,#9477,.T.);
#18574=EDGE_CURVE('',#14698,#14700,#2868,.T.);
#18575=EDGE_CURVE('',#14701,#14699,#2869,.T.);
#18576=EDGE_CURVE('',#14700,#14701,#9478,.T.);
#18577=EDGE_CURVE('',#14700,#14702,#9479,.T.);
#18578=EDGE_CURVE('',#14703,#14701,#9480,.T.);
#18579=EDGE_CURVE('',#14702,#14703,#9481,.T.);
#18580=EDGE_CURVE('',#14702,#14704,#2870,.T.);
#18581=EDGE_CURVE('',#14705,#14703,#2871,.T.);
#18582=EDGE_CURVE('',#14704,#14705,#9482,.T.);
#18583=EDGE_CURVE('',#14704,#14690,#9483,.T.);
#18584=EDGE_CURVE('',#14692,#14705,#9484,.T.);
#18585=EDGE_CURVE('',#14706,#14707,#2872,.T.);
#18586=EDGE_CURVE('',#14706,#14708,#9485,.T.);
#18587=EDGE_CURVE('',#14709,#14708,#2873,.T.);
#18588=EDGE_CURVE('',#14707,#14709,#9486,.T.);
#18589=EDGE_CURVE('',#14710,#14706,#9487,.T.);
#18590=EDGE_CURVE('',#14710,#14711,#9488,.T.);
#18591=EDGE_CURVE('',#14708,#14711,#9489,.T.);
#18592=EDGE_CURVE('',#14712,#14710,#2874,.T.);
#18593=EDGE_CURVE('',#14712,#14713,#9490,.T.);
#18594=EDGE_CURVE('',#14711,#14713,#2875,.T.);
#18595=EDGE_CURVE('',#14714,#14712,#9491,.T.);
#18596=EDGE_CURVE('',#14714,#14715,#9492,.T.);
#18597=EDGE_CURVE('',#14713,#14715,#9493,.T.);
#18598=EDGE_CURVE('',#14716,#14714,#2876,.T.);
#18599=EDGE_CURVE('',#14716,#14717,#9494,.T.);
#18600=EDGE_CURVE('',#14715,#14717,#2877,.T.);
#18601=EDGE_CURVE('',#14718,#14716,#9495,.T.);
#18602=EDGE_CURVE('',#14718,#14719,#9496,.T.);
#18603=EDGE_CURVE('',#14717,#14719,#9497,.T.);
#18604=EDGE_CURVE('',#14720,#14718,#2878,.T.);
#18605=EDGE_CURVE('',#14720,#14721,#9498,.T.);
#18606=EDGE_CURVE('',#14719,#14721,#2879,.T.);
#18607=EDGE_CURVE('',#14707,#14720,#9499,.T.);
#18608=EDGE_CURVE('',#14721,#14709,#9500,.T.);
#18609=EDGE_CURVE('',#14722,#14723,#2880,.T.);
#18610=EDGE_CURVE('',#14722,#14724,#9501,.T.);
#18611=EDGE_CURVE('',#14725,#14724,#2881,.T.);
#18612=EDGE_CURVE('',#14723,#14725,#9502,.T.);
#18613=EDGE_CURVE('',#14723,#14726,#9503,.T.);
#18614=EDGE_CURVE('',#14727,#14725,#9504,.T.);
#18615=EDGE_CURVE('',#14726,#14727,#9505,.T.);
#18616=EDGE_CURVE('',#14726,#14728,#2882,.T.);
#18617=EDGE_CURVE('',#14729,#14727,#2883,.T.);
#18618=EDGE_CURVE('',#14728,#14729,#9506,.T.);
#18619=EDGE_CURVE('',#14728,#14730,#9507,.T.);
#18620=EDGE_CURVE('',#14731,#14729,#9508,.T.);
#18621=EDGE_CURVE('',#14730,#14731,#9509,.T.);
#18622=EDGE_CURVE('',#14730,#14732,#2884,.T.);
#18623=EDGE_CURVE('',#14733,#14731,#2885,.T.);
#18624=EDGE_CURVE('',#14732,#14733,#9510,.T.);
#18625=EDGE_CURVE('',#14732,#14734,#9511,.T.);
#18626=EDGE_CURVE('',#14735,#14733,#9512,.T.);
#18627=EDGE_CURVE('',#14734,#14735,#9513,.T.);
#18628=EDGE_CURVE('',#14734,#14736,#2886,.T.);
#18629=EDGE_CURVE('',#14737,#14735,#2887,.T.);
#18630=EDGE_CURVE('',#14736,#14737,#9514,.T.);
#18631=EDGE_CURVE('',#14736,#14722,#9515,.T.);
#18632=EDGE_CURVE('',#14724,#14737,#9516,.T.);
#18633=EDGE_CURVE('',#14738,#14739,#2888,.T.);
#18634=EDGE_CURVE('',#14738,#14740,#9517,.T.);
#18635=EDGE_CURVE('',#14741,#14740,#2889,.T.);
#18636=EDGE_CURVE('',#14739,#14741,#9518,.T.);
#18637=EDGE_CURVE('',#14742,#14738,#9519,.T.);
#18638=EDGE_CURVE('',#14742,#14743,#9520,.T.);
#18639=EDGE_CURVE('',#14740,#14743,#9521,.T.);
#18640=EDGE_CURVE('',#14744,#14742,#2890,.T.);
#18641=EDGE_CURVE('',#14744,#14745,#9522,.T.);
#18642=EDGE_CURVE('',#14743,#14745,#2891,.T.);
#18643=EDGE_CURVE('',#14746,#14744,#9523,.T.);
#18644=EDGE_CURVE('',#14746,#14747,#9524,.T.);
#18645=EDGE_CURVE('',#14745,#14747,#9525,.T.);
#18646=EDGE_CURVE('',#14748,#14746,#2892,.T.);
#18647=EDGE_CURVE('',#14748,#14749,#9526,.T.);
#18648=EDGE_CURVE('',#14747,#14749,#2893,.T.);
#18649=EDGE_CURVE('',#14750,#14748,#9527,.T.);
#18650=EDGE_CURVE('',#14750,#14751,#9528,.T.);
#18651=EDGE_CURVE('',#14749,#14751,#9529,.T.);
#18652=EDGE_CURVE('',#14752,#14750,#2894,.T.);
#18653=EDGE_CURVE('',#14752,#14753,#9530,.T.);
#18654=EDGE_CURVE('',#14751,#14753,#2895,.T.);
#18655=EDGE_CURVE('',#14739,#14752,#9531,.T.);
#18656=EDGE_CURVE('',#14753,#14741,#9532,.T.);
#18657=EDGE_CURVE('',#14754,#14755,#2896,.T.);
#18658=EDGE_CURVE('',#14754,#14756,#9533,.T.);
#18659=EDGE_CURVE('',#14757,#14756,#2897,.T.);
#18660=EDGE_CURVE('',#14755,#14757,#9534,.T.);
#18661=EDGE_CURVE('',#14755,#14758,#9535,.T.);
#18662=EDGE_CURVE('',#14759,#14757,#9536,.T.);
#18663=EDGE_CURVE('',#14758,#14759,#9537,.T.);
#18664=EDGE_CURVE('',#14758,#14760,#2898,.T.);
#18665=EDGE_CURVE('',#14761,#14759,#2899,.T.);
#18666=EDGE_CURVE('',#14760,#14761,#9538,.T.);
#18667=EDGE_CURVE('',#14760,#14762,#9539,.T.);
#18668=EDGE_CURVE('',#14763,#14761,#9540,.T.);
#18669=EDGE_CURVE('',#14762,#14763,#9541,.T.);
#18670=EDGE_CURVE('',#14762,#14764,#2900,.T.);
#18671=EDGE_CURVE('',#14765,#14763,#2901,.T.);
#18672=EDGE_CURVE('',#14764,#14765,#9542,.T.);
#18673=EDGE_CURVE('',#14764,#14766,#9543,.T.);
#18674=EDGE_CURVE('',#14767,#14765,#9544,.T.);
#18675=EDGE_CURVE('',#14766,#14767,#9545,.T.);
#18676=EDGE_CURVE('',#14766,#14768,#2902,.T.);
#18677=EDGE_CURVE('',#14769,#14767,#2903,.T.);
#18678=EDGE_CURVE('',#14768,#14769,#9546,.T.);
#18679=EDGE_CURVE('',#14768,#14754,#9547,.T.);
#18680=EDGE_CURVE('',#14756,#14769,#9548,.T.);
#18681=EDGE_CURVE('',#14770,#14771,#2904,.T.);
#18682=EDGE_CURVE('',#14770,#14772,#9549,.T.);
#18683=EDGE_CURVE('',#14773,#14772,#2905,.T.);
#18684=EDGE_CURVE('',#14771,#14773,#9550,.T.);
#18685=EDGE_CURVE('',#14774,#14770,#9551,.T.);
#18686=EDGE_CURVE('',#14774,#14775,#9552,.T.);
#18687=EDGE_CURVE('',#14772,#14775,#9553,.T.);
#18688=EDGE_CURVE('',#14776,#14774,#2906,.T.);
#18689=EDGE_CURVE('',#14776,#14777,#9554,.T.);
#18690=EDGE_CURVE('',#14775,#14777,#2907,.T.);
#18691=EDGE_CURVE('',#14778,#14776,#9555,.T.);
#18692=EDGE_CURVE('',#14778,#14779,#9556,.T.);
#18693=EDGE_CURVE('',#14777,#14779,#9557,.T.);
#18694=EDGE_CURVE('',#14780,#14778,#2908,.T.);
#18695=EDGE_CURVE('',#14780,#14781,#9558,.T.);
#18696=EDGE_CURVE('',#14779,#14781,#2909,.T.);
#18697=EDGE_CURVE('',#14782,#14780,#9559,.T.);
#18698=EDGE_CURVE('',#14782,#14783,#9560,.T.);
#18699=EDGE_CURVE('',#14781,#14783,#9561,.T.);
#18700=EDGE_CURVE('',#14784,#14782,#2910,.T.);
#18701=EDGE_CURVE('',#14784,#14785,#9562,.T.);
#18702=EDGE_CURVE('',#14783,#14785,#2911,.T.);
#18703=EDGE_CURVE('',#14771,#14784,#9563,.T.);
#18704=EDGE_CURVE('',#14785,#14773,#9564,.T.);
#18705=EDGE_CURVE('',#14786,#14787,#2912,.T.);
#18706=EDGE_CURVE('',#14786,#14788,#9565,.T.);
#18707=EDGE_CURVE('',#14789,#14788,#2913,.T.);
#18708=EDGE_CURVE('',#14787,#14789,#9566,.T.);
#18709=EDGE_CURVE('',#14787,#14790,#9567,.T.);
#18710=EDGE_CURVE('',#14791,#14789,#9568,.T.);
#18711=EDGE_CURVE('',#14790,#14791,#9569,.T.);
#18712=EDGE_CURVE('',#14790,#14792,#2914,.T.);
#18713=EDGE_CURVE('',#14793,#14791,#2915,.T.);
#18714=EDGE_CURVE('',#14792,#14793,#9570,.T.);
#18715=EDGE_CURVE('',#14792,#14794,#9571,.T.);
#18716=EDGE_CURVE('',#14795,#14793,#9572,.T.);
#18717=EDGE_CURVE('',#14794,#14795,#9573,.T.);
#18718=EDGE_CURVE('',#14794,#14796,#2916,.T.);
#18719=EDGE_CURVE('',#14797,#14795,#2917,.T.);
#18720=EDGE_CURVE('',#14796,#14797,#9574,.T.);
#18721=EDGE_CURVE('',#14796,#14798,#9575,.T.);
#18722=EDGE_CURVE('',#14799,#14797,#9576,.T.);
#18723=EDGE_CURVE('',#14798,#14799,#9577,.T.);
#18724=EDGE_CURVE('',#14798,#14800,#2918,.T.);
#18725=EDGE_CURVE('',#14801,#14799,#2919,.T.);
#18726=EDGE_CURVE('',#14800,#14801,#9578,.T.);
#18727=EDGE_CURVE('',#14800,#14786,#9579,.T.);
#18728=EDGE_CURVE('',#14788,#14801,#9580,.T.);
#24214=ORIENTED_EDGE('',*,*,#18009,.T.);
#24215=ORIENTED_EDGE('',*,*,#18010,.F.);
#24216=ORIENTED_EDGE('',*,*,#18011,.F.);
#24217=ORIENTED_EDGE('',*,*,#18012,.T.);
#24218=ORIENTED_EDGE('',*,*,#18013,.T.);
#24219=ORIENTED_EDGE('',*,*,#18014,.F.);
#24220=ORIENTED_EDGE('',*,*,#18015,.F.);
#24221=ORIENTED_EDGE('',*,*,#18010,.T.);
#24222=ORIENTED_EDGE('',*,*,#18016,.T.);
#24223=ORIENTED_EDGE('',*,*,#18017,.F.);
#24224=ORIENTED_EDGE('',*,*,#18018,.F.);
#24225=ORIENTED_EDGE('',*,*,#18014,.T.);
#24226=ORIENTED_EDGE('',*,*,#18019,.T.);
#24227=ORIENTED_EDGE('',*,*,#18020,.F.);
#24228=ORIENTED_EDGE('',*,*,#18021,.F.);
#24229=ORIENTED_EDGE('',*,*,#18017,.T.);
#24230=ORIENTED_EDGE('',*,*,#18022,.T.);
#24231=ORIENTED_EDGE('',*,*,#18023,.F.);
#24232=ORIENTED_EDGE('',*,*,#18024,.F.);
#24233=ORIENTED_EDGE('',*,*,#18025,.T.);
#24234=ORIENTED_EDGE('',*,*,#18026,.T.);
#24235=ORIENTED_EDGE('',*,*,#18027,.F.);
#24236=ORIENTED_EDGE('',*,*,#18028,.F.);
#24237=ORIENTED_EDGE('',*,*,#18023,.T.);
#24238=ORIENTED_EDGE('',*,*,#18029,.T.);
#24239=ORIENTED_EDGE('',*,*,#18030,.F.);
#24240=ORIENTED_EDGE('',*,*,#18031,.F.);
#24241=ORIENTED_EDGE('',*,*,#18027,.T.);
#24242=ORIENTED_EDGE('',*,*,#18032,.T.);
#24243=ORIENTED_EDGE('',*,*,#18033,.F.);
#24244=ORIENTED_EDGE('',*,*,#18034,.F.);
#24245=ORIENTED_EDGE('',*,*,#18030,.T.);
#24246=ORIENTED_EDGE('',*,*,#18035,.T.);
#24247=ORIENTED_EDGE('',*,*,#18036,.F.);
#24248=ORIENTED_EDGE('',*,*,#18037,.F.);
#24249=ORIENTED_EDGE('',*,*,#18020,.T.);
#24250=ORIENTED_EDGE('',*,*,#18038,.T.);
#24251=ORIENTED_EDGE('',*,*,#18012,.F.);
#24252=ORIENTED_EDGE('',*,*,#18039,.F.);
#24253=ORIENTED_EDGE('',*,*,#18040,.T.);
#24254=ORIENTED_EDGE('',*,*,#18041,.T.);
#24255=ORIENTED_EDGE('',*,*,#18040,.F.);
#24256=ORIENTED_EDGE('',*,*,#18042,.F.);
#24257=ORIENTED_EDGE('',*,*,#18043,.T.);
#24258=ORIENTED_EDGE('',*,*,#18044,.T.);
#24259=ORIENTED_EDGE('',*,*,#18043,.F.);
#24260=ORIENTED_EDGE('',*,*,#18045,.F.);
#24261=ORIENTED_EDGE('',*,*,#18036,.T.);
#24262=ORIENTED_EDGE('',*,*,#18046,.T.);
#24263=ORIENTED_EDGE('',*,*,#18047,.F.);
#24264=ORIENTED_EDGE('',*,*,#18048,.F.);
#24265=ORIENTED_EDGE('',*,*,#18033,.T.);
#24266=ORIENTED_EDGE('',*,*,#18049,.T.);
#24267=ORIENTED_EDGE('',*,*,#18050,.F.);
#24268=ORIENTED_EDGE('',*,*,#18051,.F.);
#24269=ORIENTED_EDGE('',*,*,#18047,.T.);
#24270=ORIENTED_EDGE('',*,*,#18052,.T.);
#24271=ORIENTED_EDGE('',*,*,#18053,.F.);
#24272=ORIENTED_EDGE('',*,*,#18054,.F.);
#24273=ORIENTED_EDGE('',*,*,#18050,.T.);
#24274=ORIENTED_EDGE('',*,*,#18055,.T.);
#24275=ORIENTED_EDGE('',*,*,#18025,.F.);
#24276=ORIENTED_EDGE('',*,*,#18056,.F.);
#24277=ORIENTED_EDGE('',*,*,#18053,.T.);
#24278=ORIENTED_EDGE('',*,*,#18048,.T.);
#24279=ORIENTED_EDGE('',*,*,#18051,.T.);
#24280=ORIENTED_EDGE('',*,*,#18054,.T.);
#24281=ORIENTED_EDGE('',*,*,#18056,.T.);
#24282=ORIENTED_EDGE('',*,*,#18024,.T.);
#24283=ORIENTED_EDGE('',*,*,#18028,.T.);
#24284=ORIENTED_EDGE('',*,*,#18031,.T.);
#24285=ORIENTED_EDGE('',*,*,#18034,.T.);
#24286=ORIENTED_EDGE('',*,*,#18037,.T.);
#24287=ORIENTED_EDGE('',*,*,#18045,.T.);
#24288=ORIENTED_EDGE('',*,*,#18042,.T.);
#24289=ORIENTED_EDGE('',*,*,#18039,.T.);
#24290=ORIENTED_EDGE('',*,*,#18011,.T.);
#24291=ORIENTED_EDGE('',*,*,#18015,.T.);
#24292=ORIENTED_EDGE('',*,*,#18018,.T.);
#24293=ORIENTED_EDGE('',*,*,#18021,.T.);
#24294=ORIENTED_EDGE('',*,*,#18046,.F.);
#24295=ORIENTED_EDGE('',*,*,#18032,.F.);
#24296=ORIENTED_EDGE('',*,*,#18029,.F.);
#24297=ORIENTED_EDGE('',*,*,#18026,.F.);
#24298=ORIENTED_EDGE('',*,*,#18022,.F.);
#24299=ORIENTED_EDGE('',*,*,#18055,.F.);
#24300=ORIENTED_EDGE('',*,*,#18052,.F.);
#24301=ORIENTED_EDGE('',*,*,#18049,.F.);
#24302=ORIENTED_EDGE('',*,*,#18035,.F.);
#24303=ORIENTED_EDGE('',*,*,#18019,.F.);
#24304=ORIENTED_EDGE('',*,*,#18016,.F.);
#24305=ORIENTED_EDGE('',*,*,#18013,.F.);
#24306=ORIENTED_EDGE('',*,*,#18009,.F.);
#24307=ORIENTED_EDGE('',*,*,#18038,.F.);
#24308=ORIENTED_EDGE('',*,*,#18041,.F.);
#24309=ORIENTED_EDGE('',*,*,#18044,.F.);
#24310=ORIENTED_EDGE('',*,*,#18057,.T.);
#24311=ORIENTED_EDGE('',*,*,#18058,.F.);
#24312=ORIENTED_EDGE('',*,*,#18059,.F.);
#24313=ORIENTED_EDGE('',*,*,#18060,.T.);
#24314=ORIENTED_EDGE('',*,*,#18061,.T.);
#24315=ORIENTED_EDGE('',*,*,#18062,.F.);
#24316=ORIENTED_EDGE('',*,*,#18063,.F.);
#24317=ORIENTED_EDGE('',*,*,#18058,.T.);
#24318=ORIENTED_EDGE('',*,*,#18064,.T.);
#24319=ORIENTED_EDGE('',*,*,#18065,.F.);
#24320=ORIENTED_EDGE('',*,*,#18066,.F.);
#24321=ORIENTED_EDGE('',*,*,#18062,.T.);
#24322=ORIENTED_EDGE('',*,*,#18067,.T.);
#24323=ORIENTED_EDGE('',*,*,#18068,.F.);
#24324=ORIENTED_EDGE('',*,*,#18069,.F.);
#24325=ORIENTED_EDGE('',*,*,#18065,.T.);
#24326=ORIENTED_EDGE('',*,*,#18070,.T.);
#24327=ORIENTED_EDGE('',*,*,#18071,.F.);
#24328=ORIENTED_EDGE('',*,*,#18072,.F.);
#24329=ORIENTED_EDGE('',*,*,#18073,.T.);
#24330=ORIENTED_EDGE('',*,*,#18074,.T.);
#24331=ORIENTED_EDGE('',*,*,#18075,.F.);
#24332=ORIENTED_EDGE('',*,*,#18076,.F.);
#24333=ORIENTED_EDGE('',*,*,#18071,.T.);
#24334=ORIENTED_EDGE('',*,*,#18077,.T.);
#24335=ORIENTED_EDGE('',*,*,#18078,.F.);
#24336=ORIENTED_EDGE('',*,*,#18079,.F.);
#24337=ORIENTED_EDGE('',*,*,#18075,.T.);
#24338=ORIENTED_EDGE('',*,*,#18080,.T.);
#24339=ORIENTED_EDGE('',*,*,#18081,.F.);
#24340=ORIENTED_EDGE('',*,*,#18082,.F.);
#24341=ORIENTED_EDGE('',*,*,#18078,.T.);
#24342=ORIENTED_EDGE('',*,*,#18083,.T.);
#24343=ORIENTED_EDGE('',*,*,#18084,.F.);
#24344=ORIENTED_EDGE('',*,*,#18085,.F.);
#24345=ORIENTED_EDGE('',*,*,#18068,.T.);
#24346=ORIENTED_EDGE('',*,*,#18086,.T.);
#24347=ORIENTED_EDGE('',*,*,#18060,.F.);
#24348=ORIENTED_EDGE('',*,*,#18087,.F.);
#24349=ORIENTED_EDGE('',*,*,#18088,.T.);
#24350=ORIENTED_EDGE('',*,*,#18089,.T.);
#24351=ORIENTED_EDGE('',*,*,#18088,.F.);
#24352=ORIENTED_EDGE('',*,*,#18090,.F.);
#24353=ORIENTED_EDGE('',*,*,#18091,.T.);
#24354=ORIENTED_EDGE('',*,*,#18092,.T.);
#24355=ORIENTED_EDGE('',*,*,#18091,.F.);
#24356=ORIENTED_EDGE('',*,*,#18093,.F.);
#24357=ORIENTED_EDGE('',*,*,#18084,.T.);
#24358=ORIENTED_EDGE('',*,*,#18094,.T.);
#24359=ORIENTED_EDGE('',*,*,#18095,.F.);
#24360=ORIENTED_EDGE('',*,*,#18096,.F.);
#24361=ORIENTED_EDGE('',*,*,#18081,.T.);
#24362=ORIENTED_EDGE('',*,*,#18097,.T.);
#24363=ORIENTED_EDGE('',*,*,#18098,.F.);
#24364=ORIENTED_EDGE('',*,*,#18099,.F.);
#24365=ORIENTED_EDGE('',*,*,#18095,.T.);
#24366=ORIENTED_EDGE('',*,*,#18100,.T.);
#24367=ORIENTED_EDGE('',*,*,#18101,.F.);
#24368=ORIENTED_EDGE('',*,*,#18102,.F.);
#24369=ORIENTED_EDGE('',*,*,#18098,.T.);
#24370=ORIENTED_EDGE('',*,*,#18103,.T.);
#24371=ORIENTED_EDGE('',*,*,#18073,.F.);
#24372=ORIENTED_EDGE('',*,*,#18104,.F.);
#24373=ORIENTED_EDGE('',*,*,#18101,.T.);
#24374=ORIENTED_EDGE('',*,*,#18096,.T.);
#24375=ORIENTED_EDGE('',*,*,#18099,.T.);
#24376=ORIENTED_EDGE('',*,*,#18102,.T.);
#24377=ORIENTED_EDGE('',*,*,#18104,.T.);
#24378=ORIENTED_EDGE('',*,*,#18072,.T.);
#24379=ORIENTED_EDGE('',*,*,#18076,.T.);
#24380=ORIENTED_EDGE('',*,*,#18079,.T.);
#24381=ORIENTED_EDGE('',*,*,#18082,.T.);
#24382=ORIENTED_EDGE('',*,*,#18085,.T.);
#24383=ORIENTED_EDGE('',*,*,#18093,.T.);
#24384=ORIENTED_EDGE('',*,*,#18090,.T.);
#24385=ORIENTED_EDGE('',*,*,#18087,.T.);
#24386=ORIENTED_EDGE('',*,*,#18059,.T.);
#24387=ORIENTED_EDGE('',*,*,#18063,.T.);
#24388=ORIENTED_EDGE('',*,*,#18066,.T.);
#24389=ORIENTED_EDGE('',*,*,#18069,.T.);
#24390=ORIENTED_EDGE('',*,*,#18094,.F.);
#24391=ORIENTED_EDGE('',*,*,#18080,.F.);
#24392=ORIENTED_EDGE('',*,*,#18077,.F.);
#24393=ORIENTED_EDGE('',*,*,#18074,.F.);
#24394=ORIENTED_EDGE('',*,*,#18070,.F.);
#24395=ORIENTED_EDGE('',*,*,#18103,.F.);
#24396=ORIENTED_EDGE('',*,*,#18100,.F.);
#24397=ORIENTED_EDGE('',*,*,#18097,.F.);
#24398=ORIENTED_EDGE('',*,*,#18083,.F.);
#24399=ORIENTED_EDGE('',*,*,#18067,.F.);
#24400=ORIENTED_EDGE('',*,*,#18064,.F.);
#24401=ORIENTED_EDGE('',*,*,#18061,.F.);
#24402=ORIENTED_EDGE('',*,*,#18057,.F.);
#24403=ORIENTED_EDGE('',*,*,#18086,.F.);
#24404=ORIENTED_EDGE('',*,*,#18089,.F.);
#24405=ORIENTED_EDGE('',*,*,#18092,.F.);
#24406=ORIENTED_EDGE('',*,*,#18105,.T.);
#24407=ORIENTED_EDGE('',*,*,#18106,.F.);
#24408=ORIENTED_EDGE('',*,*,#18107,.F.);
#24409=ORIENTED_EDGE('',*,*,#18108,.T.);
#24410=ORIENTED_EDGE('',*,*,#18109,.T.);
#24411=ORIENTED_EDGE('',*,*,#18110,.F.);
#24412=ORIENTED_EDGE('',*,*,#18111,.F.);
#24413=ORIENTED_EDGE('',*,*,#18106,.T.);
#24414=ORIENTED_EDGE('',*,*,#18112,.T.);
#24415=ORIENTED_EDGE('',*,*,#18113,.F.);
#24416=ORIENTED_EDGE('',*,*,#18114,.F.);
#24417=ORIENTED_EDGE('',*,*,#18110,.T.);
#24418=ORIENTED_EDGE('',*,*,#18115,.T.);
#24419=ORIENTED_EDGE('',*,*,#18116,.F.);
#24420=ORIENTED_EDGE('',*,*,#18117,.F.);
#24421=ORIENTED_EDGE('',*,*,#18113,.T.);
#24422=ORIENTED_EDGE('',*,*,#18118,.T.);
#24423=ORIENTED_EDGE('',*,*,#18119,.F.);
#24424=ORIENTED_EDGE('',*,*,#18120,.F.);
#24425=ORIENTED_EDGE('',*,*,#18121,.T.);
#24426=ORIENTED_EDGE('',*,*,#18122,.T.);
#24427=ORIENTED_EDGE('',*,*,#18123,.F.);
#24428=ORIENTED_EDGE('',*,*,#18124,.F.);
#24429=ORIENTED_EDGE('',*,*,#18119,.T.);
#24430=ORIENTED_EDGE('',*,*,#18125,.T.);
#24431=ORIENTED_EDGE('',*,*,#18126,.F.);
#24432=ORIENTED_EDGE('',*,*,#18127,.F.);
#24433=ORIENTED_EDGE('',*,*,#18123,.T.);
#24434=ORIENTED_EDGE('',*,*,#18128,.T.);
#24435=ORIENTED_EDGE('',*,*,#18129,.F.);
#24436=ORIENTED_EDGE('',*,*,#18130,.F.);
#24437=ORIENTED_EDGE('',*,*,#18126,.T.);
#24438=ORIENTED_EDGE('',*,*,#18131,.T.);
#24439=ORIENTED_EDGE('',*,*,#18132,.F.);
#24440=ORIENTED_EDGE('',*,*,#18133,.F.);
#24441=ORIENTED_EDGE('',*,*,#18116,.T.);
#24442=ORIENTED_EDGE('',*,*,#18134,.T.);
#24443=ORIENTED_EDGE('',*,*,#18108,.F.);
#24444=ORIENTED_EDGE('',*,*,#18135,.F.);
#24445=ORIENTED_EDGE('',*,*,#18136,.T.);
#24446=ORIENTED_EDGE('',*,*,#18137,.T.);
#24447=ORIENTED_EDGE('',*,*,#18136,.F.);
#24448=ORIENTED_EDGE('',*,*,#18138,.F.);
#24449=ORIENTED_EDGE('',*,*,#18139,.T.);
#24450=ORIENTED_EDGE('',*,*,#18140,.T.);
#24451=ORIENTED_EDGE('',*,*,#18139,.F.);
#24452=ORIENTED_EDGE('',*,*,#18141,.F.);
#24453=ORIENTED_EDGE('',*,*,#18132,.T.);
#24454=ORIENTED_EDGE('',*,*,#18142,.T.);
#24455=ORIENTED_EDGE('',*,*,#18143,.F.);
#24456=ORIENTED_EDGE('',*,*,#18144,.F.);
#24457=ORIENTED_EDGE('',*,*,#18129,.T.);
#24458=ORIENTED_EDGE('',*,*,#18145,.T.);
#24459=ORIENTED_EDGE('',*,*,#18146,.F.);
#24460=ORIENTED_EDGE('',*,*,#18147,.F.);
#24461=ORIENTED_EDGE('',*,*,#18143,.T.);
#24462=ORIENTED_EDGE('',*,*,#18148,.T.);
#24463=ORIENTED_EDGE('',*,*,#18149,.F.);
#24464=ORIENTED_EDGE('',*,*,#18150,.F.);
#24465=ORIENTED_EDGE('',*,*,#18146,.T.);
#24466=ORIENTED_EDGE('',*,*,#18151,.T.);
#24467=ORIENTED_EDGE('',*,*,#18121,.F.);
#24468=ORIENTED_EDGE('',*,*,#18152,.F.);
#24469=ORIENTED_EDGE('',*,*,#18149,.T.);
#24470=ORIENTED_EDGE('',*,*,#18144,.T.);
#24471=ORIENTED_EDGE('',*,*,#18147,.T.);
#24472=ORIENTED_EDGE('',*,*,#18150,.T.);
#24473=ORIENTED_EDGE('',*,*,#18152,.T.);
#24474=ORIENTED_EDGE('',*,*,#18120,.T.);
#24475=ORIENTED_EDGE('',*,*,#18124,.T.);
#24476=ORIENTED_EDGE('',*,*,#18127,.T.);
#24477=ORIENTED_EDGE('',*,*,#18130,.T.);
#24478=ORIENTED_EDGE('',*,*,#18133,.T.);
#24479=ORIENTED_EDGE('',*,*,#18141,.T.);
#24480=ORIENTED_EDGE('',*,*,#18138,.T.);
#24481=ORIENTED_EDGE('',*,*,#18135,.T.);
#24482=ORIENTED_EDGE('',*,*,#18107,.T.);
#24483=ORIENTED_EDGE('',*,*,#18111,.T.);
#24484=ORIENTED_EDGE('',*,*,#18114,.T.);
#24485=ORIENTED_EDGE('',*,*,#18117,.T.);
#24486=ORIENTED_EDGE('',*,*,#18142,.F.);
#24487=ORIENTED_EDGE('',*,*,#18128,.F.);
#24488=ORIENTED_EDGE('',*,*,#18125,.F.);
#24489=ORIENTED_EDGE('',*,*,#18122,.F.);
#24490=ORIENTED_EDGE('',*,*,#18118,.F.);
#24491=ORIENTED_EDGE('',*,*,#18151,.F.);
#24492=ORIENTED_EDGE('',*,*,#18148,.F.);
#24493=ORIENTED_EDGE('',*,*,#18145,.F.);
#24494=ORIENTED_EDGE('',*,*,#18131,.F.);
#24495=ORIENTED_EDGE('',*,*,#18115,.F.);
#24496=ORIENTED_EDGE('',*,*,#18112,.F.);
#24497=ORIENTED_EDGE('',*,*,#18109,.F.);
#24498=ORIENTED_EDGE('',*,*,#18105,.F.);
#24499=ORIENTED_EDGE('',*,*,#18134,.F.);
#24500=ORIENTED_EDGE('',*,*,#18137,.F.);
#24501=ORIENTED_EDGE('',*,*,#18140,.F.);
#24502=ORIENTED_EDGE('',*,*,#18153,.T.);
#24503=ORIENTED_EDGE('',*,*,#18154,.F.);
#24504=ORIENTED_EDGE('',*,*,#18155,.F.);
#24505=ORIENTED_EDGE('',*,*,#18156,.T.);
#24506=ORIENTED_EDGE('',*,*,#18157,.T.);
#24507=ORIENTED_EDGE('',*,*,#18158,.F.);
#24508=ORIENTED_EDGE('',*,*,#18159,.F.);
#24509=ORIENTED_EDGE('',*,*,#18154,.T.);
#24510=ORIENTED_EDGE('',*,*,#18160,.T.);
#24511=ORIENTED_EDGE('',*,*,#18161,.F.);
#24512=ORIENTED_EDGE('',*,*,#18162,.F.);
#24513=ORIENTED_EDGE('',*,*,#18158,.T.);
#24514=ORIENTED_EDGE('',*,*,#18163,.T.);
#24515=ORIENTED_EDGE('',*,*,#18164,.F.);
#24516=ORIENTED_EDGE('',*,*,#18165,.F.);
#24517=ORIENTED_EDGE('',*,*,#18161,.T.);
#24518=ORIENTED_EDGE('',*,*,#18166,.T.);
#24519=ORIENTED_EDGE('',*,*,#18167,.F.);
#24520=ORIENTED_EDGE('',*,*,#18168,.F.);
#24521=ORIENTED_EDGE('',*,*,#18169,.T.);
#24522=ORIENTED_EDGE('',*,*,#18170,.T.);
#24523=ORIENTED_EDGE('',*,*,#18171,.F.);
#24524=ORIENTED_EDGE('',*,*,#18172,.F.);
#24525=ORIENTED_EDGE('',*,*,#18167,.T.);
#24526=ORIENTED_EDGE('',*,*,#18173,.T.);
#24527=ORIENTED_EDGE('',*,*,#18174,.F.);
#24528=ORIENTED_EDGE('',*,*,#18175,.F.);
#24529=ORIENTED_EDGE('',*,*,#18171,.T.);
#24530=ORIENTED_EDGE('',*,*,#18176,.T.);
#24531=ORIENTED_EDGE('',*,*,#18177,.F.);
#24532=ORIENTED_EDGE('',*,*,#18178,.F.);
#24533=ORIENTED_EDGE('',*,*,#18174,.T.);
#24534=ORIENTED_EDGE('',*,*,#18179,.T.);
#24535=ORIENTED_EDGE('',*,*,#18180,.F.);
#24536=ORIENTED_EDGE('',*,*,#18181,.F.);
#24537=ORIENTED_EDGE('',*,*,#18164,.T.);
#24538=ORIENTED_EDGE('',*,*,#18182,.T.);
#24539=ORIENTED_EDGE('',*,*,#18156,.F.);
#24540=ORIENTED_EDGE('',*,*,#18183,.F.);
#24541=ORIENTED_EDGE('',*,*,#18184,.T.);
#24542=ORIENTED_EDGE('',*,*,#18185,.T.);
#24543=ORIENTED_EDGE('',*,*,#18184,.F.);
#24544=ORIENTED_EDGE('',*,*,#18186,.F.);
#24545=ORIENTED_EDGE('',*,*,#18187,.T.);
#24546=ORIENTED_EDGE('',*,*,#18188,.T.);
#24547=ORIENTED_EDGE('',*,*,#18187,.F.);
#24548=ORIENTED_EDGE('',*,*,#18189,.F.);
#24549=ORIENTED_EDGE('',*,*,#18180,.T.);
#24550=ORIENTED_EDGE('',*,*,#18190,.T.);
#24551=ORIENTED_EDGE('',*,*,#18191,.F.);
#24552=ORIENTED_EDGE('',*,*,#18192,.F.);
#24553=ORIENTED_EDGE('',*,*,#18177,.T.);
#24554=ORIENTED_EDGE('',*,*,#18193,.T.);
#24555=ORIENTED_EDGE('',*,*,#18194,.F.);
#24556=ORIENTED_EDGE('',*,*,#18195,.F.);
#24557=ORIENTED_EDGE('',*,*,#18191,.T.);
#24558=ORIENTED_EDGE('',*,*,#18196,.T.);
#24559=ORIENTED_EDGE('',*,*,#18197,.F.);
#24560=ORIENTED_EDGE('',*,*,#18198,.F.);
#24561=ORIENTED_EDGE('',*,*,#18194,.T.);
#24562=ORIENTED_EDGE('',*,*,#18199,.T.);
#24563=ORIENTED_EDGE('',*,*,#18169,.F.);
#24564=ORIENTED_EDGE('',*,*,#18200,.F.);
#24565=ORIENTED_EDGE('',*,*,#18197,.T.);
#24566=ORIENTED_EDGE('',*,*,#18192,.T.);
#24567=ORIENTED_EDGE('',*,*,#18195,.T.);
#24568=ORIENTED_EDGE('',*,*,#18198,.T.);
#24569=ORIENTED_EDGE('',*,*,#18200,.T.);
#24570=ORIENTED_EDGE('',*,*,#18168,.T.);
#24571=ORIENTED_EDGE('',*,*,#18172,.T.);
#24572=ORIENTED_EDGE('',*,*,#18175,.T.);
#24573=ORIENTED_EDGE('',*,*,#18178,.T.);
#24574=ORIENTED_EDGE('',*,*,#18181,.T.);
#24575=ORIENTED_EDGE('',*,*,#18189,.T.);
#24576=ORIENTED_EDGE('',*,*,#18186,.T.);
#24577=ORIENTED_EDGE('',*,*,#18183,.T.);
#24578=ORIENTED_EDGE('',*,*,#18155,.T.);
#24579=ORIENTED_EDGE('',*,*,#18159,.T.);
#24580=ORIENTED_EDGE('',*,*,#18162,.T.);
#24581=ORIENTED_EDGE('',*,*,#18165,.T.);
#24582=ORIENTED_EDGE('',*,*,#18190,.F.);
#24583=ORIENTED_EDGE('',*,*,#18176,.F.);
#24584=ORIENTED_EDGE('',*,*,#18173,.F.);
#24585=ORIENTED_EDGE('',*,*,#18170,.F.);
#24586=ORIENTED_EDGE('',*,*,#18166,.F.);
#24587=ORIENTED_EDGE('',*,*,#18199,.F.);
#24588=ORIENTED_EDGE('',*,*,#18196,.F.);
#24589=ORIENTED_EDGE('',*,*,#18193,.F.);
#24590=ORIENTED_EDGE('',*,*,#18179,.F.);
#24591=ORIENTED_EDGE('',*,*,#18163,.F.);
#24592=ORIENTED_EDGE('',*,*,#18160,.F.);
#24593=ORIENTED_EDGE('',*,*,#18157,.F.);
#24594=ORIENTED_EDGE('',*,*,#18153,.F.);
#24595=ORIENTED_EDGE('',*,*,#18182,.F.);
#24596=ORIENTED_EDGE('',*,*,#18185,.F.);
#24597=ORIENTED_EDGE('',*,*,#18188,.F.);
#24598=ORIENTED_EDGE('',*,*,#18201,.F.);
#24599=ORIENTED_EDGE('',*,*,#18202,.F.);
#24600=ORIENTED_EDGE('',*,*,#18203,.F.);
#24601=ORIENTED_EDGE('',*,*,#18204,.T.);
#24602=ORIENTED_EDGE('',*,*,#18205,.F.);
#24603=ORIENTED_EDGE('',*,*,#18206,.F.);
#24604=ORIENTED_EDGE('',*,*,#18207,.F.);
#24605=ORIENTED_EDGE('',*,*,#18208,.F.);
#24606=ORIENTED_EDGE('',*,*,#18209,.F.);
#24607=ORIENTED_EDGE('',*,*,#18210,.F.);
#24608=ORIENTED_EDGE('',*,*,#18211,.F.);
#24609=ORIENTED_EDGE('',*,*,#18212,.F.);
#24610=ORIENTED_EDGE('',*,*,#18213,.F.);
#24611=ORIENTED_EDGE('',*,*,#18214,.F.);
#24612=ORIENTED_EDGE('',*,*,#18215,.F.);
#24613=ORIENTED_EDGE('',*,*,#18216,.F.);
#24614=ORIENTED_EDGE('',*,*,#18213,.T.);
#24615=ORIENTED_EDGE('',*,*,#18217,.T.);
#24616=ORIENTED_EDGE('',*,*,#18218,.T.);
#24617=ORIENTED_EDGE('',*,*,#18219,.F.);
#24618=ORIENTED_EDGE('',*,*,#18212,.T.);
#24619=ORIENTED_EDGE('',*,*,#18220,.T.);
#24620=ORIENTED_EDGE('',*,*,#18221,.T.);
#24621=ORIENTED_EDGE('',*,*,#18217,.F.);
#24622=ORIENTED_EDGE('',*,*,#18211,.T.);
#24623=ORIENTED_EDGE('',*,*,#18222,.T.);
#24624=ORIENTED_EDGE('',*,*,#18223,.T.);
#24625=ORIENTED_EDGE('',*,*,#18220,.F.);
#24626=ORIENTED_EDGE('',*,*,#18210,.T.);
#24627=ORIENTED_EDGE('',*,*,#18224,.T.);
#24628=ORIENTED_EDGE('',*,*,#18225,.T.);
#24629=ORIENTED_EDGE('',*,*,#18222,.F.);
#24630=ORIENTED_EDGE('',*,*,#18205,.T.);
#24631=ORIENTED_EDGE('',*,*,#18226,.T.);
#24632=ORIENTED_EDGE('',*,*,#18227,.T.);
#24633=ORIENTED_EDGE('',*,*,#18228,.F.);
#24634=ORIENTED_EDGE('',*,*,#18203,.T.);
#24635=ORIENTED_EDGE('',*,*,#18229,.T.);
#24636=ORIENTED_EDGE('',*,*,#18230,.T.);
#24637=ORIENTED_EDGE('',*,*,#18231,.F.);
#24638=ORIENTED_EDGE('',*,*,#18202,.T.);
#24639=ORIENTED_EDGE('',*,*,#18232,.T.);
#24640=ORIENTED_EDGE('',*,*,#18233,.T.);
#24641=ORIENTED_EDGE('',*,*,#18229,.F.);
#24642=ORIENTED_EDGE('',*,*,#18234,.F.);
#24643=ORIENTED_EDGE('',*,*,#18230,.F.);
#24644=ORIENTED_EDGE('',*,*,#18233,.F.);
#24645=ORIENTED_EDGE('',*,*,#18235,.F.);
#24646=ORIENTED_EDGE('',*,*,#18236,.F.);
#24647=ORIENTED_EDGE('',*,*,#18237,.F.);
#24648=ORIENTED_EDGE('',*,*,#18238,.F.);
#24649=ORIENTED_EDGE('',*,*,#18227,.F.);
#24650=ORIENTED_EDGE('',*,*,#18218,.F.);
#24651=ORIENTED_EDGE('',*,*,#18221,.F.);
#24652=ORIENTED_EDGE('',*,*,#18223,.F.);
#24653=ORIENTED_EDGE('',*,*,#18225,.F.);
#24654=ORIENTED_EDGE('',*,*,#18239,.F.);
#24655=ORIENTED_EDGE('',*,*,#18240,.F.);
#24656=ORIENTED_EDGE('',*,*,#18241,.F.);
#24657=ORIENTED_EDGE('',*,*,#18242,.F.);
#24658=ORIENTED_EDGE('',*,*,#18209,.T.);
#24659=ORIENTED_EDGE('',*,*,#18243,.T.);
#24660=ORIENTED_EDGE('',*,*,#18239,.T.);
#24661=ORIENTED_EDGE('',*,*,#18224,.F.);
#24662=ORIENTED_EDGE('',*,*,#18201,.T.);
#24663=ORIENTED_EDGE('',*,*,#18244,.T.);
#24664=ORIENTED_EDGE('',*,*,#18235,.T.);
#24665=ORIENTED_EDGE('',*,*,#18232,.F.);
#24666=ORIENTED_EDGE('',*,*,#18214,.T.);
#24667=ORIENTED_EDGE('',*,*,#18219,.T.);
#24668=ORIENTED_EDGE('',*,*,#18242,.T.);
#24669=ORIENTED_EDGE('',*,*,#18245,.F.);
#24670=ORIENTED_EDGE('',*,*,#18215,.T.);
#24671=ORIENTED_EDGE('',*,*,#18245,.T.);
#24672=ORIENTED_EDGE('',*,*,#18241,.T.);
#24673=ORIENTED_EDGE('',*,*,#18246,.F.);
#24674=ORIENTED_EDGE('',*,*,#18216,.T.);
#24675=ORIENTED_EDGE('',*,*,#18246,.T.);
#24676=ORIENTED_EDGE('',*,*,#18240,.T.);
#24677=ORIENTED_EDGE('',*,*,#18243,.F.);
#24678=ORIENTED_EDGE('',*,*,#18234,.T.);
#24679=ORIENTED_EDGE('',*,*,#18226,.F.);
#24680=ORIENTED_EDGE('',*,*,#18204,.F.);
#24681=ORIENTED_EDGE('',*,*,#18231,.T.);
#24682=ORIENTED_EDGE('',*,*,#18206,.T.);
#24683=ORIENTED_EDGE('',*,*,#18228,.T.);
#24684=ORIENTED_EDGE('',*,*,#18238,.T.);
#24685=ORIENTED_EDGE('',*,*,#18247,.F.);
#24686=ORIENTED_EDGE('',*,*,#18207,.T.);
#24687=ORIENTED_EDGE('',*,*,#18247,.T.);
#24688=ORIENTED_EDGE('',*,*,#18237,.T.);
#24689=ORIENTED_EDGE('',*,*,#18248,.F.);
#24690=ORIENTED_EDGE('',*,*,#18208,.T.);
#24691=ORIENTED_EDGE('',*,*,#18248,.T.);
#24692=ORIENTED_EDGE('',*,*,#18236,.T.);
#24693=ORIENTED_EDGE('',*,*,#18244,.F.);
#24694=ORIENTED_EDGE('',*,*,#18249,.F.);
#24695=ORIENTED_EDGE('',*,*,#18250,.F.);
#24696=ORIENTED_EDGE('',*,*,#18251,.F.);
#24697=ORIENTED_EDGE('',*,*,#18252,.F.);
#24698=ORIENTED_EDGE('',*,*,#18253,.F.);
#24699=ORIENTED_EDGE('',*,*,#18254,.F.);
#24700=ORIENTED_EDGE('',*,*,#18255,.F.);
#24701=ORIENTED_EDGE('',*,*,#18256,.T.);
#24702=ORIENTED_EDGE('',*,*,#18257,.F.);
#24703=ORIENTED_EDGE('',*,*,#18258,.F.);
#24704=ORIENTED_EDGE('',*,*,#18259,.F.);
#24705=ORIENTED_EDGE('',*,*,#18260,.F.);
#24706=ORIENTED_EDGE('',*,*,#18261,.F.);
#24707=ORIENTED_EDGE('',*,*,#18262,.F.);
#24708=ORIENTED_EDGE('',*,*,#18263,.F.);
#24709=ORIENTED_EDGE('',*,*,#18264,.F.);
#24710=ORIENTED_EDGE('',*,*,#18261,.T.);
#24711=ORIENTED_EDGE('',*,*,#18265,.T.);
#24712=ORIENTED_EDGE('',*,*,#18266,.T.);
#24713=ORIENTED_EDGE('',*,*,#18267,.F.);
#24714=ORIENTED_EDGE('',*,*,#18260,.T.);
#24715=ORIENTED_EDGE('',*,*,#18268,.T.);
#24716=ORIENTED_EDGE('',*,*,#18269,.T.);
#24717=ORIENTED_EDGE('',*,*,#18265,.F.);
#24718=ORIENTED_EDGE('',*,*,#18259,.T.);
#24719=ORIENTED_EDGE('',*,*,#18270,.T.);
#24720=ORIENTED_EDGE('',*,*,#18271,.T.);
#24721=ORIENTED_EDGE('',*,*,#18268,.F.);
#24722=ORIENTED_EDGE('',*,*,#18258,.T.);
#24723=ORIENTED_EDGE('',*,*,#18272,.T.);
#24724=ORIENTED_EDGE('',*,*,#18273,.T.);
#24725=ORIENTED_EDGE('',*,*,#18270,.F.);
#24726=ORIENTED_EDGE('',*,*,#18253,.T.);
#24727=ORIENTED_EDGE('',*,*,#18274,.T.);
#24728=ORIENTED_EDGE('',*,*,#18275,.T.);
#24729=ORIENTED_EDGE('',*,*,#18276,.F.);
#24730=ORIENTED_EDGE('',*,*,#18252,.T.);
#24731=ORIENTED_EDGE('',*,*,#18277,.T.);
#24732=ORIENTED_EDGE('',*,*,#18278,.T.);
#24733=ORIENTED_EDGE('',*,*,#18274,.F.);
#24734=ORIENTED_EDGE('',*,*,#18251,.T.);
#24735=ORIENTED_EDGE('',*,*,#18279,.T.);
#24736=ORIENTED_EDGE('',*,*,#18280,.T.);
#24737=ORIENTED_EDGE('',*,*,#18277,.F.);
#24738=ORIENTED_EDGE('',*,*,#18250,.T.);
#24739=ORIENTED_EDGE('',*,*,#18281,.T.);
#24740=ORIENTED_EDGE('',*,*,#18282,.T.);
#24741=ORIENTED_EDGE('',*,*,#18279,.F.);
#24742=ORIENTED_EDGE('',*,*,#18278,.F.);
#24743=ORIENTED_EDGE('',*,*,#18280,.F.);
#24744=ORIENTED_EDGE('',*,*,#18282,.F.);
#24745=ORIENTED_EDGE('',*,*,#18283,.F.);
#24746=ORIENTED_EDGE('',*,*,#18284,.F.);
#24747=ORIENTED_EDGE('',*,*,#18285,.F.);
#24748=ORIENTED_EDGE('',*,*,#18286,.F.);
#24749=ORIENTED_EDGE('',*,*,#18275,.F.);
#24750=ORIENTED_EDGE('',*,*,#18266,.F.);
#24751=ORIENTED_EDGE('',*,*,#18269,.F.);
#24752=ORIENTED_EDGE('',*,*,#18271,.F.);
#24753=ORIENTED_EDGE('',*,*,#18273,.F.);
#24754=ORIENTED_EDGE('',*,*,#18287,.F.);
#24755=ORIENTED_EDGE('',*,*,#18288,.F.);
#24756=ORIENTED_EDGE('',*,*,#18289,.F.);
#24757=ORIENTED_EDGE('',*,*,#18290,.F.);
#24758=ORIENTED_EDGE('',*,*,#18257,.T.);
#24759=ORIENTED_EDGE('',*,*,#18291,.T.);
#24760=ORIENTED_EDGE('',*,*,#18287,.T.);
#24761=ORIENTED_EDGE('',*,*,#18272,.F.);
#24762=ORIENTED_EDGE('',*,*,#18249,.T.);
#24763=ORIENTED_EDGE('',*,*,#18292,.T.);
#24764=ORIENTED_EDGE('',*,*,#18283,.T.);
#24765=ORIENTED_EDGE('',*,*,#18281,.F.);
#24766=ORIENTED_EDGE('',*,*,#18262,.T.);
#24767=ORIENTED_EDGE('',*,*,#18267,.T.);
#24768=ORIENTED_EDGE('',*,*,#18290,.T.);
#24769=ORIENTED_EDGE('',*,*,#18293,.F.);
#24770=ORIENTED_EDGE('',*,*,#18263,.T.);
#24771=ORIENTED_EDGE('',*,*,#18293,.T.);
#24772=ORIENTED_EDGE('',*,*,#18289,.T.);
#24773=ORIENTED_EDGE('',*,*,#18294,.F.);
#24774=ORIENTED_EDGE('',*,*,#18264,.T.);
#24775=ORIENTED_EDGE('',*,*,#18294,.T.);
#24776=ORIENTED_EDGE('',*,*,#18288,.T.);
#24777=ORIENTED_EDGE('',*,*,#18291,.F.);
#24778=ORIENTED_EDGE('',*,*,#18254,.T.);
#24779=ORIENTED_EDGE('',*,*,#18276,.T.);
#24780=ORIENTED_EDGE('',*,*,#18286,.T.);
#24781=ORIENTED_EDGE('',*,*,#18295,.F.);
#24782=ORIENTED_EDGE('',*,*,#18255,.T.);
#24783=ORIENTED_EDGE('',*,*,#18295,.T.);
#24784=ORIENTED_EDGE('',*,*,#18285,.T.);
#24785=ORIENTED_EDGE('',*,*,#18296,.F.);
#24786=ORIENTED_EDGE('',*,*,#18284,.T.);
#24787=ORIENTED_EDGE('',*,*,#18292,.F.);
#24788=ORIENTED_EDGE('',*,*,#18256,.F.);
#24789=ORIENTED_EDGE('',*,*,#18296,.T.);
#24790=ORIENTED_EDGE('',*,*,#18297,.F.);
#24791=ORIENTED_EDGE('',*,*,#18298,.F.);
#24792=ORIENTED_EDGE('',*,*,#18299,.F.);
#24793=ORIENTED_EDGE('',*,*,#18300,.F.);
#24794=ORIENTED_EDGE('',*,*,#18301,.F.);
#24795=ORIENTED_EDGE('',*,*,#18302,.F.);
#24796=ORIENTED_EDGE('',*,*,#18303,.F.);
#24797=ORIENTED_EDGE('',*,*,#18304,.F.);
#24798=ORIENTED_EDGE('',*,*,#18305,.F.);
#24799=ORIENTED_EDGE('',*,*,#18306,.F.);
#24800=ORIENTED_EDGE('',*,*,#18307,.F.);
#24801=ORIENTED_EDGE('',*,*,#18308,.F.);
#24802=ORIENTED_EDGE('',*,*,#18309,.F.);
#24803=ORIENTED_EDGE('',*,*,#18310,.F.);
#24804=ORIENTED_EDGE('',*,*,#18311,.F.);
#24805=ORIENTED_EDGE('',*,*,#18312,.F.);
#24806=ORIENTED_EDGE('',*,*,#18309,.T.);
#24807=ORIENTED_EDGE('',*,*,#18313,.T.);
#24808=ORIENTED_EDGE('',*,*,#18314,.T.);
#24809=ORIENTED_EDGE('',*,*,#18315,.F.);
#24810=ORIENTED_EDGE('',*,*,#18308,.T.);
#24811=ORIENTED_EDGE('',*,*,#18316,.T.);
#24812=ORIENTED_EDGE('',*,*,#18317,.T.);
#24813=ORIENTED_EDGE('',*,*,#18313,.F.);
#24814=ORIENTED_EDGE('',*,*,#18307,.T.);
#24815=ORIENTED_EDGE('',*,*,#18318,.T.);
#24816=ORIENTED_EDGE('',*,*,#18319,.T.);
#24817=ORIENTED_EDGE('',*,*,#18316,.F.);
#24818=ORIENTED_EDGE('',*,*,#18306,.T.);
#24819=ORIENTED_EDGE('',*,*,#18320,.T.);
#24820=ORIENTED_EDGE('',*,*,#18321,.T.);
#24821=ORIENTED_EDGE('',*,*,#18318,.F.);
#24822=ORIENTED_EDGE('',*,*,#18301,.T.);
#24823=ORIENTED_EDGE('',*,*,#18322,.T.);
#24824=ORIENTED_EDGE('',*,*,#18323,.T.);
#24825=ORIENTED_EDGE('',*,*,#18324,.F.);
#24826=ORIENTED_EDGE('',*,*,#18300,.T.);
#24827=ORIENTED_EDGE('',*,*,#18325,.T.);
#24828=ORIENTED_EDGE('',*,*,#18326,.T.);
#24829=ORIENTED_EDGE('',*,*,#18322,.F.);
#24830=ORIENTED_EDGE('',*,*,#18299,.T.);
#24831=ORIENTED_EDGE('',*,*,#18327,.F.);
#24832=ORIENTED_EDGE('',*,*,#18328,.T.);
#24833=ORIENTED_EDGE('',*,*,#18325,.F.);
#24834=ORIENTED_EDGE('',*,*,#18298,.T.);
#24835=ORIENTED_EDGE('',*,*,#18329,.T.);
#24836=ORIENTED_EDGE('',*,*,#18330,.T.);
#24837=ORIENTED_EDGE('',*,*,#18327,.T.);
#24838=ORIENTED_EDGE('',*,*,#18323,.F.);
#24839=ORIENTED_EDGE('',*,*,#18326,.F.);
#24840=ORIENTED_EDGE('',*,*,#18328,.F.);
#24841=ORIENTED_EDGE('',*,*,#18330,.F.);
#24842=ORIENTED_EDGE('',*,*,#18331,.F.);
#24843=ORIENTED_EDGE('',*,*,#18332,.F.);
#24844=ORIENTED_EDGE('',*,*,#18333,.T.);
#24845=ORIENTED_EDGE('',*,*,#18334,.F.);
#24846=ORIENTED_EDGE('',*,*,#18314,.F.);
#24847=ORIENTED_EDGE('',*,*,#18317,.F.);
#24848=ORIENTED_EDGE('',*,*,#18319,.F.);
#24849=ORIENTED_EDGE('',*,*,#18321,.F.);
#24850=ORIENTED_EDGE('',*,*,#18335,.F.);
#24851=ORIENTED_EDGE('',*,*,#18336,.F.);
#24852=ORIENTED_EDGE('',*,*,#18337,.F.);
#24853=ORIENTED_EDGE('',*,*,#18338,.F.);
#24854=ORIENTED_EDGE('',*,*,#18305,.T.);
#24855=ORIENTED_EDGE('',*,*,#18339,.T.);
#24856=ORIENTED_EDGE('',*,*,#18335,.T.);
#24857=ORIENTED_EDGE('',*,*,#18320,.F.);
#24858=ORIENTED_EDGE('',*,*,#18297,.T.);
#24859=ORIENTED_EDGE('',*,*,#18340,.T.);
#24860=ORIENTED_EDGE('',*,*,#18331,.T.);
#24861=ORIENTED_EDGE('',*,*,#18329,.F.);
#24862=ORIENTED_EDGE('',*,*,#18310,.T.);
#24863=ORIENTED_EDGE('',*,*,#18315,.T.);
#24864=ORIENTED_EDGE('',*,*,#18338,.T.);
#24865=ORIENTED_EDGE('',*,*,#18341,.F.);
#24866=ORIENTED_EDGE('',*,*,#18311,.T.);
#24867=ORIENTED_EDGE('',*,*,#18341,.T.);
#24868=ORIENTED_EDGE('',*,*,#18337,.T.);
#24869=ORIENTED_EDGE('',*,*,#18342,.T.);
#24870=ORIENTED_EDGE('',*,*,#18312,.T.);
#24871=ORIENTED_EDGE('',*,*,#18342,.F.);
#24872=ORIENTED_EDGE('',*,*,#18336,.T.);
#24873=ORIENTED_EDGE('',*,*,#18339,.F.);
#24874=ORIENTED_EDGE('',*,*,#18304,.T.);
#24875=ORIENTED_EDGE('',*,*,#18343,.T.);
#24876=ORIENTED_EDGE('',*,*,#18332,.T.);
#24877=ORIENTED_EDGE('',*,*,#18340,.F.);
#24878=ORIENTED_EDGE('',*,*,#18303,.T.);
#24879=ORIENTED_EDGE('',*,*,#18344,.T.);
#24880=ORIENTED_EDGE('',*,*,#18333,.F.);
#24881=ORIENTED_EDGE('',*,*,#18343,.F.);
#24882=ORIENTED_EDGE('',*,*,#18302,.T.);
#24883=ORIENTED_EDGE('',*,*,#18324,.T.);
#24884=ORIENTED_EDGE('',*,*,#18334,.T.);
#24885=ORIENTED_EDGE('',*,*,#18344,.F.);
#24886=ORIENTED_EDGE('',*,*,#18345,.F.);
#24887=ORIENTED_EDGE('',*,*,#18346,.F.);
#24888=ORIENTED_EDGE('',*,*,#18347,.F.);
#24889=ORIENTED_EDGE('',*,*,#18348,.F.);
#24890=ORIENTED_EDGE('',*,*,#18349,.F.);
#24891=ORIENTED_EDGE('',*,*,#18350,.F.);
#24892=ORIENTED_EDGE('',*,*,#18351,.T.);
#24893=ORIENTED_EDGE('',*,*,#18352,.F.);
#24894=ORIENTED_EDGE('',*,*,#18353,.F.);
#24895=ORIENTED_EDGE('',*,*,#18354,.F.);
#24896=ORIENTED_EDGE('',*,*,#18355,.F.);
#24897=ORIENTED_EDGE('',*,*,#18356,.F.);
#24898=ORIENTED_EDGE('',*,*,#18357,.F.);
#24899=ORIENTED_EDGE('',*,*,#18358,.F.);
#24900=ORIENTED_EDGE('',*,*,#18359,.F.);
#24901=ORIENTED_EDGE('',*,*,#18360,.F.);
#24902=ORIENTED_EDGE('',*,*,#18357,.T.);
#24903=ORIENTED_EDGE('',*,*,#18361,.T.);
#24904=ORIENTED_EDGE('',*,*,#18362,.T.);
#24905=ORIENTED_EDGE('',*,*,#18363,.F.);
#24906=ORIENTED_EDGE('',*,*,#18356,.T.);
#24907=ORIENTED_EDGE('',*,*,#18364,.T.);
#24908=ORIENTED_EDGE('',*,*,#18365,.T.);
#24909=ORIENTED_EDGE('',*,*,#18361,.F.);
#24910=ORIENTED_EDGE('',*,*,#18355,.T.);
#24911=ORIENTED_EDGE('',*,*,#18366,.T.);
#24912=ORIENTED_EDGE('',*,*,#18367,.T.);
#24913=ORIENTED_EDGE('',*,*,#18364,.F.);
#24914=ORIENTED_EDGE('',*,*,#18354,.T.);
#24915=ORIENTED_EDGE('',*,*,#18368,.T.);
#24916=ORIENTED_EDGE('',*,*,#18369,.T.);
#24917=ORIENTED_EDGE('',*,*,#18366,.F.);
#24918=ORIENTED_EDGE('',*,*,#18349,.T.);
#24919=ORIENTED_EDGE('',*,*,#18370,.T.);
#24920=ORIENTED_EDGE('',*,*,#18371,.T.);
#24921=ORIENTED_EDGE('',*,*,#18372,.F.);
#24922=ORIENTED_EDGE('',*,*,#18348,.T.);
#24923=ORIENTED_EDGE('',*,*,#18373,.T.);
#24924=ORIENTED_EDGE('',*,*,#18374,.T.);
#24925=ORIENTED_EDGE('',*,*,#18370,.F.);
#24926=ORIENTED_EDGE('',*,*,#18347,.T.);
#24927=ORIENTED_EDGE('',*,*,#18375,.T.);
#24928=ORIENTED_EDGE('',*,*,#18376,.T.);
#24929=ORIENTED_EDGE('',*,*,#18373,.F.);
#24930=ORIENTED_EDGE('',*,*,#18346,.T.);
#24931=ORIENTED_EDGE('',*,*,#18377,.T.);
#24932=ORIENTED_EDGE('',*,*,#18378,.T.);
#24933=ORIENTED_EDGE('',*,*,#18375,.F.);
#24934=ORIENTED_EDGE('',*,*,#18371,.F.);
#24935=ORIENTED_EDGE('',*,*,#18374,.F.);
#24936=ORIENTED_EDGE('',*,*,#18376,.F.);
#24937=ORIENTED_EDGE('',*,*,#18378,.F.);
#24938=ORIENTED_EDGE('',*,*,#18379,.F.);
#24939=ORIENTED_EDGE('',*,*,#18380,.F.);
#24940=ORIENTED_EDGE('',*,*,#18381,.F.);
#24941=ORIENTED_EDGE('',*,*,#18382,.F.);
#24942=ORIENTED_EDGE('',*,*,#18362,.F.);
#24943=ORIENTED_EDGE('',*,*,#18365,.F.);
#24944=ORIENTED_EDGE('',*,*,#18367,.F.);
#24945=ORIENTED_EDGE('',*,*,#18369,.F.);
#24946=ORIENTED_EDGE('',*,*,#18383,.F.);
#24947=ORIENTED_EDGE('',*,*,#18384,.F.);
#24948=ORIENTED_EDGE('',*,*,#18385,.F.);
#24949=ORIENTED_EDGE('',*,*,#18386,.F.);
#24950=ORIENTED_EDGE('',*,*,#18353,.T.);
#24951=ORIENTED_EDGE('',*,*,#18387,.T.);
#24952=ORIENTED_EDGE('',*,*,#18383,.T.);
#24953=ORIENTED_EDGE('',*,*,#18368,.F.);
#24954=ORIENTED_EDGE('',*,*,#18345,.T.);
#24955=ORIENTED_EDGE('',*,*,#18388,.T.);
#24956=ORIENTED_EDGE('',*,*,#18379,.T.);
#24957=ORIENTED_EDGE('',*,*,#18377,.F.);
#24958=ORIENTED_EDGE('',*,*,#18358,.T.);
#24959=ORIENTED_EDGE('',*,*,#18363,.T.);
#24960=ORIENTED_EDGE('',*,*,#18386,.T.);
#24961=ORIENTED_EDGE('',*,*,#18389,.F.);
#24962=ORIENTED_EDGE('',*,*,#18359,.T.);
#24963=ORIENTED_EDGE('',*,*,#18389,.T.);
#24964=ORIENTED_EDGE('',*,*,#18385,.T.);
#24965=ORIENTED_EDGE('',*,*,#18390,.F.);
#24966=ORIENTED_EDGE('',*,*,#18360,.T.);
#24967=ORIENTED_EDGE('',*,*,#18390,.T.);
#24968=ORIENTED_EDGE('',*,*,#18384,.T.);
#24969=ORIENTED_EDGE('',*,*,#18387,.F.);
#24970=ORIENTED_EDGE('',*,*,#18350,.T.);
#24971=ORIENTED_EDGE('',*,*,#18372,.T.);
#24972=ORIENTED_EDGE('',*,*,#18382,.T.);
#24973=ORIENTED_EDGE('',*,*,#18391,.F.);
#24974=ORIENTED_EDGE('',*,*,#18381,.T.);
#24975=ORIENTED_EDGE('',*,*,#18392,.F.);
#24976=ORIENTED_EDGE('',*,*,#18351,.F.);
#24977=ORIENTED_EDGE('',*,*,#18391,.T.);
#24978=ORIENTED_EDGE('',*,*,#18352,.T.);
#24979=ORIENTED_EDGE('',*,*,#18392,.T.);
#24980=ORIENTED_EDGE('',*,*,#18380,.T.);
#24981=ORIENTED_EDGE('',*,*,#18388,.F.);
#24982=ORIENTED_EDGE('',*,*,#18393,.T.);
#24983=ORIENTED_EDGE('',*,*,#18394,.F.);
#24984=ORIENTED_EDGE('',*,*,#18395,.F.);
#24985=ORIENTED_EDGE('',*,*,#18396,.T.);
#24986=ORIENTED_EDGE('',*,*,#18397,.T.);
#24987=ORIENTED_EDGE('',*,*,#18398,.F.);
#24988=ORIENTED_EDGE('',*,*,#18399,.F.);
#24989=ORIENTED_EDGE('',*,*,#18394,.T.);
#24990=ORIENTED_EDGE('',*,*,#18400,.T.);
#24991=ORIENTED_EDGE('',*,*,#18401,.F.);
#24992=ORIENTED_EDGE('',*,*,#18402,.F.);
#24993=ORIENTED_EDGE('',*,*,#18398,.T.);
#24994=ORIENTED_EDGE('',*,*,#18403,.T.);
#24995=ORIENTED_EDGE('',*,*,#18404,.F.);
#24996=ORIENTED_EDGE('',*,*,#18405,.F.);
#24997=ORIENTED_EDGE('',*,*,#18401,.T.);
#24998=ORIENTED_EDGE('',*,*,#18406,.T.);
#24999=ORIENTED_EDGE('',*,*,#18407,.F.);
#25000=ORIENTED_EDGE('',*,*,#18408,.F.);
#25001=ORIENTED_EDGE('',*,*,#18409,.T.);
#25002=ORIENTED_EDGE('',*,*,#18410,.T.);
#25003=ORIENTED_EDGE('',*,*,#18411,.F.);
#25004=ORIENTED_EDGE('',*,*,#18412,.F.);
#25005=ORIENTED_EDGE('',*,*,#18407,.T.);
#25006=ORIENTED_EDGE('',*,*,#18413,.T.);
#25007=ORIENTED_EDGE('',*,*,#18414,.F.);
#25008=ORIENTED_EDGE('',*,*,#18415,.F.);
#25009=ORIENTED_EDGE('',*,*,#18411,.T.);
#25010=ORIENTED_EDGE('',*,*,#18416,.T.);
#25011=ORIENTED_EDGE('',*,*,#18417,.F.);
#25012=ORIENTED_EDGE('',*,*,#18418,.F.);
#25013=ORIENTED_EDGE('',*,*,#18414,.T.);
#25014=ORIENTED_EDGE('',*,*,#18419,.T.);
#25015=ORIENTED_EDGE('',*,*,#18420,.F.);
#25016=ORIENTED_EDGE('',*,*,#18421,.F.);
#25017=ORIENTED_EDGE('',*,*,#18404,.T.);
#25018=ORIENTED_EDGE('',*,*,#18422,.T.);
#25019=ORIENTED_EDGE('',*,*,#18396,.F.);
#25020=ORIENTED_EDGE('',*,*,#18423,.F.);
#25021=ORIENTED_EDGE('',*,*,#18424,.T.);
#25022=ORIENTED_EDGE('',*,*,#18425,.T.);
#25023=ORIENTED_EDGE('',*,*,#18424,.F.);
#25024=ORIENTED_EDGE('',*,*,#18426,.F.);
#25025=ORIENTED_EDGE('',*,*,#18427,.T.);
#25026=ORIENTED_EDGE('',*,*,#18428,.T.);
#25027=ORIENTED_EDGE('',*,*,#18427,.F.);
#25028=ORIENTED_EDGE('',*,*,#18429,.F.);
#25029=ORIENTED_EDGE('',*,*,#18420,.T.);
#25030=ORIENTED_EDGE('',*,*,#18430,.T.);
#25031=ORIENTED_EDGE('',*,*,#18431,.F.);
#25032=ORIENTED_EDGE('',*,*,#18432,.F.);
#25033=ORIENTED_EDGE('',*,*,#18417,.T.);
#25034=ORIENTED_EDGE('',*,*,#18433,.T.);
#25035=ORIENTED_EDGE('',*,*,#18434,.F.);
#25036=ORIENTED_EDGE('',*,*,#18435,.F.);
#25037=ORIENTED_EDGE('',*,*,#18431,.T.);
#25038=ORIENTED_EDGE('',*,*,#18436,.T.);
#25039=ORIENTED_EDGE('',*,*,#18437,.F.);
#25040=ORIENTED_EDGE('',*,*,#18438,.F.);
#25041=ORIENTED_EDGE('',*,*,#18434,.T.);
#25042=ORIENTED_EDGE('',*,*,#18439,.T.);
#25043=ORIENTED_EDGE('',*,*,#18409,.F.);
#25044=ORIENTED_EDGE('',*,*,#18440,.F.);
#25045=ORIENTED_EDGE('',*,*,#18437,.T.);
#25046=ORIENTED_EDGE('',*,*,#18432,.T.);
#25047=ORIENTED_EDGE('',*,*,#18435,.T.);
#25048=ORIENTED_EDGE('',*,*,#18438,.T.);
#25049=ORIENTED_EDGE('',*,*,#18440,.T.);
#25050=ORIENTED_EDGE('',*,*,#18408,.T.);
#25051=ORIENTED_EDGE('',*,*,#18412,.T.);
#25052=ORIENTED_EDGE('',*,*,#18415,.T.);
#25053=ORIENTED_EDGE('',*,*,#18418,.T.);
#25054=ORIENTED_EDGE('',*,*,#18421,.T.);
#25055=ORIENTED_EDGE('',*,*,#18429,.T.);
#25056=ORIENTED_EDGE('',*,*,#18426,.T.);
#25057=ORIENTED_EDGE('',*,*,#18423,.T.);
#25058=ORIENTED_EDGE('',*,*,#18395,.T.);
#25059=ORIENTED_EDGE('',*,*,#18399,.T.);
#25060=ORIENTED_EDGE('',*,*,#18402,.T.);
#25061=ORIENTED_EDGE('',*,*,#18405,.T.);
#25062=ORIENTED_EDGE('',*,*,#18430,.F.);
#25063=ORIENTED_EDGE('',*,*,#18416,.F.);
#25064=ORIENTED_EDGE('',*,*,#18413,.F.);
#25065=ORIENTED_EDGE('',*,*,#18410,.F.);
#25066=ORIENTED_EDGE('',*,*,#18406,.F.);
#25067=ORIENTED_EDGE('',*,*,#18439,.F.);
#25068=ORIENTED_EDGE('',*,*,#18436,.F.);
#25069=ORIENTED_EDGE('',*,*,#18433,.F.);
#25070=ORIENTED_EDGE('',*,*,#18419,.F.);
#25071=ORIENTED_EDGE('',*,*,#18403,.F.);
#25072=ORIENTED_EDGE('',*,*,#18400,.F.);
#25073=ORIENTED_EDGE('',*,*,#18397,.F.);
#25074=ORIENTED_EDGE('',*,*,#18393,.F.);
#25075=ORIENTED_EDGE('',*,*,#18422,.F.);
#25076=ORIENTED_EDGE('',*,*,#18425,.F.);
#25077=ORIENTED_EDGE('',*,*,#18428,.F.);
#25078=ORIENTED_EDGE('',*,*,#18441,.T.);
#25079=ORIENTED_EDGE('',*,*,#18442,.F.);
#25080=ORIENTED_EDGE('',*,*,#18443,.F.);
#25081=ORIENTED_EDGE('',*,*,#18444,.T.);
#25082=ORIENTED_EDGE('',*,*,#18445,.T.);
#25083=ORIENTED_EDGE('',*,*,#18446,.F.);
#25084=ORIENTED_EDGE('',*,*,#18447,.F.);
#25085=ORIENTED_EDGE('',*,*,#18442,.T.);
#25086=ORIENTED_EDGE('',*,*,#18448,.T.);
#25087=ORIENTED_EDGE('',*,*,#18449,.F.);
#25088=ORIENTED_EDGE('',*,*,#18450,.F.);
#25089=ORIENTED_EDGE('',*,*,#18446,.T.);
#25090=ORIENTED_EDGE('',*,*,#18451,.T.);
#25091=ORIENTED_EDGE('',*,*,#18452,.F.);
#25092=ORIENTED_EDGE('',*,*,#18453,.F.);
#25093=ORIENTED_EDGE('',*,*,#18449,.T.);
#25094=ORIENTED_EDGE('',*,*,#18454,.T.);
#25095=ORIENTED_EDGE('',*,*,#18455,.F.);
#25096=ORIENTED_EDGE('',*,*,#18456,.F.);
#25097=ORIENTED_EDGE('',*,*,#18457,.T.);
#25098=ORIENTED_EDGE('',*,*,#18458,.T.);
#25099=ORIENTED_EDGE('',*,*,#18459,.F.);
#25100=ORIENTED_EDGE('',*,*,#18460,.F.);
#25101=ORIENTED_EDGE('',*,*,#18455,.T.);
#25102=ORIENTED_EDGE('',*,*,#18461,.T.);
#25103=ORIENTED_EDGE('',*,*,#18462,.F.);
#25104=ORIENTED_EDGE('',*,*,#18463,.F.);
#25105=ORIENTED_EDGE('',*,*,#18459,.T.);
#25106=ORIENTED_EDGE('',*,*,#18464,.T.);
#25107=ORIENTED_EDGE('',*,*,#18465,.F.);
#25108=ORIENTED_EDGE('',*,*,#18466,.F.);
#25109=ORIENTED_EDGE('',*,*,#18462,.T.);
#25110=ORIENTED_EDGE('',*,*,#18467,.T.);
#25111=ORIENTED_EDGE('',*,*,#18468,.F.);
#25112=ORIENTED_EDGE('',*,*,#18469,.F.);
#25113=ORIENTED_EDGE('',*,*,#18452,.T.);
#25114=ORIENTED_EDGE('',*,*,#18470,.T.);
#25115=ORIENTED_EDGE('',*,*,#18444,.F.);
#25116=ORIENTED_EDGE('',*,*,#18471,.F.);
#25117=ORIENTED_EDGE('',*,*,#18472,.T.);
#25118=ORIENTED_EDGE('',*,*,#18473,.T.);
#25119=ORIENTED_EDGE('',*,*,#18472,.F.);
#25120=ORIENTED_EDGE('',*,*,#18474,.F.);
#25121=ORIENTED_EDGE('',*,*,#18475,.T.);
#25122=ORIENTED_EDGE('',*,*,#18476,.T.);
#25123=ORIENTED_EDGE('',*,*,#18475,.F.);
#25124=ORIENTED_EDGE('',*,*,#18477,.F.);
#25125=ORIENTED_EDGE('',*,*,#18468,.T.);
#25126=ORIENTED_EDGE('',*,*,#18478,.T.);
#25127=ORIENTED_EDGE('',*,*,#18479,.F.);
#25128=ORIENTED_EDGE('',*,*,#18480,.F.);
#25129=ORIENTED_EDGE('',*,*,#18465,.T.);
#25130=ORIENTED_EDGE('',*,*,#18481,.T.);
#25131=ORIENTED_EDGE('',*,*,#18482,.F.);
#25132=ORIENTED_EDGE('',*,*,#18483,.F.);
#25133=ORIENTED_EDGE('',*,*,#18479,.T.);
#25134=ORIENTED_EDGE('',*,*,#18484,.T.);
#25135=ORIENTED_EDGE('',*,*,#18485,.F.);
#25136=ORIENTED_EDGE('',*,*,#18486,.F.);
#25137=ORIENTED_EDGE('',*,*,#18482,.T.);
#25138=ORIENTED_EDGE('',*,*,#18487,.T.);
#25139=ORIENTED_EDGE('',*,*,#18457,.F.);
#25140=ORIENTED_EDGE('',*,*,#18488,.F.);
#25141=ORIENTED_EDGE('',*,*,#18485,.T.);
#25142=ORIENTED_EDGE('',*,*,#18480,.T.);
#25143=ORIENTED_EDGE('',*,*,#18483,.T.);
#25144=ORIENTED_EDGE('',*,*,#18486,.T.);
#25145=ORIENTED_EDGE('',*,*,#18488,.T.);
#25146=ORIENTED_EDGE('',*,*,#18456,.T.);
#25147=ORIENTED_EDGE('',*,*,#18460,.T.);
#25148=ORIENTED_EDGE('',*,*,#18463,.T.);
#25149=ORIENTED_EDGE('',*,*,#18466,.T.);
#25150=ORIENTED_EDGE('',*,*,#18469,.T.);
#25151=ORIENTED_EDGE('',*,*,#18477,.T.);
#25152=ORIENTED_EDGE('',*,*,#18474,.T.);
#25153=ORIENTED_EDGE('',*,*,#18471,.T.);
#25154=ORIENTED_EDGE('',*,*,#18443,.T.);
#25155=ORIENTED_EDGE('',*,*,#18447,.T.);
#25156=ORIENTED_EDGE('',*,*,#18450,.T.);
#25157=ORIENTED_EDGE('',*,*,#18453,.T.);
#25158=ORIENTED_EDGE('',*,*,#18478,.F.);
#25159=ORIENTED_EDGE('',*,*,#18464,.F.);
#25160=ORIENTED_EDGE('',*,*,#18461,.F.);
#25161=ORIENTED_EDGE('',*,*,#18458,.F.);
#25162=ORIENTED_EDGE('',*,*,#18454,.F.);
#25163=ORIENTED_EDGE('',*,*,#18487,.F.);
#25164=ORIENTED_EDGE('',*,*,#18484,.F.);
#25165=ORIENTED_EDGE('',*,*,#18481,.F.);
#25166=ORIENTED_EDGE('',*,*,#18467,.F.);
#25167=ORIENTED_EDGE('',*,*,#18451,.F.);
#25168=ORIENTED_EDGE('',*,*,#18448,.F.);
#25169=ORIENTED_EDGE('',*,*,#18445,.F.);
#25170=ORIENTED_EDGE('',*,*,#18441,.F.);
#25171=ORIENTED_EDGE('',*,*,#18470,.F.);
#25172=ORIENTED_EDGE('',*,*,#18473,.F.);
#25173=ORIENTED_EDGE('',*,*,#18476,.F.);
#25174=ORIENTED_EDGE('',*,*,#18489,.T.);
#25175=ORIENTED_EDGE('',*,*,#18490,.F.);
#25176=ORIENTED_EDGE('',*,*,#18491,.F.);
#25177=ORIENTED_EDGE('',*,*,#18492,.T.);
#25178=ORIENTED_EDGE('',*,*,#18493,.T.);
#25179=ORIENTED_EDGE('',*,*,#18494,.F.);
#25180=ORIENTED_EDGE('',*,*,#18495,.F.);
#25181=ORIENTED_EDGE('',*,*,#18490,.T.);
#25182=ORIENTED_EDGE('',*,*,#18496,.T.);
#25183=ORIENTED_EDGE('',*,*,#18497,.F.);
#25184=ORIENTED_EDGE('',*,*,#18498,.F.);
#25185=ORIENTED_EDGE('',*,*,#18494,.T.);
#25186=ORIENTED_EDGE('',*,*,#18499,.T.);
#25187=ORIENTED_EDGE('',*,*,#18500,.F.);
#25188=ORIENTED_EDGE('',*,*,#18501,.F.);
#25189=ORIENTED_EDGE('',*,*,#18497,.T.);
#25190=ORIENTED_EDGE('',*,*,#18502,.T.);
#25191=ORIENTED_EDGE('',*,*,#18503,.F.);
#25192=ORIENTED_EDGE('',*,*,#18504,.F.);
#25193=ORIENTED_EDGE('',*,*,#18505,.T.);
#25194=ORIENTED_EDGE('',*,*,#18506,.T.);
#25195=ORIENTED_EDGE('',*,*,#18507,.F.);
#25196=ORIENTED_EDGE('',*,*,#18508,.F.);
#25197=ORIENTED_EDGE('',*,*,#18503,.T.);
#25198=ORIENTED_EDGE('',*,*,#18509,.T.);
#25199=ORIENTED_EDGE('',*,*,#18510,.F.);
#25200=ORIENTED_EDGE('',*,*,#18511,.F.);
#25201=ORIENTED_EDGE('',*,*,#18507,.T.);
#25202=ORIENTED_EDGE('',*,*,#18512,.T.);
#25203=ORIENTED_EDGE('',*,*,#18513,.F.);
#25204=ORIENTED_EDGE('',*,*,#18514,.F.);
#25205=ORIENTED_EDGE('',*,*,#18510,.T.);
#25206=ORIENTED_EDGE('',*,*,#18515,.T.);
#25207=ORIENTED_EDGE('',*,*,#18516,.F.);
#25208=ORIENTED_EDGE('',*,*,#18517,.F.);
#25209=ORIENTED_EDGE('',*,*,#18500,.T.);
#25210=ORIENTED_EDGE('',*,*,#18518,.T.);
#25211=ORIENTED_EDGE('',*,*,#18492,.F.);
#25212=ORIENTED_EDGE('',*,*,#18519,.F.);
#25213=ORIENTED_EDGE('',*,*,#18520,.T.);
#25214=ORIENTED_EDGE('',*,*,#18521,.T.);
#25215=ORIENTED_EDGE('',*,*,#18520,.F.);
#25216=ORIENTED_EDGE('',*,*,#18522,.F.);
#25217=ORIENTED_EDGE('',*,*,#18523,.T.);
#25218=ORIENTED_EDGE('',*,*,#18524,.T.);
#25219=ORIENTED_EDGE('',*,*,#18523,.F.);
#25220=ORIENTED_EDGE('',*,*,#18525,.F.);
#25221=ORIENTED_EDGE('',*,*,#18516,.T.);
#25222=ORIENTED_EDGE('',*,*,#18526,.T.);
#25223=ORIENTED_EDGE('',*,*,#18527,.F.);
#25224=ORIENTED_EDGE('',*,*,#18528,.F.);
#25225=ORIENTED_EDGE('',*,*,#18513,.T.);
#25226=ORIENTED_EDGE('',*,*,#18529,.T.);
#25227=ORIENTED_EDGE('',*,*,#18530,.F.);
#25228=ORIENTED_EDGE('',*,*,#18531,.F.);
#25229=ORIENTED_EDGE('',*,*,#18527,.T.);
#25230=ORIENTED_EDGE('',*,*,#18532,.T.);
#25231=ORIENTED_EDGE('',*,*,#18533,.F.);
#25232=ORIENTED_EDGE('',*,*,#18534,.F.);
#25233=ORIENTED_EDGE('',*,*,#18530,.T.);
#25234=ORIENTED_EDGE('',*,*,#18535,.T.);
#25235=ORIENTED_EDGE('',*,*,#18505,.F.);
#25236=ORIENTED_EDGE('',*,*,#18536,.F.);
#25237=ORIENTED_EDGE('',*,*,#18533,.T.);
#25238=ORIENTED_EDGE('',*,*,#18528,.T.);
#25239=ORIENTED_EDGE('',*,*,#18531,.T.);
#25240=ORIENTED_EDGE('',*,*,#18534,.T.);
#25241=ORIENTED_EDGE('',*,*,#18536,.T.);
#25242=ORIENTED_EDGE('',*,*,#18504,.T.);
#25243=ORIENTED_EDGE('',*,*,#18508,.T.);
#25244=ORIENTED_EDGE('',*,*,#18511,.T.);
#25245=ORIENTED_EDGE('',*,*,#18514,.T.);
#25246=ORIENTED_EDGE('',*,*,#18517,.T.);
#25247=ORIENTED_EDGE('',*,*,#18525,.T.);
#25248=ORIENTED_EDGE('',*,*,#18522,.T.);
#25249=ORIENTED_EDGE('',*,*,#18519,.T.);
#25250=ORIENTED_EDGE('',*,*,#18491,.T.);
#25251=ORIENTED_EDGE('',*,*,#18495,.T.);
#25252=ORIENTED_EDGE('',*,*,#18498,.T.);
#25253=ORIENTED_EDGE('',*,*,#18501,.T.);
#25254=ORIENTED_EDGE('',*,*,#18526,.F.);
#25255=ORIENTED_EDGE('',*,*,#18512,.F.);
#25256=ORIENTED_EDGE('',*,*,#18509,.F.);
#25257=ORIENTED_EDGE('',*,*,#18506,.F.);
#25258=ORIENTED_EDGE('',*,*,#18502,.F.);
#25259=ORIENTED_EDGE('',*,*,#18535,.F.);
#25260=ORIENTED_EDGE('',*,*,#18532,.F.);
#25261=ORIENTED_EDGE('',*,*,#18529,.F.);
#25262=ORIENTED_EDGE('',*,*,#18515,.F.);
#25263=ORIENTED_EDGE('',*,*,#18499,.F.);
#25264=ORIENTED_EDGE('',*,*,#18496,.F.);
#25265=ORIENTED_EDGE('',*,*,#18493,.F.);
#25266=ORIENTED_EDGE('',*,*,#18489,.F.);
#25267=ORIENTED_EDGE('',*,*,#18518,.F.);
#25268=ORIENTED_EDGE('',*,*,#18521,.F.);
#25269=ORIENTED_EDGE('',*,*,#18524,.F.);
#25270=ORIENTED_EDGE('',*,*,#18537,.F.);
#25271=ORIENTED_EDGE('',*,*,#18538,.T.);
#25272=ORIENTED_EDGE('',*,*,#18539,.F.);
#25273=ORIENTED_EDGE('',*,*,#18540,.F.);
#25274=ORIENTED_EDGE('',*,*,#18541,.F.);
#25275=ORIENTED_EDGE('',*,*,#18542,.T.);
#25276=ORIENTED_EDGE('',*,*,#18543,.F.);
#25277=ORIENTED_EDGE('',*,*,#18538,.F.);
#25278=ORIENTED_EDGE('',*,*,#18544,.F.);
#25279=ORIENTED_EDGE('',*,*,#18545,.T.);
#25280=ORIENTED_EDGE('',*,*,#18546,.F.);
#25281=ORIENTED_EDGE('',*,*,#18542,.F.);
#25282=ORIENTED_EDGE('',*,*,#18547,.F.);
#25283=ORIENTED_EDGE('',*,*,#18548,.T.);
#25284=ORIENTED_EDGE('',*,*,#18549,.F.);
#25285=ORIENTED_EDGE('',*,*,#18545,.F.);
#25286=ORIENTED_EDGE('',*,*,#18550,.F.);
#25287=ORIENTED_EDGE('',*,*,#18551,.T.);
#25288=ORIENTED_EDGE('',*,*,#18552,.F.);
#25289=ORIENTED_EDGE('',*,*,#18548,.F.);
#25290=ORIENTED_EDGE('',*,*,#18553,.F.);
#25291=ORIENTED_EDGE('',*,*,#18554,.T.);
#25292=ORIENTED_EDGE('',*,*,#18555,.F.);
#25293=ORIENTED_EDGE('',*,*,#18551,.F.);
#25294=ORIENTED_EDGE('',*,*,#18556,.F.);
#25295=ORIENTED_EDGE('',*,*,#18557,.T.);
#25296=ORIENTED_EDGE('',*,*,#18558,.F.);
#25297=ORIENTED_EDGE('',*,*,#18554,.F.);
#25298=ORIENTED_EDGE('',*,*,#18559,.F.);
#25299=ORIENTED_EDGE('',*,*,#18540,.T.);
#25300=ORIENTED_EDGE('',*,*,#18560,.F.);
#25301=ORIENTED_EDGE('',*,*,#18557,.F.);
#25302=ORIENTED_EDGE('',*,*,#18561,.F.);
#25303=ORIENTED_EDGE('',*,*,#18562,.T.);
#25304=ORIENTED_EDGE('',*,*,#18563,.F.);
#25305=ORIENTED_EDGE('',*,*,#18564,.F.);
#25306=ORIENTED_EDGE('',*,*,#18565,.F.);
#25307=ORIENTED_EDGE('',*,*,#18564,.T.);
#25308=ORIENTED_EDGE('',*,*,#18566,.F.);
#25309=ORIENTED_EDGE('',*,*,#18567,.F.);
#25310=ORIENTED_EDGE('',*,*,#18568,.F.);
#25311=ORIENTED_EDGE('',*,*,#18567,.T.);
#25312=ORIENTED_EDGE('',*,*,#18569,.F.);
#25313=ORIENTED_EDGE('',*,*,#18570,.F.);
#25314=ORIENTED_EDGE('',*,*,#18571,.F.);
#25315=ORIENTED_EDGE('',*,*,#18570,.T.);
#25316=ORIENTED_EDGE('',*,*,#18572,.F.);
#25317=ORIENTED_EDGE('',*,*,#18573,.F.);
#25318=ORIENTED_EDGE('',*,*,#18574,.F.);
#25319=ORIENTED_EDGE('',*,*,#18573,.T.);
#25320=ORIENTED_EDGE('',*,*,#18575,.F.);
#25321=ORIENTED_EDGE('',*,*,#18576,.F.);
#25322=ORIENTED_EDGE('',*,*,#18577,.F.);
#25323=ORIENTED_EDGE('',*,*,#18576,.T.);
#25324=ORIENTED_EDGE('',*,*,#18578,.F.);
#25325=ORIENTED_EDGE('',*,*,#18579,.F.);
#25326=ORIENTED_EDGE('',*,*,#18580,.F.);
#25327=ORIENTED_EDGE('',*,*,#18579,.T.);
#25328=ORIENTED_EDGE('',*,*,#18581,.F.);
#25329=ORIENTED_EDGE('',*,*,#18582,.F.);
#25330=ORIENTED_EDGE('',*,*,#18583,.F.);
#25331=ORIENTED_EDGE('',*,*,#18582,.T.);
#25332=ORIENTED_EDGE('',*,*,#18584,.F.);
#25333=ORIENTED_EDGE('',*,*,#18562,.F.);
#25334=ORIENTED_EDGE('',*,*,#18583,.T.);
#25335=ORIENTED_EDGE('',*,*,#18561,.T.);
#25336=ORIENTED_EDGE('',*,*,#18565,.T.);
#25337=ORIENTED_EDGE('',*,*,#18568,.T.);
#25338=ORIENTED_EDGE('',*,*,#18571,.T.);
#25339=ORIENTED_EDGE('',*,*,#18574,.T.);
#25340=ORIENTED_EDGE('',*,*,#18577,.T.);
#25341=ORIENTED_EDGE('',*,*,#18580,.T.);
#25342=ORIENTED_EDGE('',*,*,#18537,.T.);
#25343=ORIENTED_EDGE('',*,*,#18559,.T.);
#25344=ORIENTED_EDGE('',*,*,#18556,.T.);
#25345=ORIENTED_EDGE('',*,*,#18553,.T.);
#25346=ORIENTED_EDGE('',*,*,#18550,.T.);
#25347=ORIENTED_EDGE('',*,*,#18547,.T.);
#25348=ORIENTED_EDGE('',*,*,#18544,.T.);
#25349=ORIENTED_EDGE('',*,*,#18541,.T.);
#25350=ORIENTED_EDGE('',*,*,#18584,.T.);
#25351=ORIENTED_EDGE('',*,*,#18581,.T.);
#25352=ORIENTED_EDGE('',*,*,#18578,.T.);
#25353=ORIENTED_EDGE('',*,*,#18575,.T.);
#25354=ORIENTED_EDGE('',*,*,#18572,.T.);
#25355=ORIENTED_EDGE('',*,*,#18569,.T.);
#25356=ORIENTED_EDGE('',*,*,#18566,.T.);
#25357=ORIENTED_EDGE('',*,*,#18563,.T.);
#25358=ORIENTED_EDGE('',*,*,#18539,.T.);
#25359=ORIENTED_EDGE('',*,*,#18543,.T.);
#25360=ORIENTED_EDGE('',*,*,#18546,.T.);
#25361=ORIENTED_EDGE('',*,*,#18549,.T.);
#25362=ORIENTED_EDGE('',*,*,#18552,.T.);
#25363=ORIENTED_EDGE('',*,*,#18555,.T.);
#25364=ORIENTED_EDGE('',*,*,#18558,.T.);
#25365=ORIENTED_EDGE('',*,*,#18560,.T.);
#25366=ORIENTED_EDGE('',*,*,#18585,.F.);
#25367=ORIENTED_EDGE('',*,*,#18586,.T.);
#25368=ORIENTED_EDGE('',*,*,#18587,.F.);
#25369=ORIENTED_EDGE('',*,*,#18588,.F.);
#25370=ORIENTED_EDGE('',*,*,#18589,.F.);
#25371=ORIENTED_EDGE('',*,*,#18590,.T.);
#25372=ORIENTED_EDGE('',*,*,#18591,.F.);
#25373=ORIENTED_EDGE('',*,*,#18586,.F.);
#25374=ORIENTED_EDGE('',*,*,#18592,.F.);
#25375=ORIENTED_EDGE('',*,*,#18593,.T.);
#25376=ORIENTED_EDGE('',*,*,#18594,.F.);
#25377=ORIENTED_EDGE('',*,*,#18590,.F.);
#25378=ORIENTED_EDGE('',*,*,#18595,.F.);
#25379=ORIENTED_EDGE('',*,*,#18596,.T.);
#25380=ORIENTED_EDGE('',*,*,#18597,.F.);
#25381=ORIENTED_EDGE('',*,*,#18593,.F.);
#25382=ORIENTED_EDGE('',*,*,#18598,.F.);
#25383=ORIENTED_EDGE('',*,*,#18599,.T.);
#25384=ORIENTED_EDGE('',*,*,#18600,.F.);
#25385=ORIENTED_EDGE('',*,*,#18596,.F.);
#25386=ORIENTED_EDGE('',*,*,#18601,.F.);
#25387=ORIENTED_EDGE('',*,*,#18602,.T.);
#25388=ORIENTED_EDGE('',*,*,#18603,.F.);
#25389=ORIENTED_EDGE('',*,*,#18599,.F.);
#25390=ORIENTED_EDGE('',*,*,#18604,.F.);
#25391=ORIENTED_EDGE('',*,*,#18605,.T.);
#25392=ORIENTED_EDGE('',*,*,#18606,.F.);
#25393=ORIENTED_EDGE('',*,*,#18602,.F.);
#25394=ORIENTED_EDGE('',*,*,#18607,.F.);
#25395=ORIENTED_EDGE('',*,*,#18588,.T.);
#25396=ORIENTED_EDGE('',*,*,#18608,.F.);
#25397=ORIENTED_EDGE('',*,*,#18605,.F.);
#25398=ORIENTED_EDGE('',*,*,#18609,.F.);
#25399=ORIENTED_EDGE('',*,*,#18610,.T.);
#25400=ORIENTED_EDGE('',*,*,#18611,.F.);
#25401=ORIENTED_EDGE('',*,*,#18612,.F.);
#25402=ORIENTED_EDGE('',*,*,#18613,.F.);
#25403=ORIENTED_EDGE('',*,*,#18612,.T.);
#25404=ORIENTED_EDGE('',*,*,#18614,.F.);
#25405=ORIENTED_EDGE('',*,*,#18615,.F.);
#25406=ORIENTED_EDGE('',*,*,#18616,.F.);
#25407=ORIENTED_EDGE('',*,*,#18615,.T.);
#25408=ORIENTED_EDGE('',*,*,#18617,.F.);
#25409=ORIENTED_EDGE('',*,*,#18618,.F.);
#25410=ORIENTED_EDGE('',*,*,#18619,.F.);
#25411=ORIENTED_EDGE('',*,*,#18618,.T.);
#25412=ORIENTED_EDGE('',*,*,#18620,.F.);
#25413=ORIENTED_EDGE('',*,*,#18621,.F.);
#25414=ORIENTED_EDGE('',*,*,#18622,.F.);
#25415=ORIENTED_EDGE('',*,*,#18621,.T.);
#25416=ORIENTED_EDGE('',*,*,#18623,.F.);
#25417=ORIENTED_EDGE('',*,*,#18624,.F.);
#25418=ORIENTED_EDGE('',*,*,#18625,.F.);
#25419=ORIENTED_EDGE('',*,*,#18624,.T.);
#25420=ORIENTED_EDGE('',*,*,#18626,.F.);
#25421=ORIENTED_EDGE('',*,*,#18627,.F.);
#25422=ORIENTED_EDGE('',*,*,#18628,.F.);
#25423=ORIENTED_EDGE('',*,*,#18627,.T.);
#25424=ORIENTED_EDGE('',*,*,#18629,.F.);
#25425=ORIENTED_EDGE('',*,*,#18630,.F.);
#25426=ORIENTED_EDGE('',*,*,#18631,.F.);
#25427=ORIENTED_EDGE('',*,*,#18630,.T.);
#25428=ORIENTED_EDGE('',*,*,#18632,.F.);
#25429=ORIENTED_EDGE('',*,*,#18610,.F.);
#25430=ORIENTED_EDGE('',*,*,#18631,.T.);
#25431=ORIENTED_EDGE('',*,*,#18609,.T.);
#25432=ORIENTED_EDGE('',*,*,#18613,.T.);
#25433=ORIENTED_EDGE('',*,*,#18616,.T.);
#25434=ORIENTED_EDGE('',*,*,#18619,.T.);
#25435=ORIENTED_EDGE('',*,*,#18622,.T.);
#25436=ORIENTED_EDGE('',*,*,#18625,.T.);
#25437=ORIENTED_EDGE('',*,*,#18628,.T.);
#25438=ORIENTED_EDGE('',*,*,#18585,.T.);
#25439=ORIENTED_EDGE('',*,*,#18607,.T.);
#25440=ORIENTED_EDGE('',*,*,#18604,.T.);
#25441=ORIENTED_EDGE('',*,*,#18601,.T.);
#25442=ORIENTED_EDGE('',*,*,#18598,.T.);
#25443=ORIENTED_EDGE('',*,*,#18595,.T.);
#25444=ORIENTED_EDGE('',*,*,#18592,.T.);
#25445=ORIENTED_EDGE('',*,*,#18589,.T.);
#25446=ORIENTED_EDGE('',*,*,#18632,.T.);
#25447=ORIENTED_EDGE('',*,*,#18629,.T.);
#25448=ORIENTED_EDGE('',*,*,#18626,.T.);
#25449=ORIENTED_EDGE('',*,*,#18623,.T.);
#25450=ORIENTED_EDGE('',*,*,#18620,.T.);
#25451=ORIENTED_EDGE('',*,*,#18617,.T.);
#25452=ORIENTED_EDGE('',*,*,#18614,.T.);
#25453=ORIENTED_EDGE('',*,*,#18611,.T.);
#25454=ORIENTED_EDGE('',*,*,#18587,.T.);
#25455=ORIENTED_EDGE('',*,*,#18591,.T.);
#25456=ORIENTED_EDGE('',*,*,#18594,.T.);
#25457=ORIENTED_EDGE('',*,*,#18597,.T.);
#25458=ORIENTED_EDGE('',*,*,#18600,.T.);
#25459=ORIENTED_EDGE('',*,*,#18603,.T.);
#25460=ORIENTED_EDGE('',*,*,#18606,.T.);
#25461=ORIENTED_EDGE('',*,*,#18608,.T.);
#25462=ORIENTED_EDGE('',*,*,#18633,.F.);
#25463=ORIENTED_EDGE('',*,*,#18634,.T.);
#25464=ORIENTED_EDGE('',*,*,#18635,.F.);
#25465=ORIENTED_EDGE('',*,*,#18636,.F.);
#25466=ORIENTED_EDGE('',*,*,#18637,.F.);
#25467=ORIENTED_EDGE('',*,*,#18638,.T.);
#25468=ORIENTED_EDGE('',*,*,#18639,.F.);
#25469=ORIENTED_EDGE('',*,*,#18634,.F.);
#25470=ORIENTED_EDGE('',*,*,#18640,.F.);
#25471=ORIENTED_EDGE('',*,*,#18641,.T.);
#25472=ORIENTED_EDGE('',*,*,#18642,.F.);
#25473=ORIENTED_EDGE('',*,*,#18638,.F.);
#25474=ORIENTED_EDGE('',*,*,#18643,.F.);
#25475=ORIENTED_EDGE('',*,*,#18644,.T.);
#25476=ORIENTED_EDGE('',*,*,#18645,.F.);
#25477=ORIENTED_EDGE('',*,*,#18641,.F.);
#25478=ORIENTED_EDGE('',*,*,#18646,.F.);
#25479=ORIENTED_EDGE('',*,*,#18647,.T.);
#25480=ORIENTED_EDGE('',*,*,#18648,.F.);
#25481=ORIENTED_EDGE('',*,*,#18644,.F.);
#25482=ORIENTED_EDGE('',*,*,#18649,.F.);
#25483=ORIENTED_EDGE('',*,*,#18650,.T.);
#25484=ORIENTED_EDGE('',*,*,#18651,.F.);
#25485=ORIENTED_EDGE('',*,*,#18647,.F.);
#25486=ORIENTED_EDGE('',*,*,#18652,.F.);
#25487=ORIENTED_EDGE('',*,*,#18653,.T.);
#25488=ORIENTED_EDGE('',*,*,#18654,.F.);
#25489=ORIENTED_EDGE('',*,*,#18650,.F.);
#25490=ORIENTED_EDGE('',*,*,#18655,.F.);
#25491=ORIENTED_EDGE('',*,*,#18636,.T.);
#25492=ORIENTED_EDGE('',*,*,#18656,.F.);
#25493=ORIENTED_EDGE('',*,*,#18653,.F.);
#25494=ORIENTED_EDGE('',*,*,#18657,.F.);
#25495=ORIENTED_EDGE('',*,*,#18658,.T.);
#25496=ORIENTED_EDGE('',*,*,#18659,.F.);
#25497=ORIENTED_EDGE('',*,*,#18660,.F.);
#25498=ORIENTED_EDGE('',*,*,#18661,.F.);
#25499=ORIENTED_EDGE('',*,*,#18660,.T.);
#25500=ORIENTED_EDGE('',*,*,#18662,.F.);
#25501=ORIENTED_EDGE('',*,*,#18663,.F.);
#25502=ORIENTED_EDGE('',*,*,#18664,.F.);
#25503=ORIENTED_EDGE('',*,*,#18663,.T.);
#25504=ORIENTED_EDGE('',*,*,#18665,.F.);
#25505=ORIENTED_EDGE('',*,*,#18666,.F.);
#25506=ORIENTED_EDGE('',*,*,#18667,.F.);
#25507=ORIENTED_EDGE('',*,*,#18666,.T.);
#25508=ORIENTED_EDGE('',*,*,#18668,.F.);
#25509=ORIENTED_EDGE('',*,*,#18669,.F.);
#25510=ORIENTED_EDGE('',*,*,#18670,.F.);
#25511=ORIENTED_EDGE('',*,*,#18669,.T.);
#25512=ORIENTED_EDGE('',*,*,#18671,.F.);
#25513=ORIENTED_EDGE('',*,*,#18672,.F.);
#25514=ORIENTED_EDGE('',*,*,#18673,.F.);
#25515=ORIENTED_EDGE('',*,*,#18672,.T.);
#25516=ORIENTED_EDGE('',*,*,#18674,.F.);
#25517=ORIENTED_EDGE('',*,*,#18675,.F.);
#25518=ORIENTED_EDGE('',*,*,#18676,.F.);
#25519=ORIENTED_EDGE('',*,*,#18675,.T.);
#25520=ORIENTED_EDGE('',*,*,#18677,.F.);
#25521=ORIENTED_EDGE('',*,*,#18678,.F.);
#25522=ORIENTED_EDGE('',*,*,#18679,.F.);
#25523=ORIENTED_EDGE('',*,*,#18678,.T.);
#25524=ORIENTED_EDGE('',*,*,#18680,.F.);
#25525=ORIENTED_EDGE('',*,*,#18658,.F.);
#25526=ORIENTED_EDGE('',*,*,#18679,.T.);
#25527=ORIENTED_EDGE('',*,*,#18657,.T.);
#25528=ORIENTED_EDGE('',*,*,#18661,.T.);
#25529=ORIENTED_EDGE('',*,*,#18664,.T.);
#25530=ORIENTED_EDGE('',*,*,#18667,.T.);
#25531=ORIENTED_EDGE('',*,*,#18670,.T.);
#25532=ORIENTED_EDGE('',*,*,#18673,.T.);
#25533=ORIENTED_EDGE('',*,*,#18676,.T.);
#25534=ORIENTED_EDGE('',*,*,#18633,.T.);
#25535=ORIENTED_EDGE('',*,*,#18655,.T.);
#25536=ORIENTED_EDGE('',*,*,#18652,.T.);
#25537=ORIENTED_EDGE('',*,*,#18649,.T.);
#25538=ORIENTED_EDGE('',*,*,#18646,.T.);
#25539=ORIENTED_EDGE('',*,*,#18643,.T.);
#25540=ORIENTED_EDGE('',*,*,#18640,.T.);
#25541=ORIENTED_EDGE('',*,*,#18637,.T.);
#25542=ORIENTED_EDGE('',*,*,#18680,.T.);
#25543=ORIENTED_EDGE('',*,*,#18677,.T.);
#25544=ORIENTED_EDGE('',*,*,#18674,.T.);
#25545=ORIENTED_EDGE('',*,*,#18671,.T.);
#25546=ORIENTED_EDGE('',*,*,#18668,.T.);
#25547=ORIENTED_EDGE('',*,*,#18665,.T.);
#25548=ORIENTED_EDGE('',*,*,#18662,.T.);
#25549=ORIENTED_EDGE('',*,*,#18659,.T.);
#25550=ORIENTED_EDGE('',*,*,#18635,.T.);
#25551=ORIENTED_EDGE('',*,*,#18639,.T.);
#25552=ORIENTED_EDGE('',*,*,#18642,.T.);
#25553=ORIENTED_EDGE('',*,*,#18645,.T.);
#25554=ORIENTED_EDGE('',*,*,#18648,.T.);
#25555=ORIENTED_EDGE('',*,*,#18651,.T.);
#25556=ORIENTED_EDGE('',*,*,#18654,.T.);
#25557=ORIENTED_EDGE('',*,*,#18656,.T.);
#25558=ORIENTED_EDGE('',*,*,#18681,.F.);
#25559=ORIENTED_EDGE('',*,*,#18682,.T.);
#25560=ORIENTED_EDGE('',*,*,#18683,.F.);
#25561=ORIENTED_EDGE('',*,*,#18684,.F.);
#25562=ORIENTED_EDGE('',*,*,#18685,.F.);
#25563=ORIENTED_EDGE('',*,*,#18686,.T.);
#25564=ORIENTED_EDGE('',*,*,#18687,.F.);
#25565=ORIENTED_EDGE('',*,*,#18682,.F.);
#25566=ORIENTED_EDGE('',*,*,#18688,.F.);
#25567=ORIENTED_EDGE('',*,*,#18689,.T.);
#25568=ORIENTED_EDGE('',*,*,#18690,.F.);
#25569=ORIENTED_EDGE('',*,*,#18686,.F.);
#25570=ORIENTED_EDGE('',*,*,#18691,.F.);
#25571=ORIENTED_EDGE('',*,*,#18692,.T.);
#25572=ORIENTED_EDGE('',*,*,#18693,.F.);
#25573=ORIENTED_EDGE('',*,*,#18689,.F.);
#25574=ORIENTED_EDGE('',*,*,#18694,.F.);
#25575=ORIENTED_EDGE('',*,*,#18695,.T.);
#25576=ORIENTED_EDGE('',*,*,#18696,.F.);
#25577=ORIENTED_EDGE('',*,*,#18692,.F.);
#25578=ORIENTED_EDGE('',*,*,#18697,.F.);
#25579=ORIENTED_EDGE('',*,*,#18698,.T.);
#25580=ORIENTED_EDGE('',*,*,#18699,.F.);
#25581=ORIENTED_EDGE('',*,*,#18695,.F.);
#25582=ORIENTED_EDGE('',*,*,#18700,.F.);
#25583=ORIENTED_EDGE('',*,*,#18701,.T.);
#25584=ORIENTED_EDGE('',*,*,#18702,.F.);
#25585=ORIENTED_EDGE('',*,*,#18698,.F.);
#25586=ORIENTED_EDGE('',*,*,#18703,.F.);
#25587=ORIENTED_EDGE('',*,*,#18684,.T.);
#25588=ORIENTED_EDGE('',*,*,#18704,.F.);
#25589=ORIENTED_EDGE('',*,*,#18701,.F.);
#25590=ORIENTED_EDGE('',*,*,#18705,.F.);
#25591=ORIENTED_EDGE('',*,*,#18706,.T.);
#25592=ORIENTED_EDGE('',*,*,#18707,.F.);
#25593=ORIENTED_EDGE('',*,*,#18708,.F.);
#25594=ORIENTED_EDGE('',*,*,#18709,.F.);
#25595=ORIENTED_EDGE('',*,*,#18708,.T.);
#25596=ORIENTED_EDGE('',*,*,#18710,.F.);
#25597=ORIENTED_EDGE('',*,*,#18711,.F.);
#25598=ORIENTED_EDGE('',*,*,#18712,.F.);
#25599=ORIENTED_EDGE('',*,*,#18711,.T.);
#25600=ORIENTED_EDGE('',*,*,#18713,.F.);
#25601=ORIENTED_EDGE('',*,*,#18714,.F.);
#25602=ORIENTED_EDGE('',*,*,#18715,.F.);
#25603=ORIENTED_EDGE('',*,*,#18714,.T.);
#25604=ORIENTED_EDGE('',*,*,#18716,.F.);
#25605=ORIENTED_EDGE('',*,*,#18717,.F.);
#25606=ORIENTED_EDGE('',*,*,#18718,.F.);
#25607=ORIENTED_EDGE('',*,*,#18717,.T.);
#25608=ORIENTED_EDGE('',*,*,#18719,.F.);
#25609=ORIENTED_EDGE('',*,*,#18720,.F.);
#25610=ORIENTED_EDGE('',*,*,#18721,.F.);
#25611=ORIENTED_EDGE('',*,*,#18720,.T.);
#25612=ORIENTED_EDGE('',*,*,#18722,.F.);
#25613=ORIENTED_EDGE('',*,*,#18723,.F.);
#25614=ORIENTED_EDGE('',*,*,#18724,.F.);
#25615=ORIENTED_EDGE('',*,*,#18723,.T.);
#25616=ORIENTED_EDGE('',*,*,#18725,.F.);
#25617=ORIENTED_EDGE('',*,*,#18726,.F.);
#25618=ORIENTED_EDGE('',*,*,#18727,.F.);
#25619=ORIENTED_EDGE('',*,*,#18726,.T.);
#25620=ORIENTED_EDGE('',*,*,#18728,.F.);
#25621=ORIENTED_EDGE('',*,*,#18706,.F.);
#25622=ORIENTED_EDGE('',*,*,#18727,.T.);
#25623=ORIENTED_EDGE('',*,*,#18705,.T.);
#25624=ORIENTED_EDGE('',*,*,#18709,.T.);
#25625=ORIENTED_EDGE('',*,*,#18712,.T.);
#25626=ORIENTED_EDGE('',*,*,#18715,.T.);
#25627=ORIENTED_EDGE('',*,*,#18718,.T.);
#25628=ORIENTED_EDGE('',*,*,#18721,.T.);
#25629=ORIENTED_EDGE('',*,*,#18724,.T.);
#25630=ORIENTED_EDGE('',*,*,#18681,.T.);
#25631=ORIENTED_EDGE('',*,*,#18703,.T.);
#25632=ORIENTED_EDGE('',*,*,#18700,.T.);
#25633=ORIENTED_EDGE('',*,*,#18697,.T.);
#25634=ORIENTED_EDGE('',*,*,#18694,.T.);
#25635=ORIENTED_EDGE('',*,*,#18691,.T.);
#25636=ORIENTED_EDGE('',*,*,#18688,.T.);
#25637=ORIENTED_EDGE('',*,*,#18685,.T.);
#25638=ORIENTED_EDGE('',*,*,#18728,.T.);
#25639=ORIENTED_EDGE('',*,*,#18725,.T.);
#25640=ORIENTED_EDGE('',*,*,#18722,.T.);
#25641=ORIENTED_EDGE('',*,*,#18719,.T.);
#25642=ORIENTED_EDGE('',*,*,#18716,.T.);
#25643=ORIENTED_EDGE('',*,*,#18713,.T.);
#25644=ORIENTED_EDGE('',*,*,#18710,.T.);
#25645=ORIENTED_EDGE('',*,*,#18707,.T.);
#25646=ORIENTED_EDGE('',*,*,#18683,.T.);
#25647=ORIENTED_EDGE('',*,*,#18687,.T.);
#25648=ORIENTED_EDGE('',*,*,#18690,.T.);
#25649=ORIENTED_EDGE('',*,*,#18693,.T.);
#25650=ORIENTED_EDGE('',*,*,#18696,.T.);
#25651=ORIENTED_EDGE('',*,*,#18699,.T.);
#25652=ORIENTED_EDGE('',*,*,#18702,.T.);
#25653=ORIENTED_EDGE('',*,*,#18704,.T.);
#31428=PLANE('',#35192);
#31429=PLANE('',#35196);
#31430=PLANE('',#35200);
#31431=PLANE('',#35204);
#31432=PLANE('',#35208);
#31433=PLANE('',#35212);
#31434=PLANE('',#35216);
#31435=PLANE('',#35220);
#31436=PLANE('',#35224);
#31437=PLANE('',#35225);
#31438=PLANE('',#35226);
#31439=PLANE('',#35230);
#31440=PLANE('',#35234);
#31441=PLANE('',#35238);
#31442=PLANE('',#35242);
#31443=PLANE('',#35246);
#31444=PLANE('',#35250);
#31445=PLANE('',#35254);
#31446=PLANE('',#35258);
#31447=PLANE('',#35259);
#31448=PLANE('',#35260);
#31449=PLANE('',#35264);
#31450=PLANE('',#35268);
#31451=PLANE('',#35272);
#31452=PLANE('',#35276);
#31453=PLANE('',#35280);
#31454=PLANE('',#35284);
#31455=PLANE('',#35288);
#31456=PLANE('',#35292);
#31457=PLANE('',#35293);
#31458=PLANE('',#35294);
#31459=PLANE('',#35298);
#31460=PLANE('',#35302);
#31461=PLANE('',#35306);
#31462=PLANE('',#35310);
#31463=PLANE('',#35314);
#31464=PLANE('',#35318);
#31465=PLANE('',#35322);
#31466=PLANE('',#35326);
#31467=PLANE('',#35327);
#31468=PLANE('',#35328);
#31469=PLANE('',#35337);
#31470=PLANE('',#35340);
#31471=PLANE('',#35347);
#31472=PLANE('',#35348);
#31473=PLANE('',#35353);
#31474=PLANE('',#35356);
#31475=PLANE('',#35358);
#31476=PLANE('',#35359);
#31477=PLANE('',#35361);
#31478=PLANE('',#35362);
#31479=PLANE('',#35371);
#31480=PLANE('',#35374);
#31481=PLANE('',#35379);
#31482=PLANE('',#35382);
#31483=PLANE('',#35383);
#31484=PLANE('',#35388);
#31485=PLANE('',#35391);
#31486=PLANE('',#35393);
#31487=PLANE('',#35395);
#31488=PLANE('',#35396);
#31489=PLANE('',#35405);
#31490=PLANE('',#35408);
#31491=PLANE('',#35411);
#31492=PLANE('',#35414);
#31493=PLANE('',#35417);
#31494=PLANE('',#35422);
#31495=PLANE('',#35423);
#31496=PLANE('',#35425);
#31497=PLANE('',#35428);
#31498=PLANE('',#35430);
#31499=PLANE('',#35439);
#31500=PLANE('',#35442);
#31501=PLANE('',#35445);
#31502=PLANE('',#35448);
#31503=PLANE('',#35451);
#31504=PLANE('',#35456);
#31505=PLANE('',#35457);
#31506=PLANE('',#35459);
#31507=PLANE('',#35462);
#31508=PLANE('',#35464);
#31509=PLANE('',#35468);
#31510=PLANE('',#35472);
#31511=PLANE('',#35476);
#31512=PLANE('',#35480);
#31513=PLANE('',#35484);
#31514=PLANE('',#35488);
#31515=PLANE('',#35492);
#31516=PLANE('',#35496);
#31517=PLANE('',#35497);
#31518=PLANE('',#35498);
#31519=PLANE('',#35502);
#31520=PLANE('',#35506);
#31521=PLANE('',#35510);
#31522=PLANE('',#35514);
#31523=PLANE('',#35518);
#31524=PLANE('',#35522);
#31525=PLANE('',#35526);
#31526=PLANE('',#35530);
#31527=PLANE('',#35531);
#31528=PLANE('',#35532);
#31529=PLANE('',#35536);
#31530=PLANE('',#35540);
#31531=PLANE('',#35544);
#31532=PLANE('',#35548);
#31533=PLANE('',#35552);
#31534=PLANE('',#35556);
#31535=PLANE('',#35560);
#31536=PLANE('',#35564);
#31537=PLANE('',#35565);
#31538=PLANE('',#35569);
#31539=PLANE('',#35573);
#31540=PLANE('',#35577);
#31541=PLANE('',#35581);
#31542=PLANE('',#35585);
#31543=PLANE('',#35589);
#31544=PLANE('',#35593);
#31545=PLANE('',#35597);
#31546=PLANE('',#35598);
#31547=PLANE('',#35599);
#31548=PLANE('',#35603);
#31549=PLANE('',#35607);
#31550=PLANE('',#35611);
#31551=PLANE('',#35615);
#31552=PLANE('',#35619);
#31553=PLANE('',#35623);
#31554=PLANE('',#35627);
#31555=PLANE('',#35631);
#31556=PLANE('',#35632);
#31557=PLANE('',#35633);
#31558=PLANE('',#35637);
#31559=PLANE('',#35641);
#31560=PLANE('',#35645);
#31561=PLANE('',#35649);
#31562=PLANE('',#35653);
#31563=PLANE('',#35657);
#31564=PLANE('',#35661);
#31565=PLANE('',#35665);
#31566=PLANE('',#35666);
#31567=PLANE('',#35667);
#31568=PLANE('',#35671);
#31569=PLANE('',#35675);
#31570=PLANE('',#35679);
#31571=PLANE('',#35683);
#31572=PLANE('',#35687);
#31573=PLANE('',#35691);
#31574=PLANE('',#35695);
#31575=PLANE('',#35699);
#31576=PLANE('',#35700);
#31577=PLANE('',#35701);
#32487=ADVANCED_FACE('',(#4806),#31428,.F.);
#32488=ADVANCED_FACE('',(#4807),#1191,.F.);
#32489=ADVANCED_FACE('',(#4808),#31429,.F.);
#32490=ADVANCED_FACE('',(#4809),#1192,.F.);
#32491=ADVANCED_FACE('',(#4810),#31430,.T.);
#32492=ADVANCED_FACE('',(#4811),#1193,.T.);
#32493=ADVANCED_FACE('',(#4812),#31431,.T.);
#32494=ADVANCED_FACE('',(#4813),#1194,.T.);
#32495=ADVANCED_FACE('',(#4814),#31432,.F.);
#32496=ADVANCED_FACE('',(#4815),#1195,.F.);
#32497=ADVANCED_FACE('',(#4816),#31433,.F.);
#32498=ADVANCED_FACE('',(#4817),#1196,.F.);
#32499=ADVANCED_FACE('',(#4818),#31434,.T.);
#32500=ADVANCED_FACE('',(#4819),#1197,.T.);
#32501=ADVANCED_FACE('',(#4820),#31435,.T.);
#32502=ADVANCED_FACE('',(#4821),#1198,.T.);
#32503=ADVANCED_FACE('',(#4822,#1978),#31436,.F.);
#32504=ADVANCED_FACE('',(#4823,#1979),#31437,.T.);
#32505=ADVANCED_FACE('',(#4824),#31438,.F.);
#32506=ADVANCED_FACE('',(#4825),#1199,.F.);
#32507=ADVANCED_FACE('',(#4826),#31439,.F.);
#32508=ADVANCED_FACE('',(#4827),#1200,.F.);
#32509=ADVANCED_FACE('',(#4828),#31440,.T.);
#32510=ADVANCED_FACE('',(#4829),#1201,.T.);
#32511=ADVANCED_FACE('',(#4830),#31441,.T.);
#32512=ADVANCED_FACE('',(#4831),#1202,.T.);
#32513=ADVANCED_FACE('',(#4832),#31442,.F.);
#32514=ADVANCED_FACE('',(#4833),#1203,.F.);
#32515=ADVANCED_FACE('',(#4834),#31443,.F.);
#32516=ADVANCED_FACE('',(#4835),#1204,.F.);
#32517=ADVANCED_FACE('',(#4836),#31444,.T.);
#32518=ADVANCED_FACE('',(#4837),#1205,.T.);
#32519=ADVANCED_FACE('',(#4838),#31445,.T.);
#32520=ADVANCED_FACE('',(#4839),#1206,.T.);
#32521=ADVANCED_FACE('',(#4840,#1980),#31446,.F.);
#32522=ADVANCED_FACE('',(#4841,#1981),#31447,.T.);
#32523=ADVANCED_FACE('',(#4842),#31448,.F.);
#32524=ADVANCED_FACE('',(#4843),#1207,.F.);
#32525=ADVANCED_FACE('',(#4844),#31449,.F.);
#32526=ADVANCED_FACE('',(#4845),#1208,.F.);
#32527=ADVANCED_FACE('',(#4846),#31450,.T.);
#32528=ADVANCED_FACE('',(#4847),#1209,.T.);
#32529=ADVANCED_FACE('',(#4848),#31451,.T.);
#32530=ADVANCED_FACE('',(#4849),#1210,.T.);
#32531=ADVANCED_FACE('',(#4850),#31452,.F.);
#32532=ADVANCED_FACE('',(#4851),#1211,.F.);
#32533=ADVANCED_FACE('',(#4852),#31453,.F.);
#32534=ADVANCED_FACE('',(#4853),#1212,.F.);
#32535=ADVANCED_FACE('',(#4854),#31454,.T.);
#32536=ADVANCED_FACE('',(#4855),#1213,.T.);
#32537=ADVANCED_FACE('',(#4856),#31455,.T.);
#32538=ADVANCED_FACE('',(#4857),#1214,.T.);
#32539=ADVANCED_FACE('',(#4858,#1982),#31456,.F.);
#32540=ADVANCED_FACE('',(#4859,#1983),#31457,.T.);
#32541=ADVANCED_FACE('',(#4860),#31458,.F.);
#32542=ADVANCED_FACE('',(#4861),#1215,.F.);
#32543=ADVANCED_FACE('',(#4862),#31459,.F.);
#32544=ADVANCED_FACE('',(#4863),#1216,.F.);
#32545=ADVANCED_FACE('',(#4864),#31460,.T.);
#32546=ADVANCED_FACE('',(#4865),#1217,.T.);
#32547=ADVANCED_FACE('',(#4866),#31461,.T.);
#32548=ADVANCED_FACE('',(#4867),#1218,.T.);
#32549=ADVANCED_FACE('',(#4868),#31462,.F.);
#32550=ADVANCED_FACE('',(#4869),#1219,.F.);
#32551=ADVANCED_FACE('',(#4870),#31463,.F.);
#32552=ADVANCED_FACE('',(#4871),#1220,.F.);
#32553=ADVANCED_FACE('',(#4872),#31464,.T.);
#32554=ADVANCED_FACE('',(#4873),#1221,.T.);
#32555=ADVANCED_FACE('',(#4874),#31465,.T.);
#32556=ADVANCED_FACE('',(#4875),#1222,.T.);
#32557=ADVANCED_FACE('',(#4876,#1984),#31466,.F.);
#32558=ADVANCED_FACE('',(#4877,#1985),#31467,.T.);
#32559=ADVANCED_FACE('',(#4878,#1986),#31468,.F.);
#32560=ADVANCED_FACE('',(#4879),#31469,.F.);
#32561=ADVANCED_FACE('',(#4880),#1223,.F.);
#32562=ADVANCED_FACE('',(#4881),#31470,.F.);
#32563=ADVANCED_FACE('',(#4882),#1224,.F.);
#32564=ADVANCED_FACE('',(#4883),#1225,.T.);
#32565=ADVANCED_FACE('',(#4884),#1226,.T.);
#32566=ADVANCED_FACE('',(#4885),#31471,.T.);
#32567=ADVANCED_FACE('',(#4886,#1987),#31472,.F.);
#32568=ADVANCED_FACE('',(#4887),#31473,.F.);
#32569=ADVANCED_FACE('',(#4888),#1227,.T.);
#32570=ADVANCED_FACE('',(#4889),#1228,.F.);
#32571=ADVANCED_FACE('',(#4890),#31474,.F.);
#32572=ADVANCED_FACE('',(#4891),#1229,.F.);
#32573=ADVANCED_FACE('',(#4892),#31475,.T.);
#32574=ADVANCED_FACE('',(#4893),#31476,.T.);
#32575=ADVANCED_FACE('',(#4894),#1230,.T.);
#32576=ADVANCED_FACE('',(#4895),#31477,.T.);
#32577=ADVANCED_FACE('',(#4896,#1988),#31478,.F.);
#32578=ADVANCED_FACE('',(#4897),#31479,.F.);
#32579=ADVANCED_FACE('',(#4898),#1231,.F.);
#32580=ADVANCED_FACE('',(#4899),#31480,.F.);
#32581=ADVANCED_FACE('',(#4900),#1232,.F.);
#32582=ADVANCED_FACE('',(#4901),#1233,.T.);
#32583=ADVANCED_FACE('',(#4902),#31481,.T.);
#32584=ADVANCED_FACE('',(#4903),#1234,.T.);
#32585=ADVANCED_FACE('',(#4904),#31482,.T.);
#32586=ADVANCED_FACE('',(#4905,#1989),#31483,.F.);
#32587=ADVANCED_FACE('',(#4906),#31484,.F.);
#32588=ADVANCED_FACE('',(#4907),#1235,.T.);
#32589=ADVANCED_FACE('',(#4908),#1236,.F.);
#32590=ADVANCED_FACE('',(#4909),#31485,.F.);
#32591=ADVANCED_FACE('',(#4910),#1237,.F.);
#32592=ADVANCED_FACE('',(#4911),#31486,.T.);
#32593=ADVANCED_FACE('',(#4912),#1238,.T.);
#32594=ADVANCED_FACE('',(#4913),#31487,.T.);
#32595=ADVANCED_FACE('',(#4914,#1990),#31488,.F.);
#32596=ADVANCED_FACE('',(#4915),#31489,.F.);
#32597=ADVANCED_FACE('',(#4916),#1239,.F.);
#32598=ADVANCED_FACE('',(#4917),#31490,.F.);
#32599=ADVANCED_FACE('',(#4918),#1240,.F.);
#32600=ADVANCED_FACE('',(#4919),#31491,.T.);
#32601=ADVANCED_FACE('',(#4920),#1241,.T.);
#32602=ADVANCED_FACE('',(#4921),#31492,.T.);
#32603=ADVANCED_FACE('',(#4922),#1242,.T.);
#32604=ADVANCED_FACE('',(#4923,#1991),#31493,.F.);
#32605=ADVANCED_FACE('',(#4924),#31494,.F.);
#32606=ADVANCED_FACE('',(#4925),#31495,.T.);
#32607=ADVANCED_FACE('',(#4926),#1243,.F.);
#32608=ADVANCED_FACE('',(#4927),#31496,.F.);
#32609=ADVANCED_FACE('',(#4928),#1244,.F.);
#32610=ADVANCED_FACE('',(#4929),#1245,.T.);
#32611=ADVANCED_FACE('',(#4930),#31497,.T.);
#32612=ADVANCED_FACE('',(#4931),#1246,.T.);
#32613=ADVANCED_FACE('',(#4932,#1992),#31498,.F.);
#32614=ADVANCED_FACE('',(#4933),#31499,.F.);
#32615=ADVANCED_FACE('',(#4934),#1247,.F.);
#32616=ADVANCED_FACE('',(#4935),#31500,.F.);
#32617=ADVANCED_FACE('',(#4936),#1248,.F.);
#32618=ADVANCED_FACE('',(#4937),#31501,.T.);
#32619=ADVANCED_FACE('',(#4938),#1249,.T.);
#32620=ADVANCED_FACE('',(#4939),#31502,.T.);
#32621=ADVANCED_FACE('',(#4940),#1250,.T.);
#32622=ADVANCED_FACE('',(#4941,#1993),#31503,.F.);
#32623=ADVANCED_FACE('',(#4942),#31504,.F.);
#32624=ADVANCED_FACE('',(#4943),#31505,.T.);
#32625=ADVANCED_FACE('',(#4944),#1251,.F.);
#32626=ADVANCED_FACE('',(#4945),#31506,.F.);
#32627=ADVANCED_FACE('',(#4946),#1252,.F.);
#32628=ADVANCED_FACE('',(#4947),#1253,.T.);
#32629=ADVANCED_FACE('',(#4948),#31507,.T.);
#32630=ADVANCED_FACE('',(#4949),#1254,.T.);
#32631=ADVANCED_FACE('',(#4950),#31508,.F.);
#32632=ADVANCED_FACE('',(#4951),#1255,.F.);
#32633=ADVANCED_FACE('',(#4952),#31509,.F.);
#32634=ADVANCED_FACE('',(#4953),#1256,.F.);
#32635=ADVANCED_FACE('',(#4954),#31510,.T.);
#32636=ADVANCED_FACE('',(#4955),#1257,.T.);
#32637=ADVANCED_FACE('',(#4956),#31511,.T.);
#32638=ADVANCED_FACE('',(#4957),#1258,.T.);
#32639=ADVANCED_FACE('',(#4958),#31512,.F.);
#32640=ADVANCED_FACE('',(#4959),#1259,.F.);
#32641=ADVANCED_FACE('',(#4960),#31513,.F.);
#32642=ADVANCED_FACE('',(#4961),#1260,.F.);
#32643=ADVANCED_FACE('',(#4962),#31514,.T.);
#32644=ADVANCED_FACE('',(#4963),#1261,.T.);
#32645=ADVANCED_FACE('',(#4964),#31515,.T.);
#32646=ADVANCED_FACE('',(#4965),#1262,.T.);
#32647=ADVANCED_FACE('',(#4966,#1994),#31516,.F.);
#32648=ADVANCED_FACE('',(#4967,#1995),#31517,.T.);
#32649=ADVANCED_FACE('',(#4968),#31518,.F.);
#32650=ADVANCED_FACE('',(#4969),#1263,.F.);
#32651=ADVANCED_FACE('',(#4970),#31519,.F.);
#32652=ADVANCED_FACE('',(#4971),#1264,.F.);
#32653=ADVANCED_FACE('',(#4972),#31520,.T.);
#32654=ADVANCED_FACE('',(#4973),#1265,.T.);
#32655=ADVANCED_FACE('',(#4974),#31521,.T.);
#32656=ADVANCED_FACE('',(#4975),#1266,.T.);
#32657=ADVANCED_FACE('',(#4976),#31522,.F.);
#32658=ADVANCED_FACE('',(#4977),#1267,.F.);
#32659=ADVANCED_FACE('',(#4978),#31523,.F.);
#32660=ADVANCED_FACE('',(#4979),#1268,.F.);
#32661=ADVANCED_FACE('',(#4980),#31524,.T.);
#32662=ADVANCED_FACE('',(#4981),#1269,.T.);
#32663=ADVANCED_FACE('',(#4982),#31525,.T.);
#32664=ADVANCED_FACE('',(#4983),#1270,.T.);
#32665=ADVANCED_FACE('',(#4984,#1996),#31526,.F.);
#32666=ADVANCED_FACE('',(#4985,#1997),#31527,.T.);
#32667=ADVANCED_FACE('',(#4986),#31528,.F.);
#32668=ADVANCED_FACE('',(#4987),#1271,.F.);
#32669=ADVANCED_FACE('',(#4988),#31529,.F.);
#32670=ADVANCED_FACE('',(#4989),#1272,.F.);
#32671=ADVANCED_FACE('',(#4990),#31530,.T.);
#32672=ADVANCED_FACE('',(#4991),#1273,.T.);
#32673=ADVANCED_FACE('',(#4992),#31531,.T.);
#32674=ADVANCED_FACE('',(#4993),#1274,.T.);
#32675=ADVANCED_FACE('',(#4994),#31532,.F.);
#32676=ADVANCED_FACE('',(#4995),#1275,.F.);
#32677=ADVANCED_FACE('',(#4996),#31533,.F.);
#32678=ADVANCED_FACE('',(#4997),#1276,.F.);
#32679=ADVANCED_FACE('',(#4998),#31534,.T.);
#32680=ADVANCED_FACE('',(#4999),#1277,.T.);
#32681=ADVANCED_FACE('',(#5000),#31535,.T.);
#32682=ADVANCED_FACE('',(#5001),#1278,.T.);
#32683=ADVANCED_FACE('',(#5002,#1998),#31536,.F.);
#32684=ADVANCED_FACE('',(#5003,#1999),#31537,.T.);
#32685=ADVANCED_FACE('',(#5004),#1279,.F.);
#32686=ADVANCED_FACE('',(#5005),#31538,.F.);
#32687=ADVANCED_FACE('',(#5006),#1280,.F.);
#32688=ADVANCED_FACE('',(#5007),#31539,.F.);
#32689=ADVANCED_FACE('',(#5008),#1281,.F.);
#32690=ADVANCED_FACE('',(#5009),#31540,.F.);
#32691=ADVANCED_FACE('',(#5010),#1282,.F.);
#32692=ADVANCED_FACE('',(#5011),#31541,.F.);
#32693=ADVANCED_FACE('',(#5012),#1283,.T.);
#32694=ADVANCED_FACE('',(#5013),#31542,.T.);
#32695=ADVANCED_FACE('',(#5014),#1284,.T.);
#32696=ADVANCED_FACE('',(#5015),#31543,.T.);
#32697=ADVANCED_FACE('',(#5016),#1285,.T.);
#32698=ADVANCED_FACE('',(#5017),#31544,.T.);
#32699=ADVANCED_FACE('',(#5018),#1286,.T.);
#32700=ADVANCED_FACE('',(#5019),#31545,.T.);
#32701=ADVANCED_FACE('',(#5020,#2000),#31546,.F.);
#32702=ADVANCED_FACE('',(#5021,#2001),#31547,.T.);
#32703=ADVANCED_FACE('',(#5022),#1287,.F.);
#32704=ADVANCED_FACE('',(#5023),#31548,.F.);
#32705=ADVANCED_FACE('',(#5024),#1288,.F.);
#32706=ADVANCED_FACE('',(#5025),#31549,.F.);
#32707=ADVANCED_FACE('',(#5026),#1289,.F.);
#32708=ADVANCED_FACE('',(#5027),#31550,.F.);
#32709=ADVANCED_FACE('',(#5028),#1290,.F.);
#32710=ADVANCED_FACE('',(#5029),#31551,.F.);
#32711=ADVANCED_FACE('',(#5030),#1291,.T.);
#32712=ADVANCED_FACE('',(#5031),#31552,.T.);
#32713=ADVANCED_FACE('',(#5032),#1292,.T.);
#32714=ADVANCED_FACE('',(#5033),#31553,.T.);
#32715=ADVANCED_FACE('',(#5034),#1293,.T.);
#32716=ADVANCED_FACE('',(#5035),#31554,.T.);
#32717=ADVANCED_FACE('',(#5036),#1294,.T.);
#32718=ADVANCED_FACE('',(#5037),#31555,.T.);
#32719=ADVANCED_FACE('',(#5038,#2002),#31556,.F.);
#32720=ADVANCED_FACE('',(#5039,#2003),#31557,.T.);
#32721=ADVANCED_FACE('',(#5040),#1295,.F.);
#32722=ADVANCED_FACE('',(#5041),#31558,.F.);
#32723=ADVANCED_FACE('',(#5042),#1296,.F.);
#32724=ADVANCED_FACE('',(#5043),#31559,.F.);
#32725=ADVANCED_FACE('',(#5044),#1297,.F.);
#32726=ADVANCED_FACE('',(#5045),#31560,.F.);
#32727=ADVANCED_FACE('',(#5046),#1298,.F.);
#32728=ADVANCED_FACE('',(#5047),#31561,.F.);
#32729=ADVANCED_FACE('',(#5048),#1299,.T.);
#32730=ADVANCED_FACE('',(#5049),#31562,.T.);
#32731=ADVANCED_FACE('',(#5050),#1300,.T.);
#32732=ADVANCED_FACE('',(#5051),#31563,.T.);
#32733=ADVANCED_FACE('',(#5052),#1301,.T.);
#32734=ADVANCED_FACE('',(#5053),#31564,.T.);
#32735=ADVANCED_FACE('',(#5054),#1302,.T.);
#32736=ADVANCED_FACE('',(#5055),#31565,.T.);
#32737=ADVANCED_FACE('',(#5056,#2004),#31566,.F.);
#32738=ADVANCED_FACE('',(#5057,#2005),#31567,.T.);
#32739=ADVANCED_FACE('',(#5058),#1303,.F.);
#32740=ADVANCED_FACE('',(#5059),#31568,.F.);
#32741=ADVANCED_FACE('',(#5060),#1304,.F.);
#32742=ADVANCED_FACE('',(#5061),#31569,.F.);
#32743=ADVANCED_FACE('',(#5062),#1305,.F.);
#32744=ADVANCED_FACE('',(#5063),#31570,.F.);
#32745=ADVANCED_FACE('',(#5064),#1306,.F.);
#32746=ADVANCED_FACE('',(#5065),#31571,.F.);
#32747=ADVANCED_FACE('',(#5066),#1307,.T.);
#32748=ADVANCED_FACE('',(#5067),#31572,.T.);
#32749=ADVANCED_FACE('',(#5068),#1308,.T.);
#32750=ADVANCED_FACE('',(#5069),#31573,.T.);
#32751=ADVANCED_FACE('',(#5070),#1309,.T.);
#32752=ADVANCED_FACE('',(#5071),#31574,.T.);
#32753=ADVANCED_FACE('',(#5072),#1310,.T.);
#32754=ADVANCED_FACE('',(#5073),#31575,.T.);
#32755=ADVANCED_FACE('',(#5074,#2006),#31576,.F.);
#32756=ADVANCED_FACE('',(#5075,#2007),#31577,.T.);
#33801=CLOSED_SHELL('',(#32487,#32488,#32489,#32490,#32491,#32492,#32493,
#32494,#32495,#32496,#32497,#32498,#32499,#32500,#32501,#32502,#32503,#32504));
#33802=CLOSED_SHELL('',(#32505,#32506,#32507,#32508,#32509,#32510,#32511,
#32512,#32513,#32514,#32515,#32516,#32517,#32518,#32519,#32520,#32521,#32522));
#33803=CLOSED_SHELL('',(#32523,#32524,#32525,#32526,#32527,#32528,#32529,
#32530,#32531,#32532,#32533,#32534,#32535,#32536,#32537,#32538,#32539,#32540));
#33804=CLOSED_SHELL('',(#32541,#32542,#32543,#32544,#32545,#32546,#32547,
#32548,#32549,#32550,#32551,#32552,#32553,#32554,#32555,#32556,#32557,#32558));
#33805=CLOSED_SHELL('',(#32559,#32560,#32561,#32562,#32563,#32564,#32565,
#32566,#32567,#32568,#32569,#32570,#32571,#32572,#32573,#32574,#32575,#32576));
#33806=CLOSED_SHELL('',(#32577,#32578,#32579,#32580,#32581,#32582,#32583,
#32584,#32585,#32586,#32587,#32588,#32589,#32590,#32591,#32592,#32593,#32594));
#33807=CLOSED_SHELL('',(#32595,#32596,#32597,#32598,#32599,#32600,#32601,
#32602,#32603,#32604,#32605,#32606,#32607,#32608,#32609,#32610,#32611,#32612));
#33808=CLOSED_SHELL('',(#32613,#32614,#32615,#32616,#32617,#32618,#32619,
#32620,#32621,#32622,#32623,#32624,#32625,#32626,#32627,#32628,#32629,#32630));
#33809=CLOSED_SHELL('',(#32631,#32632,#32633,#32634,#32635,#32636,#32637,
#32638,#32639,#32640,#32641,#32642,#32643,#32644,#32645,#32646,#32647,#32648));
#33810=CLOSED_SHELL('',(#32649,#32650,#32651,#32652,#32653,#32654,#32655,
#32656,#32657,#32658,#32659,#32660,#32661,#32662,#32663,#32664,#32665,#32666));
#33811=CLOSED_SHELL('',(#32667,#32668,#32669,#32670,#32671,#32672,#32673,
#32674,#32675,#32676,#32677,#32678,#32679,#32680,#32681,#32682,#32683,#32684));
#33812=CLOSED_SHELL('',(#32685,#32686,#32687,#32688,#32689,#32690,#32691,
#32692,#32693,#32694,#32695,#32696,#32697,#32698,#32699,#32700,#32701,#32702));
#33813=CLOSED_SHELL('',(#32703,#32704,#32705,#32706,#32707,#32708,#32709,
#32710,#32711,#32712,#32713,#32714,#32715,#32716,#32717,#32718,#32719,#32720));
#33814=CLOSED_SHELL('',(#32721,#32722,#32723,#32724,#32725,#32726,#32727,
#32728,#32729,#32730,#32731,#32732,#32733,#32734,#32735,#32736,#32737,#32738));
#33815=CLOSED_SHELL('',(#32739,#32740,#32741,#32742,#32743,#32744,#32745,
#32746,#32747,#32748,#32749,#32750,#32751,#32752,#32753,#32754,#32755,#32756));
#35191=AXIS2_PLACEMENT_3D('',#53781,#41079,#41080);
#35192=AXIS2_PLACEMENT_3D('',#53782,#41081,#41082);
#35193=AXIS2_PLACEMENT_3D('',#53791,#41087,#41088);
#35194=AXIS2_PLACEMENT_3D('',#53793,#41089,#41090);
#35195=AXIS2_PLACEMENT_3D('',#53796,#41092,#41093);
#35196=AXIS2_PLACEMENT_3D('',#53797,#41094,#41095);
#35197=AXIS2_PLACEMENT_3D('',#53803,#41099,#41100);
#35198=AXIS2_PLACEMENT_3D('',#53805,#41101,#41102);
#35199=AXIS2_PLACEMENT_3D('',#53808,#41104,#41105);
#35200=AXIS2_PLACEMENT_3D('',#53809,#41106,#41107);
#35201=AXIS2_PLACEMENT_3D('',#53818,#41112,#41113);
#35202=AXIS2_PLACEMENT_3D('',#53820,#41114,#41115);
#35203=AXIS2_PLACEMENT_3D('',#53823,#41117,#41118);
#35204=AXIS2_PLACEMENT_3D('',#53824,#41119,#41120);
#35205=AXIS2_PLACEMENT_3D('',#53830,#41124,#41125);
#35206=AXIS2_PLACEMENT_3D('',#53832,#41126,#41127);
#35207=AXIS2_PLACEMENT_3D('',#53835,#41129,#41130);
#35208=AXIS2_PLACEMENT_3D('',#53836,#41131,#41132);
#35209=AXIS2_PLACEMENT_3D('',#53842,#41136,#41137);
#35210=AXIS2_PLACEMENT_3D('',#53844,#41138,#41139);
#35211=AXIS2_PLACEMENT_3D('',#53846,#41140,#41141);
#35212=AXIS2_PLACEMENT_3D('',#53848,#41143,#41144);
#35213=AXIS2_PLACEMENT_3D('',#53854,#41148,#41149);
#35214=AXIS2_PLACEMENT_3D('',#53855,#41150,#41151);
#35215=AXIS2_PLACEMENT_3D('',#53856,#41152,#41153);
#35216=AXIS2_PLACEMENT_3D('',#53857,#41154,#41155);
#35217=AXIS2_PLACEMENT_3D('',#53863,#41159,#41160);
#35218=AXIS2_PLACEMENT_3D('',#53865,#41161,#41162);
#35219=AXIS2_PLACEMENT_3D('',#53868,#41164,#41165);
#35220=AXIS2_PLACEMENT_3D('',#53869,#41166,#41167);
#35221=AXIS2_PLACEMENT_3D('',#53875,#41171,#41172);
#35222=AXIS2_PLACEMENT_3D('',#53876,#41173,#41174);
#35223=AXIS2_PLACEMENT_3D('',#53877,#41175,#41176);
#35224=AXIS2_PLACEMENT_3D('',#53878,#41177,#41178);
#35225=AXIS2_PLACEMENT_3D('',#53879,#41179,#41180);
#35226=AXIS2_PLACEMENT_3D('',#53880,#41181,#41182);
#35227=AXIS2_PLACEMENT_3D('',#53889,#41187,#41188);
#35228=AXIS2_PLACEMENT_3D('',#53891,#41189,#41190);
#35229=AXIS2_PLACEMENT_3D('',#53894,#41192,#41193);
#35230=AXIS2_PLACEMENT_3D('',#53895,#41194,#41195);
#35231=AXIS2_PLACEMENT_3D('',#53901,#41199,#41200);
#35232=AXIS2_PLACEMENT_3D('',#53903,#41201,#41202);
#35233=AXIS2_PLACEMENT_3D('',#53906,#41204,#41205);
#35234=AXIS2_PLACEMENT_3D('',#53907,#41206,#41207);
#35235=AXIS2_PLACEMENT_3D('',#53916,#41212,#41213);
#35236=AXIS2_PLACEMENT_3D('',#53918,#41214,#41215);
#35237=AXIS2_PLACEMENT_3D('',#53921,#41217,#41218);
#35238=AXIS2_PLACEMENT_3D('',#53922,#41219,#41220);
#35239=AXIS2_PLACEMENT_3D('',#53928,#41224,#41225);
#35240=AXIS2_PLACEMENT_3D('',#53930,#41226,#41227);
#35241=AXIS2_PLACEMENT_3D('',#53933,#41229,#41230);
#35242=AXIS2_PLACEMENT_3D('',#53934,#41231,#41232);
#35243=AXIS2_PLACEMENT_3D('',#53940,#41236,#41237);
#35244=AXIS2_PLACEMENT_3D('',#53942,#41238,#41239);
#35245=AXIS2_PLACEMENT_3D('',#53944,#41240,#41241);
#35246=AXIS2_PLACEMENT_3D('',#53946,#41243,#41244);
#35247=AXIS2_PLACEMENT_3D('',#53952,#41248,#41249);
#35248=AXIS2_PLACEMENT_3D('',#53953,#41250,#41251);
#35249=AXIS2_PLACEMENT_3D('',#53954,#41252,#41253);
#35250=AXIS2_PLACEMENT_3D('',#53955,#41254,#41255);
#35251=AXIS2_PLACEMENT_3D('',#53961,#41259,#41260);
#35252=AXIS2_PLACEMENT_3D('',#53963,#41261,#41262);
#35253=AXIS2_PLACEMENT_3D('',#53966,#41264,#41265);
#35254=AXIS2_PLACEMENT_3D('',#53967,#41266,#41267);
#35255=AXIS2_PLACEMENT_3D('',#53973,#41271,#41272);
#35256=AXIS2_PLACEMENT_3D('',#53974,#41273,#41274);
#35257=AXIS2_PLACEMENT_3D('',#53975,#41275,#41276);
#35258=AXIS2_PLACEMENT_3D('',#53976,#41277,#41278);
#35259=AXIS2_PLACEMENT_3D('',#53977,#41279,#41280);
#35260=AXIS2_PLACEMENT_3D('',#53978,#41281,#41282);
#35261=AXIS2_PLACEMENT_3D('',#53987,#41287,#41288);
#35262=AXIS2_PLACEMENT_3D('',#53989,#41289,#41290);
#35263=AXIS2_PLACEMENT_3D('',#53992,#41292,#41293);
#35264=AXIS2_PLACEMENT_3D('',#53993,#41294,#41295);
#35265=AXIS2_PLACEMENT_3D('',#53999,#41299,#41300);
#35266=AXIS2_PLACEMENT_3D('',#54001,#41301,#41302);
#35267=AXIS2_PLACEMENT_3D('',#54004,#41304,#41305);
#35268=AXIS2_PLACEMENT_3D('',#54005,#41306,#41307);
#35269=AXIS2_PLACEMENT_3D('',#54014,#41312,#41313);
#35270=AXIS2_PLACEMENT_3D('',#54016,#41314,#41315);
#35271=AXIS2_PLACEMENT_3D('',#54019,#41317,#41318);
#35272=AXIS2_PLACEMENT_3D('',#54020,#41319,#41320);
#35273=AXIS2_PLACEMENT_3D('',#54026,#41324,#41325);
#35274=AXIS2_PLACEMENT_3D('',#54028,#41326,#41327);
#35275=AXIS2_PLACEMENT_3D('',#54031,#41329,#41330);
#35276=AXIS2_PLACEMENT_3D('',#54032,#41331,#41332);
#35277=AXIS2_PLACEMENT_3D('',#54038,#41336,#41337);
#35278=AXIS2_PLACEMENT_3D('',#54040,#41338,#41339);
#35279=AXIS2_PLACEMENT_3D('',#54042,#41340,#41341);
#35280=AXIS2_PLACEMENT_3D('',#54044,#41343,#41344);
#35281=AXIS2_PLACEMENT_3D('',#54050,#41348,#41349);
#35282=AXIS2_PLACEMENT_3D('',#54051,#41350,#41351);
#35283=AXIS2_PLACEMENT_3D('',#54052,#41352,#41353);
#35284=AXIS2_PLACEMENT_3D('',#54053,#41354,#41355);
#35285=AXIS2_PLACEMENT_3D('',#54059,#41359,#41360);
#35286=AXIS2_PLACEMENT_3D('',#54061,#41361,#41362);
#35287=AXIS2_PLACEMENT_3D('',#54064,#41364,#41365);
#35288=AXIS2_PLACEMENT_3D('',#54065,#41366,#41367);
#35289=AXIS2_PLACEMENT_3D('',#54071,#41371,#41372);
#35290=AXIS2_PLACEMENT_3D('',#54072,#41373,#41374);
#35291=AXIS2_PLACEMENT_3D('',#54073,#41375,#41376);
#35292=AXIS2_PLACEMENT_3D('',#54074,#41377,#41378);
#35293=AXIS2_PLACEMENT_3D('',#54075,#41379,#41380);
#35294=AXIS2_PLACEMENT_3D('',#54076,#41381,#41382);
#35295=AXIS2_PLACEMENT_3D('',#54085,#41387,#41388);
#35296=AXIS2_PLACEMENT_3D('',#54087,#41389,#41390);
#35297=AXIS2_PLACEMENT_3D('',#54090,#41392,#41393);
#35298=AXIS2_PLACEMENT_3D('',#54091,#41394,#41395);
#35299=AXIS2_PLACEMENT_3D('',#54097,#41399,#41400);
#35300=AXIS2_PLACEMENT_3D('',#54099,#41401,#41402);
#35301=AXIS2_PLACEMENT_3D('',#54102,#41404,#41405);
#35302=AXIS2_PLACEMENT_3D('',#54103,#41406,#41407);
#35303=AXIS2_PLACEMENT_3D('',#54112,#41412,#41413);
#35304=AXIS2_PLACEMENT_3D('',#54114,#41414,#41415);
#35305=AXIS2_PLACEMENT_3D('',#54117,#41417,#41418);
#35306=AXIS2_PLACEMENT_3D('',#54118,#41419,#41420);
#35307=AXIS2_PLACEMENT_3D('',#54124,#41424,#41425);
#35308=AXIS2_PLACEMENT_3D('',#54126,#41426,#41427);
#35309=AXIS2_PLACEMENT_3D('',#54129,#41429,#41430);
#35310=AXIS2_PLACEMENT_3D('',#54130,#41431,#41432);
#35311=AXIS2_PLACEMENT_3D('',#54136,#41436,#41437);
#35312=AXIS2_PLACEMENT_3D('',#54138,#41438,#41439);
#35313=AXIS2_PLACEMENT_3D('',#54140,#41440,#41441);
#35314=AXIS2_PLACEMENT_3D('',#54142,#41443,#41444);
#35315=AXIS2_PLACEMENT_3D('',#54148,#41448,#41449);
#35316=AXIS2_PLACEMENT_3D('',#54149,#41450,#41451);
#35317=AXIS2_PLACEMENT_3D('',#54150,#41452,#41453);
#35318=AXIS2_PLACEMENT_3D('',#54151,#41454,#41455);
#35319=AXIS2_PLACEMENT_3D('',#54157,#41459,#41460);
#35320=AXIS2_PLACEMENT_3D('',#54159,#41461,#41462);
#35321=AXIS2_PLACEMENT_3D('',#54162,#41464,#41465);
#35322=AXIS2_PLACEMENT_3D('',#54163,#41466,#41467);
#35323=AXIS2_PLACEMENT_3D('',#54169,#41471,#41472);
#35324=AXIS2_PLACEMENT_3D('',#54170,#41473,#41474);
#35325=AXIS2_PLACEMENT_3D('',#54171,#41475,#41476);
#35326=AXIS2_PLACEMENT_3D('',#54172,#41477,#41478);
#35327=AXIS2_PLACEMENT_3D('',#54173,#41479,#41480);
#35328=AXIS2_PLACEMENT_3D('',#54174,#41481,#41482);
#35329=AXIS2_PLACEMENT_3D('',#54177,#41483,#41484);
#35330=AXIS2_PLACEMENT_3D('',#54181,#41486,#41487);
#35331=AXIS2_PLACEMENT_3D('',#54185,#41489,#41490);
#35332=AXIS2_PLACEMENT_3D('',#54189,#41492,#41493);
#35333=AXIS2_PLACEMENT_3D('',#54195,#41496,#41497);
#35334=AXIS2_PLACEMENT_3D('',#54199,#41499,#41500);
#35335=AXIS2_PLACEMENT_3D('',#54203,#41502,#41503);
#35336=AXIS2_PLACEMENT_3D('',#54206,#41505,#41506);
#35337=AXIS2_PLACEMENT_3D('',#54207,#41507,#41508);
#35338=AXIS2_PLACEMENT_3D('',#54213,#41512,#41513);
#35339=AXIS2_PLACEMENT_3D('',#54216,#41515,#41516);
#35340=AXIS2_PLACEMENT_3D('',#54217,#41517,#41518);
#35341=AXIS2_PLACEMENT_3D('',#54221,#41521,#41522);
#35342=AXIS2_PLACEMENT_3D('',#54224,#41524,#41525);
#35343=AXIS2_PLACEMENT_3D('',#54225,#41526,#41527);
#35344=AXIS2_PLACEMENT_3D('',#54229,#41529,#41530);
#35345=AXIS2_PLACEMENT_3D('',#54231,#41532,#41533);
#35346=AXIS2_PLACEMENT_3D('',#54235,#41535,#41536);
#35347=AXIS2_PLACEMENT_3D('',#54237,#41538,#41539);
#35348=AXIS2_PLACEMENT_3D('',#54241,#41542,#41543);
#35349=AXIS2_PLACEMENT_3D('',#54244,#41545,#41546);
#35350=AXIS2_PLACEMENT_3D('',#54248,#41548,#41549);
#35351=AXIS2_PLACEMENT_3D('',#54253,#41552,#41553);
#35352=AXIS2_PLACEMENT_3D('',#54256,#41555,#41556);
#35353=AXIS2_PLACEMENT_3D('',#54257,#41557,#41558);
#35354=AXIS2_PLACEMENT_3D('',#54259,#41560,#41561);
#35355=AXIS2_PLACEMENT_3D('',#54261,#41563,#41564);
#35356=AXIS2_PLACEMENT_3D('',#54263,#41566,#41567);
#35357=AXIS2_PLACEMENT_3D('',#54265,#41569,#41570);
#35358=AXIS2_PLACEMENT_3D('',#54266,#41571,#41572);
#35359=AXIS2_PLACEMENT_3D('',#54267,#41573,#41574);
#35360=AXIS2_PLACEMENT_3D('',#54269,#41576,#41577);
#35361=AXIS2_PLACEMENT_3D('',#54271,#41579,#41580);
#35362=AXIS2_PLACEMENT_3D('',#54272,#41581,#41582);
#35363=AXIS2_PLACEMENT_3D('',#54275,#41583,#41584);
#35364=AXIS2_PLACEMENT_3D('',#54279,#41586,#41587);
#35365=AXIS2_PLACEMENT_3D('',#54283,#41589,#41590);
#35366=AXIS2_PLACEMENT_3D('',#54287,#41592,#41593);
#35367=AXIS2_PLACEMENT_3D('',#54293,#41596,#41597);
#35368=AXIS2_PLACEMENT_3D('',#54297,#41599,#41600);
#35369=AXIS2_PLACEMENT_3D('',#54301,#41602,#41603);
#35370=AXIS2_PLACEMENT_3D('',#54304,#41605,#41606);
#35371=AXIS2_PLACEMENT_3D('',#54305,#41607,#41608);
#35372=AXIS2_PLACEMENT_3D('',#54311,#41612,#41613);
#35373=AXIS2_PLACEMENT_3D('',#54314,#41615,#41616);
#35374=AXIS2_PLACEMENT_3D('',#54315,#41617,#41618);
#35375=AXIS2_PLACEMENT_3D('',#54319,#41621,#41622);
#35376=AXIS2_PLACEMENT_3D('',#54322,#41624,#41625);
#35377=AXIS2_PLACEMENT_3D('',#54323,#41626,#41627);
#35378=AXIS2_PLACEMENT_3D('',#54327,#41629,#41630);
#35379=AXIS2_PLACEMENT_3D('',#54329,#41632,#41633);
#35380=AXIS2_PLACEMENT_3D('',#54333,#41636,#41637);
#35381=AXIS2_PLACEMENT_3D('',#54336,#41639,#41640);
#35382=AXIS2_PLACEMENT_3D('',#54337,#41641,#41642);
#35383=AXIS2_PLACEMENT_3D('',#54341,#41645,#41646);
#35384=AXIS2_PLACEMENT_3D('',#54343,#41647,#41648);
#35385=AXIS2_PLACEMENT_3D('',#54347,#41650,#41651);
#35386=AXIS2_PLACEMENT_3D('',#54352,#41654,#41655);
#35387=AXIS2_PLACEMENT_3D('',#54355,#41657,#41658);
#35388=AXIS2_PLACEMENT_3D('',#54356,#41659,#41660);
#35389=AXIS2_PLACEMENT_3D('',#54358,#41662,#41663);
#35390=AXIS2_PLACEMENT_3D('',#54360,#41665,#41666);
#35391=AXIS2_PLACEMENT_3D('',#54362,#41668,#41669);
#35392=AXIS2_PLACEMENT_3D('',#54364,#41671,#41672);
#35393=AXIS2_PLACEMENT_3D('',#54365,#41673,#41674);
#35394=AXIS2_PLACEMENT_3D('',#54367,#41676,#41677);
#35395=AXIS2_PLACEMENT_3D('',#54369,#41679,#41680);
#35396=AXIS2_PLACEMENT_3D('',#54370,#41681,#41682);
#35397=AXIS2_PLACEMENT_3D('',#54375,#41684,#41685);
#35398=AXIS2_PLACEMENT_3D('',#54379,#41687,#41688);
#35399=AXIS2_PLACEMENT_3D('',#54383,#41690,#41691);
#35400=AXIS2_PLACEMENT_3D('',#54386,#41693,#41694);
#35401=AXIS2_PLACEMENT_3D('',#54391,#41696,#41697);
#35402=AXIS2_PLACEMENT_3D('',#54395,#41699,#41700);
#35403=AXIS2_PLACEMENT_3D('',#54399,#41702,#41703);
#35404=AXIS2_PLACEMENT_3D('',#54402,#41705,#41706);
#35405=AXIS2_PLACEMENT_3D('',#54403,#41707,#41708);
#35406=AXIS2_PLACEMENT_3D('',#54409,#41712,#41713);
#35407=AXIS2_PLACEMENT_3D('',#54412,#41715,#41716);
#35408=AXIS2_PLACEMENT_3D('',#54413,#41717,#41718);
#35409=AXIS2_PLACEMENT_3D('',#54417,#41721,#41722);
#35410=AXIS2_PLACEMENT_3D('',#54420,#41724,#41725);
#35411=AXIS2_PLACEMENT_3D('',#54421,#41726,#41727);
#35412=AXIS2_PLACEMENT_3D('',#54427,#41731,#41732);
#35413=AXIS2_PLACEMENT_3D('',#54430,#41734,#41735);
#35414=AXIS2_PLACEMENT_3D('',#54431,#41736,#41737);
#35415=AXIS2_PLACEMENT_3D('',#54435,#41740,#41741);
#35416=AXIS2_PLACEMENT_3D('',#54438,#41743,#41744);
#35417=AXIS2_PLACEMENT_3D('',#54439,#41745,#41746);
#35418=AXIS2_PLACEMENT_3D('',#54443,#41748,#41749);
#35419=AXIS2_PLACEMENT_3D('',#54446,#41751,#41752);
#35420=AXIS2_PLACEMENT_3D('',#54450,#41754,#41755);
#35421=AXIS2_PLACEMENT_3D('',#54453,#41757,#41758);
#35422=AXIS2_PLACEMENT_3D('',#54454,#41759,#41760);
#35423=AXIS2_PLACEMENT_3D('',#54456,#41762,#41763);
#35424=AXIS2_PLACEMENT_3D('',#54458,#41765,#41766);
#35425=AXIS2_PLACEMENT_3D('',#54460,#41768,#41769);
#35426=AXIS2_PLACEMENT_3D('',#54462,#41771,#41772);
#35427=AXIS2_PLACEMENT_3D('',#54463,#41773,#41774);
#35428=AXIS2_PLACEMENT_3D('',#54465,#41776,#41777);
#35429=AXIS2_PLACEMENT_3D('',#54467,#41779,#41780);
#35430=AXIS2_PLACEMENT_3D('',#54468,#41781,#41782);
#35431=AXIS2_PLACEMENT_3D('',#54473,#41784,#41785);
#35432=AXIS2_PLACEMENT_3D('',#54477,#41787,#41788);
#35433=AXIS2_PLACEMENT_3D('',#54481,#41790,#41791);
#35434=AXIS2_PLACEMENT_3D('',#54484,#41793,#41794);
#35435=AXIS2_PLACEMENT_3D('',#54489,#41796,#41797);
#35436=AXIS2_PLACEMENT_3D('',#54493,#41799,#41800);
#35437=AXIS2_PLACEMENT_3D('',#54497,#41802,#41803);
#35438=AXIS2_PLACEMENT_3D('',#54500,#41805,#41806);
#35439=AXIS2_PLACEMENT_3D('',#54501,#41807,#41808);
#35440=AXIS2_PLACEMENT_3D('',#54507,#41812,#41813);
#35441=AXIS2_PLACEMENT_3D('',#54510,#41815,#41816);
#35442=AXIS2_PLACEMENT_3D('',#54511,#41817,#41818);
#35443=AXIS2_PLACEMENT_3D('',#54515,#41821,#41822);
#35444=AXIS2_PLACEMENT_3D('',#54518,#41824,#41825);
#35445=AXIS2_PLACEMENT_3D('',#54519,#41826,#41827);
#35446=AXIS2_PLACEMENT_3D('',#54525,#41831,#41832);
#35447=AXIS2_PLACEMENT_3D('',#54528,#41834,#41835);
#35448=AXIS2_PLACEMENT_3D('',#54529,#41836,#41837);
#35449=AXIS2_PLACEMENT_3D('',#54533,#41840,#41841);
#35450=AXIS2_PLACEMENT_3D('',#54536,#41843,#41844);
#35451=AXIS2_PLACEMENT_3D('',#54537,#41845,#41846);
#35452=AXIS2_PLACEMENT_3D('',#54541,#41848,#41849);
#35453=AXIS2_PLACEMENT_3D('',#54544,#41851,#41852);
#35454=AXIS2_PLACEMENT_3D('',#54548,#41854,#41855);
#35455=AXIS2_PLACEMENT_3D('',#54551,#41857,#41858);
#35456=AXIS2_PLACEMENT_3D('',#54552,#41859,#41860);
#35457=AXIS2_PLACEMENT_3D('',#54554,#41862,#41863);
#35458=AXIS2_PLACEMENT_3D('',#54556,#41865,#41866);
#35459=AXIS2_PLACEMENT_3D('',#54558,#41868,#41869);
#35460=AXIS2_PLACEMENT_3D('',#54560,#41871,#41872);
#35461=AXIS2_PLACEMENT_3D('',#54561,#41873,#41874);
#35462=AXIS2_PLACEMENT_3D('',#54563,#41876,#41877);
#35463=AXIS2_PLACEMENT_3D('',#54565,#41879,#41880);
#35464=AXIS2_PLACEMENT_3D('',#54566,#41881,#41882);
#35465=AXIS2_PLACEMENT_3D('',#54575,#41887,#41888);
#35466=AXIS2_PLACEMENT_3D('',#54577,#41889,#41890);
#35467=AXIS2_PLACEMENT_3D('',#54580,#41892,#41893);
#35468=AXIS2_PLACEMENT_3D('',#54581,#41894,#41895);
#35469=AXIS2_PLACEMENT_3D('',#54587,#41899,#41900);
#35470=AXIS2_PLACEMENT_3D('',#54589,#41901,#41902);
#35471=AXIS2_PLACEMENT_3D('',#54592,#41904,#41905);
#35472=AXIS2_PLACEMENT_3D('',#54593,#41906,#41907);
#35473=AXIS2_PLACEMENT_3D('',#54602,#41912,#41913);
#35474=AXIS2_PLACEMENT_3D('',#54604,#41914,#41915);
#35475=AXIS2_PLACEMENT_3D('',#54607,#41917,#41918);
#35476=AXIS2_PLACEMENT_3D('',#54608,#41919,#41920);
#35477=AXIS2_PLACEMENT_3D('',#54614,#41924,#41925);
#35478=AXIS2_PLACEMENT_3D('',#54616,#41926,#41927);
#35479=AXIS2_PLACEMENT_3D('',#54619,#41929,#41930);
#35480=AXIS2_PLACEMENT_3D('',#54620,#41931,#41932);
#35481=AXIS2_PLACEMENT_3D('',#54626,#41936,#41937);
#35482=AXIS2_PLACEMENT_3D('',#54628,#41938,#41939);
#35483=AXIS2_PLACEMENT_3D('',#54630,#41940,#41941);
#35484=AXIS2_PLACEMENT_3D('',#54632,#41943,#41944);
#35485=AXIS2_PLACEMENT_3D('',#54638,#41948,#41949);
#35486=AXIS2_PLACEMENT_3D('',#54639,#41950,#41951);
#35487=AXIS2_PLACEMENT_3D('',#54640,#41952,#41953);
#35488=AXIS2_PLACEMENT_3D('',#54641,#41954,#41955);
#35489=AXIS2_PLACEMENT_3D('',#54647,#41959,#41960);
#35490=AXIS2_PLACEMENT_3D('',#54649,#41961,#41962);
#35491=AXIS2_PLACEMENT_3D('',#54652,#41964,#41965);
#35492=AXIS2_PLACEMENT_3D('',#54653,#41966,#41967);
#35493=AXIS2_PLACEMENT_3D('',#54659,#41971,#41972);
#35494=AXIS2_PLACEMENT_3D('',#54660,#41973,#41974);
#35495=AXIS2_PLACEMENT_3D('',#54661,#41975,#41976);
#35496=AXIS2_PLACEMENT_3D('',#54662,#41977,#41978);
#35497=AXIS2_PLACEMENT_3D('',#54663,#41979,#41980);
#35498=AXIS2_PLACEMENT_3D('',#54664,#41981,#41982);
#35499=AXIS2_PLACEMENT_3D('',#54673,#41987,#41988);
#35500=AXIS2_PLACEMENT_3D('',#54675,#41989,#41990);
#35501=AXIS2_PLACEMENT_3D('',#54678,#41992,#41993);
#35502=AXIS2_PLACEMENT_3D('',#54679,#41994,#41995);
#35503=AXIS2_PLACEMENT_3D('',#54685,#41999,#42000);
#35504=AXIS2_PLACEMENT_3D('',#54687,#42001,#42002);
#35505=AXIS2_PLACEMENT_3D('',#54690,#42004,#42005);
#35506=AXIS2_PLACEMENT_3D('',#54691,#42006,#42007);
#35507=AXIS2_PLACEMENT_3D('',#54700,#42012,#42013);
#35508=AXIS2_PLACEMENT_3D('',#54702,#42014,#42015);
#35509=AXIS2_PLACEMENT_3D('',#54705,#42017,#42018);
#35510=AXIS2_PLACEMENT_3D('',#54706,#42019,#42020);
#35511=AXIS2_PLACEMENT_3D('',#54712,#42024,#42025);
#35512=AXIS2_PLACEMENT_3D('',#54714,#42026,#42027);
#35513=AXIS2_PLACEMENT_3D('',#54717,#42029,#42030);
#35514=AXIS2_PLACEMENT_3D('',#54718,#42031,#42032);
#35515=AXIS2_PLACEMENT_3D('',#54724,#42036,#42037);
#35516=AXIS2_PLACEMENT_3D('',#54726,#42038,#42039);
#35517=AXIS2_PLACEMENT_3D('',#54728,#42040,#42041);
#35518=AXIS2_PLACEMENT_3D('',#54730,#42043,#42044);
#35519=AXIS2_PLACEMENT_3D('',#54736,#42048,#42049);
#35520=AXIS2_PLACEMENT_3D('',#54737,#42050,#42051);
#35521=AXIS2_PLACEMENT_3D('',#54738,#42052,#42053);
#35522=AXIS2_PLACEMENT_3D('',#54739,#42054,#42055);
#35523=AXIS2_PLACEMENT_3D('',#54745,#42059,#42060);
#35524=AXIS2_PLACEMENT_3D('',#54747,#42061,#42062);
#35525=AXIS2_PLACEMENT_3D('',#54750,#42064,#42065);
#35526=AXIS2_PLACEMENT_3D('',#54751,#42066,#42067);
#35527=AXIS2_PLACEMENT_3D('',#54757,#42071,#42072);
#35528=AXIS2_PLACEMENT_3D('',#54758,#42073,#42074);
#35529=AXIS2_PLACEMENT_3D('',#54759,#42075,#42076);
#35530=AXIS2_PLACEMENT_3D('',#54760,#42077,#42078);
#35531=AXIS2_PLACEMENT_3D('',#54761,#42079,#42080);
#35532=AXIS2_PLACEMENT_3D('',#54762,#42081,#42082);
#35533=AXIS2_PLACEMENT_3D('',#54771,#42087,#42088);
#35534=AXIS2_PLACEMENT_3D('',#54773,#42089,#42090);
#35535=AXIS2_PLACEMENT_3D('',#54776,#42092,#42093);
#35536=AXIS2_PLACEMENT_3D('',#54777,#42094,#42095);
#35537=AXIS2_PLACEMENT_3D('',#54783,#42099,#42100);
#35538=AXIS2_PLACEMENT_3D('',#54785,#42101,#42102);
#35539=AXIS2_PLACEMENT_3D('',#54788,#42104,#42105);
#35540=AXIS2_PLACEMENT_3D('',#54789,#42106,#42107);
#35541=AXIS2_PLACEMENT_3D('',#54798,#42112,#42113);
#35542=AXIS2_PLACEMENT_3D('',#54800,#42114,#42115);
#35543=AXIS2_PLACEMENT_3D('',#54803,#42117,#42118);
#35544=AXIS2_PLACEMENT_3D('',#54804,#42119,#42120);
#35545=AXIS2_PLACEMENT_3D('',#54810,#42124,#42125);
#35546=AXIS2_PLACEMENT_3D('',#54812,#42126,#42127);
#35547=AXIS2_PLACEMENT_3D('',#54815,#42129,#42130);
#35548=AXIS2_PLACEMENT_3D('',#54816,#42131,#42132);
#35549=AXIS2_PLACEMENT_3D('',#54822,#42136,#42137);
#35550=AXIS2_PLACEMENT_3D('',#54824,#42138,#42139);
#35551=AXIS2_PLACEMENT_3D('',#54826,#42140,#42141);
#35552=AXIS2_PLACEMENT_3D('',#54828,#42143,#42144);
#35553=AXIS2_PLACEMENT_3D('',#54834,#42148,#42149);
#35554=AXIS2_PLACEMENT_3D('',#54835,#42150,#42151);
#35555=AXIS2_PLACEMENT_3D('',#54836,#42152,#42153);
#35556=AXIS2_PLACEMENT_3D('',#54837,#42154,#42155);
#35557=AXIS2_PLACEMENT_3D('',#54843,#42159,#42160);
#35558=AXIS2_PLACEMENT_3D('',#54845,#42161,#42162);
#35559=AXIS2_PLACEMENT_3D('',#54848,#42164,#42165);
#35560=AXIS2_PLACEMENT_3D('',#54849,#42166,#42167);
#35561=AXIS2_PLACEMENT_3D('',#54855,#42171,#42172);
#35562=AXIS2_PLACEMENT_3D('',#54856,#42173,#42174);
#35563=AXIS2_PLACEMENT_3D('',#54857,#42175,#42176);
#35564=AXIS2_PLACEMENT_3D('',#54858,#42177,#42178);
#35565=AXIS2_PLACEMENT_3D('',#54859,#42179,#42180);
#35566=AXIS2_PLACEMENT_3D('',#54860,#42181,#42182);
#35567=AXIS2_PLACEMENT_3D('',#54863,#42183,#42184);
#35568=AXIS2_PLACEMENT_3D('',#54867,#42186,#42187);
#35569=AXIS2_PLACEMENT_3D('',#54869,#42189,#42190);
#35570=AXIS2_PLACEMENT_3D('',#54875,#42194,#42195);
#35571=AXIS2_PLACEMENT_3D('',#54877,#42196,#42197);
#35572=AXIS2_PLACEMENT_3D('',#54880,#42199,#42200);
#35573=AXIS2_PLACEMENT_3D('',#54881,#42201,#42202);
#35574=AXIS2_PLACEMENT_3D('',#54887,#42206,#42207);
#35575=AXIS2_PLACEMENT_3D('',#54889,#42208,#42209);
#35576=AXIS2_PLACEMENT_3D('',#54892,#42211,#42212);
#35577=AXIS2_PLACEMENT_3D('',#54893,#42213,#42214);
#35578=AXIS2_PLACEMENT_3D('',#54899,#42218,#42219);
#35579=AXIS2_PLACEMENT_3D('',#54901,#42220,#42221);
#35580=AXIS2_PLACEMENT_3D('',#54904,#42223,#42224);
#35581=AXIS2_PLACEMENT_3D('',#54905,#42225,#42226);
#35582=AXIS2_PLACEMENT_3D('',#54908,#42229,#42230);
#35583=AXIS2_PLACEMENT_3D('',#54911,#42231,#42232);
#35584=AXIS2_PLACEMENT_3D('',#54915,#42234,#42235);
#35585=AXIS2_PLACEMENT_3D('',#54917,#42237,#42238);
#35586=AXIS2_PLACEMENT_3D('',#54923,#42242,#42243);
#35587=AXIS2_PLACEMENT_3D('',#54925,#42244,#42245);
#35588=AXIS2_PLACEMENT_3D('',#54927,#42246,#42247);
#35589=AXIS2_PLACEMENT_3D('',#54929,#42249,#42250);
#35590=AXIS2_PLACEMENT_3D('',#54935,#42254,#42255);
#35591=AXIS2_PLACEMENT_3D('',#54937,#42256,#42257);
#35592=AXIS2_PLACEMENT_3D('',#54939,#42258,#42259);
#35593=AXIS2_PLACEMENT_3D('',#54941,#42261,#42262);
#35594=AXIS2_PLACEMENT_3D('',#54947,#42266,#42267);
#35595=AXIS2_PLACEMENT_3D('',#54949,#42268,#42269);
#35596=AXIS2_PLACEMENT_3D('',#54951,#42270,#42271);
#35597=AXIS2_PLACEMENT_3D('',#54953,#42273,#42274);
#35598=AXIS2_PLACEMENT_3D('',#54956,#42277,#42278);
#35599=AXIS2_PLACEMENT_3D('',#54957,#42279,#42280);
#35600=AXIS2_PLACEMENT_3D('',#54958,#42281,#42282);
#35601=AXIS2_PLACEMENT_3D('',#54961,#42283,#42284);
#35602=AXIS2_PLACEMENT_3D('',#54965,#42286,#42287);
#35603=AXIS2_PLACEMENT_3D('',#54967,#42289,#42290);
#35604=AXIS2_PLACEMENT_3D('',#54973,#42294,#42295);
#35605=AXIS2_PLACEMENT_3D('',#54975,#42296,#42297);
#35606=AXIS2_PLACEMENT_3D('',#54978,#42299,#42300);
#35607=AXIS2_PLACEMENT_3D('',#54979,#42301,#42302);
#35608=AXIS2_PLACEMENT_3D('',#54985,#42306,#42307);
#35609=AXIS2_PLACEMENT_3D('',#54987,#42308,#42309);
#35610=AXIS2_PLACEMENT_3D('',#54990,#42311,#42312);
#35611=AXIS2_PLACEMENT_3D('',#54991,#42313,#42314);
#35612=AXIS2_PLACEMENT_3D('',#54997,#42318,#42319);
#35613=AXIS2_PLACEMENT_3D('',#54999,#42320,#42321);
#35614=AXIS2_PLACEMENT_3D('',#55002,#42323,#42324);
#35615=AXIS2_PLACEMENT_3D('',#55003,#42325,#42326);
#35616=AXIS2_PLACEMENT_3D('',#55006,#42329,#42330);
#35617=AXIS2_PLACEMENT_3D('',#55009,#42331,#42332);
#35618=AXIS2_PLACEMENT_3D('',#55013,#42334,#42335);
#35619=AXIS2_PLACEMENT_3D('',#55015,#42337,#42338);
#35620=AXIS2_PLACEMENT_3D('',#55021,#42342,#42343);
#35621=AXIS2_PLACEMENT_3D('',#55023,#42344,#42345);
#35622=AXIS2_PLACEMENT_3D('',#55025,#42346,#42347);
#35623=AXIS2_PLACEMENT_3D('',#55027,#42349,#42350);
#35624=AXIS2_PLACEMENT_3D('',#55033,#42354,#42355);
#35625=AXIS2_PLACEMENT_3D('',#55035,#42356,#42357);
#35626=AXIS2_PLACEMENT_3D('',#55037,#42358,#42359);
#35627=AXIS2_PLACEMENT_3D('',#55039,#42361,#42362);
#35628=AXIS2_PLACEMENT_3D('',#55045,#42366,#42367);
#35629=AXIS2_PLACEMENT_3D('',#55047,#42368,#42369);
#35630=AXIS2_PLACEMENT_3D('',#55049,#42370,#42371);
#35631=AXIS2_PLACEMENT_3D('',#55051,#42373,#42374);
#35632=AXIS2_PLACEMENT_3D('',#55054,#42377,#42378);
#35633=AXIS2_PLACEMENT_3D('',#55055,#42379,#42380);
#35634=AXIS2_PLACEMENT_3D('',#55056,#42381,#42382);
#35635=AXIS2_PLACEMENT_3D('',#55059,#42383,#42384);
#35636=AXIS2_PLACEMENT_3D('',#55063,#42386,#42387);
#35637=AXIS2_PLACEMENT_3D('',#55065,#42389,#42390);
#35638=AXIS2_PLACEMENT_3D('',#55071,#42394,#42395);
#35639=AXIS2_PLACEMENT_3D('',#55073,#42396,#42397);
#35640=AXIS2_PLACEMENT_3D('',#55076,#42399,#42400);
#35641=AXIS2_PLACEMENT_3D('',#55077,#42401,#42402);
#35642=AXIS2_PLACEMENT_3D('',#55083,#42406,#42407);
#35643=AXIS2_PLACEMENT_3D('',#55085,#42408,#42409);
#35644=AXIS2_PLACEMENT_3D('',#55088,#42411,#42412);
#35645=AXIS2_PLACEMENT_3D('',#55089,#42413,#42414);
#35646=AXIS2_PLACEMENT_3D('',#55095,#42418,#42419);
#35647=AXIS2_PLACEMENT_3D('',#55097,#42420,#42421);
#35648=AXIS2_PLACEMENT_3D('',#55100,#42423,#42424);
#35649=AXIS2_PLACEMENT_3D('',#55101,#42425,#42426);
#35650=AXIS2_PLACEMENT_3D('',#55104,#42429,#42430);
#35651=AXIS2_PLACEMENT_3D('',#55107,#42431,#42432);
#35652=AXIS2_PLACEMENT_3D('',#55111,#42434,#42435);
#35653=AXIS2_PLACEMENT_3D('',#55113,#42437,#42438);
#35654=AXIS2_PLACEMENT_3D('',#55119,#42442,#42443);
#35655=AXIS2_PLACEMENT_3D('',#55121,#42444,#42445);
#35656=AXIS2_PLACEMENT_3D('',#55123,#42446,#42447);
#35657=AXIS2_PLACEMENT_3D('',#55125,#42449,#42450);
#35658=AXIS2_PLACEMENT_3D('',#55131,#42454,#42455);
#35659=AXIS2_PLACEMENT_3D('',#55133,#42456,#42457);
#35660=AXIS2_PLACEMENT_3D('',#55135,#42458,#42459);
#35661=AXIS2_PLACEMENT_3D('',#55137,#42461,#42462);
#35662=AXIS2_PLACEMENT_3D('',#55143,#42466,#42467);
#35663=AXIS2_PLACEMENT_3D('',#55145,#42468,#42469);
#35664=AXIS2_PLACEMENT_3D('',#55147,#42470,#42471);
#35665=AXIS2_PLACEMENT_3D('',#55149,#42473,#42474);
#35666=AXIS2_PLACEMENT_3D('',#55152,#42477,#42478);
#35667=AXIS2_PLACEMENT_3D('',#55153,#42479,#42480);
#35668=AXIS2_PLACEMENT_3D('',#55154,#42481,#42482);
#35669=AXIS2_PLACEMENT_3D('',#55157,#42483,#42484);
#35670=AXIS2_PLACEMENT_3D('',#55161,#42486,#42487);
#35671=AXIS2_PLACEMENT_3D('',#55163,#42489,#42490);
#35672=AXIS2_PLACEMENT_3D('',#55169,#42494,#42495);
#35673=AXIS2_PLACEMENT_3D('',#55171,#42496,#42497);
#35674=AXIS2_PLACEMENT_3D('',#55174,#42499,#42500);
#35675=AXIS2_PLACEMENT_3D('',#55175,#42501,#42502);
#35676=AXIS2_PLACEMENT_3D('',#55181,#42506,#42507);
#35677=AXIS2_PLACEMENT_3D('',#55183,#42508,#42509);
#35678=AXIS2_PLACEMENT_3D('',#55186,#42511,#42512);
#35679=AXIS2_PLACEMENT_3D('',#55187,#42513,#42514);
#35680=AXIS2_PLACEMENT_3D('',#55193,#42518,#42519);
#35681=AXIS2_PLACEMENT_3D('',#55195,#42520,#42521);
#35682=AXIS2_PLACEMENT_3D('',#55198,#42523,#42524);
#35683=AXIS2_PLACEMENT_3D('',#55199,#42525,#42526);
#35684=AXIS2_PLACEMENT_3D('',#55202,#42529,#42530);
#35685=AXIS2_PLACEMENT_3D('',#55205,#42531,#42532);
#35686=AXIS2_PLACEMENT_3D('',#55209,#42534,#42535);
#35687=AXIS2_PLACEMENT_3D('',#55211,#42537,#42538);
#35688=AXIS2_PLACEMENT_3D('',#55217,#42542,#42543);
#35689=AXIS2_PLACEMENT_3D('',#55219,#42544,#42545);
#35690=AXIS2_PLACEMENT_3D('',#55221,#42546,#42547);
#35691=AXIS2_PLACEMENT_3D('',#55223,#42549,#42550);
#35692=AXIS2_PLACEMENT_3D('',#55229,#42554,#42555);
#35693=AXIS2_PLACEMENT_3D('',#55231,#42556,#42557);
#35694=AXIS2_PLACEMENT_3D('',#55233,#42558,#42559);
#35695=AXIS2_PLACEMENT_3D('',#55235,#42561,#42562);
#35696=AXIS2_PLACEMENT_3D('',#55241,#42566,#42567);
#35697=AXIS2_PLACEMENT_3D('',#55243,#42568,#42569);
#35698=AXIS2_PLACEMENT_3D('',#55245,#42570,#42571);
#35699=AXIS2_PLACEMENT_3D('',#55247,#42573,#42574);
#35700=AXIS2_PLACEMENT_3D('',#55250,#42577,#42578);
#35701=AXIS2_PLACEMENT_3D('',#55251,#42579,#42580);
#41079=DIRECTION('axis',(0.,0.,1.));
#41080=DIRECTION('refdir',(1.,0.,0.));
#41081=DIRECTION('center_axis',(-1.53651348736138E-16,-1.,1.45117688885522E-12));
#41082=DIRECTION('ref_axis',(-3.34404360992238E-15,-1.45117688885522E-12,
-1.));
#41083=DIRECTION('',(1.,-1.53651348740991E-16,-3.34404360992216E-15));
#41084=DIRECTION('',(3.34404360992238E-15,1.45117688885522E-12,1.));
#41085=DIRECTION('',(1.,-1.53651348740991E-16,-3.34404360992216E-15));
#41086=DIRECTION('',(3.34404360992238E-15,1.45117688885522E-12,1.));
#41087=DIRECTION('center_axis',(3.34404360992238E-15,1.45117688885522E-12,
1.));
#41088=DIRECTION('ref_axis',(5.00596043931499E-16,1.,-1.45117688885522E-12));
#41089=DIRECTION('center_axis',(3.34404360992238E-15,1.45117688885522E-12,
1.));
#41090=DIRECTION('ref_axis',(5.00596043931499E-16,1.,-1.45117688885522E-12));
#41091=DIRECTION('',(3.34404360992238E-15,1.45117688885522E-12,1.));
#41092=DIRECTION('center_axis',(3.34404360992238E-15,1.45117688885522E-12,
1.));
#41093=DIRECTION('ref_axis',(5.00596043931499E-16,1.,-1.45117688885522E-12));
#41094=DIRECTION('center_axis',(1.,-3.61818165858207E-16,-3.34404360992185E-15));
#41095=DIRECTION('ref_axis',(-3.34404360992238E-15,-1.45117688885522E-12,
-1.));
#41096=DIRECTION('',(3.61818165853354E-16,1.,-1.45117688885522E-12));
#41097=DIRECTION('',(3.34404360992238E-15,1.45117688885522E-12,1.));
#41098=DIRECTION('',(3.61818165853354E-16,1.,-1.45117688885522E-12));
#41099=DIRECTION('center_axis',(3.34404360992238E-15,1.45117688885522E-12,
1.));
#41100=DIRECTION('ref_axis',(-1.,5.00596043936352E-16,3.34404360992165E-15));
#41101=DIRECTION('center_axis',(3.34404360992238E-15,1.45117688885522E-12,
1.));
#41102=DIRECTION('ref_axis',(-1.,5.00596043936352E-16,3.34404360992165E-15));
#41103=DIRECTION('',(3.34404360992238E-15,1.45117688885522E-12,1.));
#41104=DIRECTION('center_axis',(3.34404360992238E-15,1.45117688885522E-12,
1.));
#41105=DIRECTION('ref_axis',(-1.,5.00596043936352E-16,3.34404360992165E-15));
#41106=DIRECTION('center_axis',(1.,-6.39373922014497E-16,-3.34404360992145E-15));
#41107=DIRECTION('ref_axis',(-3.34404360992238E-15,-1.45117688885522E-12,
-1.));
#41108=DIRECTION('',(-6.39373922009644E-16,-1.,1.45117688885522E-12));
#41109=DIRECTION('',(3.34404360992238E-15,1.45117688885522E-12,1.));
#41110=DIRECTION('',(-6.39373922009644E-16,-1.,1.45117688885522E-12));
#41111=DIRECTION('',(3.34404360992238E-15,1.45117688885522E-12,1.));
#41112=DIRECTION('center_axis',(3.34404360992238E-15,1.45117688885522E-12,
1.));
#41113=DIRECTION('ref_axis',(-5.45154683810787E-17,1.,-1.45117688885522E-12));
#41114=DIRECTION('center_axis',(-3.34404360992238E-15,-1.45117688885522E-12,
-1.));
#41115=DIRECTION('ref_axis',(-5.45154683810787E-17,1.,-1.45117688885522E-12));
#41116=DIRECTION('',(3.34404360992238E-15,1.45117688885522E-12,1.));
#41117=DIRECTION('center_axis',(-3.34404360992238E-15,-1.45117688885522E-12,
-1.));
#41118=DIRECTION('ref_axis',(-5.45154683810787E-17,1.,-1.45117688885522E-12));
#41119=DIRECTION('center_axis',(-5.00596043931499E-16,-1.,1.45117688885522E-12));
#41120=DIRECTION('ref_axis',(-3.34404360992238E-15,-1.45117688885522E-12,
-1.));
#41121=DIRECTION('',(-1.,5.00596043936352E-16,3.34404360992165E-15));
#41122=DIRECTION('',(3.34404360992238E-15,1.45117688885522E-12,1.));
#41123=DIRECTION('',(-1.,5.00596043936352E-16,3.34404360992165E-15));
#41124=DIRECTION('center_axis',(3.34404360992238E-15,1.45117688885522E-12,
1.));
#41125=DIRECTION('ref_axis',(1.,-5.00596043936352E-16,-3.34404360992165E-15));
#41126=DIRECTION('center_axis',(-3.34404360992238E-15,-1.45117688885522E-12,
-1.));
#41127=DIRECTION('ref_axis',(1.,-5.00596043936352E-16,-3.34404360992165E-15));
#41128=DIRECTION('',(3.34404360992238E-15,1.45117688885522E-12,1.));
#41129=DIRECTION('center_axis',(-3.34404360992238E-15,-1.45117688885522E-12,
-1.));
#41130=DIRECTION('ref_axis',(1.,-5.00596043936352E-16,-3.34404360992165E-15));
#41131=DIRECTION('center_axis',(3.61818165853354E-16,1.,-1.45117688885522E-12));
#41132=DIRECTION('ref_axis',(3.34404360992238E-15,1.45117688885522E-12,
1.));
#41133=DIRECTION('',(-1.,3.61818165858207E-16,3.34404360992185E-15));
#41134=DIRECTION('',(3.34404360992238E-15,1.45117688885522E-12,1.));
#41135=DIRECTION('',(-1.,3.61818165858207E-16,3.34404360992185E-15));
#41136=DIRECTION('center_axis',(3.34404360992238E-15,1.45117688885522E-12,
1.));
#41137=DIRECTION('ref_axis',(1.,-5.00596043936352E-16,-3.34404360992165E-15));
#41138=DIRECTION('center_axis',(3.34404360992238E-15,1.45117688885522E-12,
1.));
#41139=DIRECTION('ref_axis',(1.,-5.00596043936352E-16,-3.34404360992165E-15));
#41140=DIRECTION('center_axis',(3.34404360992238E-15,1.45117688885522E-12,
1.));
#41141=DIRECTION('ref_axis',(1.,-5.00596043936352E-16,-3.34404360992165E-15));
#41142=DIRECTION('',(3.34404360992238E-15,1.45117688885522E-12,1.));
#41143=DIRECTION('center_axis',(-1.,3.61818165858207E-16,3.34404360992185E-15));
#41144=DIRECTION('ref_axis',(3.34404360992238E-15,1.45117688885522E-12,
1.));
#41145=DIRECTION('',(-3.61818165853354E-16,-1.,1.45117688885522E-12));
#41146=DIRECTION('',(-3.61818165853354E-16,-1.,1.45117688885522E-12));
#41147=DIRECTION('',(3.34404360992238E-15,1.45117688885522E-12,1.));
#41148=DIRECTION('center_axis',(3.34404360992238E-15,1.45117688885522E-12,
1.));
#41149=DIRECTION('ref_axis',(-5.00596043931499E-16,-1.,1.45117688885522E-12));
#41150=DIRECTION('center_axis',(3.34404360992238E-15,1.45117688885522E-12,
1.));
#41151=DIRECTION('ref_axis',(-5.00596043931499E-16,-1.,1.45117688885522E-12));
#41152=DIRECTION('center_axis',(3.34404360992238E-15,1.45117688885522E-12,
1.));
#41153=DIRECTION('ref_axis',(-5.00596043931499E-16,-1.,1.45117688885522E-12));
#41154=DIRECTION('center_axis',(-1.,5.00596043936352E-16,3.34404360992165E-15));
#41155=DIRECTION('ref_axis',(3.34404360992238E-15,1.45117688885522E-12,
1.));
#41156=DIRECTION('',(5.00596043931499E-16,1.,-1.45117688885522E-12));
#41157=DIRECTION('',(3.34404360992238E-15,1.45117688885522E-12,1.));
#41158=DIRECTION('',(5.00596043931499E-16,1.,-1.45117688885522E-12));
#41159=DIRECTION('center_axis',(3.34404360992238E-15,1.45117688885522E-12,
1.));
#41160=DIRECTION('ref_axis',(-5.00596043931499E-16,-1.,1.45117688885522E-12));
#41161=DIRECTION('center_axis',(-3.34404360992238E-15,-1.45117688885522E-12,
-1.));
#41162=DIRECTION('ref_axis',(-5.00596043931499E-16,-1.,1.45117688885522E-12));
#41163=DIRECTION('',(3.34404360992238E-15,1.45117688885522E-12,1.));
#41164=DIRECTION('center_axis',(-3.34404360992238E-15,-1.45117688885522E-12,
-1.));
#41165=DIRECTION('ref_axis',(-5.00596043931499E-16,-1.,1.45117688885522E-12));
#41166=DIRECTION('center_axis',(-5.45154683810787E-17,1.,-1.45117688885522E-12));
#41167=DIRECTION('ref_axis',(3.34404360992238E-15,1.45117688885522E-12,
1.));
#41168=DIRECTION('',(1.,5.45154683762259E-17,-3.34404360992246E-15));
#41169=DIRECTION('',(3.34404360992238E-15,1.45117688885522E-12,1.));
#41170=DIRECTION('',(1.,5.45154683762259E-17,-3.34404360992246E-15));
#41171=DIRECTION('center_axis',(3.34404360992238E-15,1.45117688885522E-12,
1.));
#41172=DIRECTION('ref_axis',(-1.,5.00596043936352E-16,3.34404360992165E-15));
#41173=DIRECTION('center_axis',(-3.34404360992238E-15,-1.45117688885522E-12,
-1.));
#41174=DIRECTION('ref_axis',(-1.,5.00596043936352E-16,3.34404360992165E-15));
#41175=DIRECTION('center_axis',(-3.34404360992238E-15,-1.45117688885522E-12,
-1.));
#41176=DIRECTION('ref_axis',(-1.,5.00596043936352E-16,3.34404360992165E-15));
#41177=DIRECTION('center_axis',(3.34404360992238E-15,1.45117688885522E-12,
1.));
#41178=DIRECTION('ref_axis',(1.,-5.00596043936352E-16,-3.34404360992165E-15));
#41179=DIRECTION('center_axis',(3.34404360992238E-15,1.45117688885522E-12,
1.));
#41180=DIRECTION('ref_axis',(1.,-5.00596043936352E-16,-3.34404360992165E-15));
#41181=DIRECTION('center_axis',(-1.53651348736138E-16,-1.,1.45117688885522E-12));
#41182=DIRECTION('ref_axis',(-3.34404360992238E-15,-1.45117688885522E-12,
-1.));
#41183=DIRECTION('',(1.,-1.53651348740991E-16,-3.34404360992216E-15));
#41184=DIRECTION('',(3.34404360992238E-15,1.45117688885522E-12,1.));
#41185=DIRECTION('',(1.,-1.53651348740991E-16,-3.34404360992216E-15));
#41186=DIRECTION('',(3.34404360992238E-15,1.45117688885522E-12,1.));
#41187=DIRECTION('center_axis',(3.34404360992238E-15,1.45117688885522E-12,
1.));
#41188=DIRECTION('ref_axis',(5.00596043931499E-16,1.,-1.45117688885522E-12));
#41189=DIRECTION('center_axis',(3.34404360992238E-15,1.45117688885522E-12,
1.));
#41190=DIRECTION('ref_axis',(5.00596043931499E-16,1.,-1.45117688885522E-12));
#41191=DIRECTION('',(3.34404360992238E-15,1.45117688885522E-12,1.));
#41192=DIRECTION('center_axis',(3.34404360992238E-15,1.45117688885522E-12,
1.));
#41193=DIRECTION('ref_axis',(5.00596043931499E-16,1.,-1.45117688885522E-12));
#41194=DIRECTION('center_axis',(1.,-3.61818165858207E-16,-3.34404360992185E-15));
#41195=DIRECTION('ref_axis',(-3.34404360992238E-15,-1.45117688885522E-12,
-1.));
#41196=DIRECTION('',(3.61818165853354E-16,1.,-1.45117688885522E-12));
#41197=DIRECTION('',(3.34404360992238E-15,1.45117688885522E-12,1.));
#41198=DIRECTION('',(3.61818165853354E-16,1.,-1.45117688885522E-12));
#41199=DIRECTION('center_axis',(3.34404360992238E-15,1.45117688885522E-12,
1.));
#41200=DIRECTION('ref_axis',(-1.,5.00596043936352E-16,3.34404360992165E-15));
#41201=DIRECTION('center_axis',(3.34404360992238E-15,1.45117688885522E-12,
1.));
#41202=DIRECTION('ref_axis',(-1.,5.00596043936352E-16,3.34404360992165E-15));
#41203=DIRECTION('',(3.34404360992238E-15,1.45117688885522E-12,1.));
#41204=DIRECTION('center_axis',(3.34404360992238E-15,1.45117688885522E-12,
1.));
#41205=DIRECTION('ref_axis',(-1.,5.00596043936352E-16,3.34404360992165E-15));
#41206=DIRECTION('center_axis',(1.,-6.39373922014497E-16,-3.34404360992145E-15));
#41207=DIRECTION('ref_axis',(-3.34404360992238E-15,-1.45117688885522E-12,
-1.));
#41208=DIRECTION('',(-6.39373922009644E-16,-1.,1.45117688885522E-12));
#41209=DIRECTION('',(3.34404360992238E-15,1.45117688885522E-12,1.));
#41210=DIRECTION('',(-6.39373922009644E-16,-1.,1.45117688885522E-12));
#41211=DIRECTION('',(3.34404360992238E-15,1.45117688885522E-12,1.));
#41212=DIRECTION('center_axis',(3.34404360992238E-15,1.45117688885522E-12,
1.));
#41213=DIRECTION('ref_axis',(-5.45154683810787E-17,1.,-1.45117688885522E-12));
#41214=DIRECTION('center_axis',(-3.34404360992238E-15,-1.45117688885522E-12,
-1.));
#41215=DIRECTION('ref_axis',(-5.45154683810787E-17,1.,-1.45117688885522E-12));
#41216=DIRECTION('',(3.34404360992238E-15,1.45117688885522E-12,1.));
#41217=DIRECTION('center_axis',(-3.34404360992238E-15,-1.45117688885522E-12,
-1.));
#41218=DIRECTION('ref_axis',(-5.45154683810787E-17,1.,-1.45117688885522E-12));
#41219=DIRECTION('center_axis',(-5.00596043931499E-16,-1.,1.45117688885522E-12));
#41220=DIRECTION('ref_axis',(-3.34404360992238E-15,-1.45117688885522E-12,
-1.));
#41221=DIRECTION('',(-1.,5.00596043936352E-16,3.34404360992165E-15));
#41222=DIRECTION('',(3.34404360992238E-15,1.45117688885522E-12,1.));
#41223=DIRECTION('',(-1.,5.00596043936352E-16,3.34404360992165E-15));
#41224=DIRECTION('center_axis',(3.34404360992238E-15,1.45117688885522E-12,
1.));
#41225=DIRECTION('ref_axis',(1.,-5.00596043936352E-16,-3.34404360992165E-15));
#41226=DIRECTION('center_axis',(-3.34404360992238E-15,-1.45117688885522E-12,
-1.));
#41227=DIRECTION('ref_axis',(1.,-5.00596043936352E-16,-3.34404360992165E-15));
#41228=DIRECTION('',(3.34404360992238E-15,1.45117688885522E-12,1.));
#41229=DIRECTION('center_axis',(-3.34404360992238E-15,-1.45117688885522E-12,
-1.));
#41230=DIRECTION('ref_axis',(1.,-5.00596043936352E-16,-3.34404360992165E-15));
#41231=DIRECTION('center_axis',(3.61818165853354E-16,1.,-1.45117688885522E-12));
#41232=DIRECTION('ref_axis',(3.34404360992238E-15,1.45117688885522E-12,
1.));
#41233=DIRECTION('',(-1.,3.61818165858207E-16,3.34404360992185E-15));
#41234=DIRECTION('',(3.34404360992238E-15,1.45117688885522E-12,1.));
#41235=DIRECTION('',(-1.,3.61818165858207E-16,3.34404360992185E-15));
#41236=DIRECTION('center_axis',(3.34404360992238E-15,1.45117688885522E-12,
1.));
#41237=DIRECTION('ref_axis',(1.,-5.00596043936352E-16,-3.34404360992165E-15));
#41238=DIRECTION('center_axis',(3.34404360992238E-15,1.45117688885522E-12,
1.));
#41239=DIRECTION('ref_axis',(1.,-5.00596043936352E-16,-3.34404360992165E-15));
#41240=DIRECTION('center_axis',(3.34404360992238E-15,1.45117688885522E-12,
1.));
#41241=DIRECTION('ref_axis',(1.,-5.00596043936352E-16,-3.34404360992165E-15));
#41242=DIRECTION('',(3.34404360992238E-15,1.45117688885522E-12,1.));
#41243=DIRECTION('center_axis',(-1.,3.61818165858207E-16,3.34404360992185E-15));
#41244=DIRECTION('ref_axis',(3.34404360992238E-15,1.45117688885522E-12,
1.));
#41245=DIRECTION('',(-3.61818165853354E-16,-1.,1.45117688885522E-12));
#41246=DIRECTION('',(-3.61818165853354E-16,-1.,1.45117688885522E-12));
#41247=DIRECTION('',(3.34404360992238E-15,1.45117688885522E-12,1.));
#41248=DIRECTION('center_axis',(3.34404360992238E-15,1.45117688885522E-12,
1.));
#41249=DIRECTION('ref_axis',(-5.00596043931499E-16,-1.,1.45117688885522E-12));
#41250=DIRECTION('center_axis',(3.34404360992238E-15,1.45117688885522E-12,
1.));
#41251=DIRECTION('ref_axis',(-5.00596043931499E-16,-1.,1.45117688885522E-12));
#41252=DIRECTION('center_axis',(3.34404360992238E-15,1.45117688885522E-12,
1.));
#41253=DIRECTION('ref_axis',(-5.00596043931499E-16,-1.,1.45117688885522E-12));
#41254=DIRECTION('center_axis',(-1.,5.00596043936352E-16,3.34404360992165E-15));
#41255=DIRECTION('ref_axis',(3.34404360992238E-15,1.45117688885522E-12,
1.));
#41256=DIRECTION('',(5.00596043931499E-16,1.,-1.45117688885522E-12));
#41257=DIRECTION('',(3.34404360992238E-15,1.45117688885522E-12,1.));
#41258=DIRECTION('',(5.00596043931499E-16,1.,-1.45117688885522E-12));
#41259=DIRECTION('center_axis',(3.34404360992238E-15,1.45117688885522E-12,
1.));
#41260=DIRECTION('ref_axis',(-5.00596043931499E-16,-1.,1.45117688885522E-12));
#41261=DIRECTION('center_axis',(-3.34404360992238E-15,-1.45117688885522E-12,
-1.));
#41262=DIRECTION('ref_axis',(-5.00596043931499E-16,-1.,1.45117688885522E-12));
#41263=DIRECTION('',(3.34404360992238E-15,1.45117688885522E-12,1.));
#41264=DIRECTION('center_axis',(-3.34404360992238E-15,-1.45117688885522E-12,
-1.));
#41265=DIRECTION('ref_axis',(-5.00596043931499E-16,-1.,1.45117688885522E-12));
#41266=DIRECTION('center_axis',(-5.45154683810787E-17,1.,-1.45117688885522E-12));
#41267=DIRECTION('ref_axis',(3.34404360992238E-15,1.45117688885522E-12,
1.));
#41268=DIRECTION('',(1.,5.45154683762259E-17,-3.34404360992246E-15));
#41269=DIRECTION('',(3.34404360992238E-15,1.45117688885522E-12,1.));
#41270=DIRECTION('',(1.,5.45154683762259E-17,-3.34404360992246E-15));
#41271=DIRECTION('center_axis',(3.34404360992238E-15,1.45117688885522E-12,
1.));
#41272=DIRECTION('ref_axis',(-1.,5.00596043936352E-16,3.34404360992165E-15));
#41273=DIRECTION('center_axis',(-3.34404360992238E-15,-1.45117688885522E-12,
-1.));
#41274=DIRECTION('ref_axis',(-1.,5.00596043936352E-16,3.34404360992165E-15));
#41275=DIRECTION('center_axis',(-3.34404360992238E-15,-1.45117688885522E-12,
-1.));
#41276=DIRECTION('ref_axis',(-1.,5.00596043936352E-16,3.34404360992165E-15));
#41277=DIRECTION('center_axis',(3.34404360992238E-15,1.45117688885522E-12,
1.));
#41278=DIRECTION('ref_axis',(1.,-5.00596043936352E-16,-3.34404360992165E-15));
#41279=DIRECTION('center_axis',(3.34404360992238E-15,1.45117688885522E-12,
1.));
#41280=DIRECTION('ref_axis',(1.,-5.00596043936352E-16,-3.34404360992165E-15));
#41281=DIRECTION('center_axis',(-1.53651348736138E-16,-1.,1.45117688885522E-12));
#41282=DIRECTION('ref_axis',(-3.34404360992238E-15,-1.45117688885522E-12,
-1.));
#41283=DIRECTION('',(1.,-1.53651348740991E-16,-3.34404360992216E-15));
#41284=DIRECTION('',(3.34404360992238E-15,1.45117688885522E-12,1.));
#41285=DIRECTION('',(1.,-1.53651348740991E-16,-3.34404360992216E-15));
#41286=DIRECTION('',(3.34404360992238E-15,1.45117688885522E-12,1.));
#41287=DIRECTION('center_axis',(3.34404360992238E-15,1.45117688885522E-12,
1.));
#41288=DIRECTION('ref_axis',(5.00596043931499E-16,1.,-1.45117688885522E-12));
#41289=DIRECTION('center_axis',(3.34404360992238E-15,1.45117688885522E-12,
1.));
#41290=DIRECTION('ref_axis',(5.00596043931499E-16,1.,-1.45117688885522E-12));
#41291=DIRECTION('',(3.34404360992238E-15,1.45117688885522E-12,1.));
#41292=DIRECTION('center_axis',(3.34404360992238E-15,1.45117688885522E-12,
1.));
#41293=DIRECTION('ref_axis',(5.00596043931499E-16,1.,-1.45117688885522E-12));
#41294=DIRECTION('center_axis',(1.,-3.61818165858207E-16,-3.34404360992185E-15));
#41295=DIRECTION('ref_axis',(-3.34404360992238E-15,-1.45117688885522E-12,
-1.));
#41296=DIRECTION('',(3.61818165853354E-16,1.,-1.45117688885522E-12));
#41297=DIRECTION('',(3.34404360992238E-15,1.45117688885522E-12,1.));
#41298=DIRECTION('',(3.61818165853354E-16,1.,-1.45117688885522E-12));
#41299=DIRECTION('center_axis',(3.34404360992238E-15,1.45117688885522E-12,
1.));
#41300=DIRECTION('ref_axis',(-1.,5.00596043936352E-16,3.34404360992165E-15));
#41301=DIRECTION('center_axis',(3.34404360992238E-15,1.45117688885522E-12,
1.));
#41302=DIRECTION('ref_axis',(-1.,5.00596043936352E-16,3.34404360992165E-15));
#41303=DIRECTION('',(3.34404360992238E-15,1.45117688885522E-12,1.));
#41304=DIRECTION('center_axis',(3.34404360992238E-15,1.45117688885522E-12,
1.));
#41305=DIRECTION('ref_axis',(-1.,5.00596043936352E-16,3.34404360992165E-15));
#41306=DIRECTION('center_axis',(1.,-6.39373922014497E-16,-3.34404360992145E-15));
#41307=DIRECTION('ref_axis',(-3.34404360992238E-15,-1.45117688885522E-12,
-1.));
#41308=DIRECTION('',(-6.39373922009644E-16,-1.,1.45117688885522E-12));
#41309=DIRECTION('',(3.34404360992238E-15,1.45117688885522E-12,1.));
#41310=DIRECTION('',(-6.39373922009644E-16,-1.,1.45117688885522E-12));
#41311=DIRECTION('',(3.34404360992238E-15,1.45117688885522E-12,1.));
#41312=DIRECTION('center_axis',(3.34404360992238E-15,1.45117688885522E-12,
1.));
#41313=DIRECTION('ref_axis',(-5.45154683810787E-17,1.,-1.45117688885522E-12));
#41314=DIRECTION('center_axis',(-3.34404360992238E-15,-1.45117688885522E-12,
-1.));
#41315=DIRECTION('ref_axis',(-5.45154683810787E-17,1.,-1.45117688885522E-12));
#41316=DIRECTION('',(3.34404360992238E-15,1.45117688885522E-12,1.));
#41317=DIRECTION('center_axis',(-3.34404360992238E-15,-1.45117688885522E-12,
-1.));
#41318=DIRECTION('ref_axis',(-5.45154683810787E-17,1.,-1.45117688885522E-12));
#41319=DIRECTION('center_axis',(-5.00596043931499E-16,-1.,1.45117688885522E-12));
#41320=DIRECTION('ref_axis',(-3.34404360992238E-15,-1.45117688885522E-12,
-1.));
#41321=DIRECTION('',(-1.,5.00596043936352E-16,3.34404360992165E-15));
#41322=DIRECTION('',(3.34404360992238E-15,1.45117688885522E-12,1.));
#41323=DIRECTION('',(-1.,5.00596043936352E-16,3.34404360992165E-15));
#41324=DIRECTION('center_axis',(3.34404360992238E-15,1.45117688885522E-12,
1.));
#41325=DIRECTION('ref_axis',(1.,-5.00596043936352E-16,-3.34404360992165E-15));
#41326=DIRECTION('center_axis',(-3.34404360992238E-15,-1.45117688885522E-12,
-1.));
#41327=DIRECTION('ref_axis',(1.,-5.00596043936352E-16,-3.34404360992165E-15));
#41328=DIRECTION('',(3.34404360992238E-15,1.45117688885522E-12,1.));
#41329=DIRECTION('center_axis',(-3.34404360992238E-15,-1.45117688885522E-12,
-1.));
#41330=DIRECTION('ref_axis',(1.,-5.00596043936352E-16,-3.34404360992165E-15));
#41331=DIRECTION('center_axis',(3.61818165853354E-16,1.,-1.45117688885522E-12));
#41332=DIRECTION('ref_axis',(3.34404360992238E-15,1.45117688885522E-12,
1.));
#41333=DIRECTION('',(-1.,3.61818165858207E-16,3.34404360992185E-15));
#41334=DIRECTION('',(3.34404360992238E-15,1.45117688885522E-12,1.));
#41335=DIRECTION('',(-1.,3.61818165858207E-16,3.34404360992185E-15));
#41336=DIRECTION('center_axis',(3.34404360992238E-15,1.45117688885522E-12,
1.));
#41337=DIRECTION('ref_axis',(1.,-5.00596043936352E-16,-3.34404360992165E-15));
#41338=DIRECTION('center_axis',(3.34404360992238E-15,1.45117688885522E-12,
1.));
#41339=DIRECTION('ref_axis',(1.,-5.00596043936352E-16,-3.34404360992165E-15));
#41340=DIRECTION('center_axis',(3.34404360992238E-15,1.45117688885522E-12,
1.));
#41341=DIRECTION('ref_axis',(1.,-5.00596043936352E-16,-3.34404360992165E-15));
#41342=DIRECTION('',(3.34404360992238E-15,1.45117688885522E-12,1.));
#41343=DIRECTION('center_axis',(-1.,3.61818165858207E-16,3.34404360992185E-15));
#41344=DIRECTION('ref_axis',(3.34404360992238E-15,1.45117688885522E-12,
1.));
#41345=DIRECTION('',(-3.61818165853354E-16,-1.,1.45117688885522E-12));
#41346=DIRECTION('',(-3.61818165853354E-16,-1.,1.45117688885522E-12));
#41347=DIRECTION('',(3.34404360992238E-15,1.45117688885522E-12,1.));
#41348=DIRECTION('center_axis',(3.34404360992238E-15,1.45117688885522E-12,
1.));
#41349=DIRECTION('ref_axis',(-5.00596043931499E-16,-1.,1.45117688885522E-12));
#41350=DIRECTION('center_axis',(3.34404360992238E-15,1.45117688885522E-12,
1.));
#41351=DIRECTION('ref_axis',(-5.00596043931499E-16,-1.,1.45117688885522E-12));
#41352=DIRECTION('center_axis',(3.34404360992238E-15,1.45117688885522E-12,
1.));
#41353=DIRECTION('ref_axis',(-5.00596043931499E-16,-1.,1.45117688885522E-12));
#41354=DIRECTION('center_axis',(-1.,5.00596043936352E-16,3.34404360992165E-15));
#41355=DIRECTION('ref_axis',(3.34404360992238E-15,1.45117688885522E-12,
1.));
#41356=DIRECTION('',(5.00596043931499E-16,1.,-1.45117688885522E-12));
#41357=DIRECTION('',(3.34404360992238E-15,1.45117688885522E-12,1.));
#41358=DIRECTION('',(5.00596043931499E-16,1.,-1.45117688885522E-12));
#41359=DIRECTION('center_axis',(3.34404360992238E-15,1.45117688885522E-12,
1.));
#41360=DIRECTION('ref_axis',(-5.00596043931499E-16,-1.,1.45117688885522E-12));
#41361=DIRECTION('center_axis',(-3.34404360992238E-15,-1.45117688885522E-12,
-1.));
#41362=DIRECTION('ref_axis',(-5.00596043931499E-16,-1.,1.45117688885522E-12));
#41363=DIRECTION('',(3.34404360992238E-15,1.45117688885522E-12,1.));
#41364=DIRECTION('center_axis',(-3.34404360992238E-15,-1.45117688885522E-12,
-1.));
#41365=DIRECTION('ref_axis',(-5.00596043931499E-16,-1.,1.45117688885522E-12));
#41366=DIRECTION('center_axis',(-5.45154683810787E-17,1.,-1.45117688885522E-12));
#41367=DIRECTION('ref_axis',(3.34404360992238E-15,1.45117688885522E-12,
1.));
#41368=DIRECTION('',(1.,5.45154683762259E-17,-3.34404360992246E-15));
#41369=DIRECTION('',(3.34404360992238E-15,1.45117688885522E-12,1.));
#41370=DIRECTION('',(1.,5.45154683762259E-17,-3.34404360992246E-15));
#41371=DIRECTION('center_axis',(3.34404360992238E-15,1.45117688885522E-12,
1.));
#41372=DIRECTION('ref_axis',(-1.,5.00596043936352E-16,3.34404360992165E-15));
#41373=DIRECTION('center_axis',(-3.34404360992238E-15,-1.45117688885522E-12,
-1.));
#41374=DIRECTION('ref_axis',(-1.,5.00596043936352E-16,3.34404360992165E-15));
#41375=DIRECTION('center_axis',(-3.34404360992238E-15,-1.45117688885522E-12,
-1.));
#41376=DIRECTION('ref_axis',(-1.,5.00596043936352E-16,3.34404360992165E-15));
#41377=DIRECTION('center_axis',(3.34404360992238E-15,1.45117688885522E-12,
1.));
#41378=DIRECTION('ref_axis',(1.,-5.00596043936352E-16,-3.34404360992165E-15));
#41379=DIRECTION('center_axis',(3.34404360992238E-15,1.45117688885522E-12,
1.));
#41380=DIRECTION('ref_axis',(1.,-5.00596043936352E-16,-3.34404360992165E-15));
#41381=DIRECTION('center_axis',(-1.53651348736138E-16,-1.,1.45117688885522E-12));
#41382=DIRECTION('ref_axis',(-3.34404360992238E-15,-1.45117688885522E-12,
-1.));
#41383=DIRECTION('',(1.,-1.53651348740991E-16,-3.34404360992216E-15));
#41384=DIRECTION('',(3.34404360992238E-15,1.45117688885522E-12,1.));
#41385=DIRECTION('',(1.,-1.53651348740991E-16,-3.34404360992216E-15));
#41386=DIRECTION('',(3.34404360992238E-15,1.45117688885522E-12,1.));
#41387=DIRECTION('center_axis',(3.34404360992238E-15,1.45117688885522E-12,
1.));
#41388=DIRECTION('ref_axis',(5.00596043931499E-16,1.,-1.45117688885522E-12));
#41389=DIRECTION('center_axis',(3.34404360992238E-15,1.45117688885522E-12,
1.));
#41390=DIRECTION('ref_axis',(5.00596043931499E-16,1.,-1.45117688885522E-12));
#41391=DIRECTION('',(3.34404360992238E-15,1.45117688885522E-12,1.));
#41392=DIRECTION('center_axis',(3.34404360992238E-15,1.45117688885522E-12,
1.));
#41393=DIRECTION('ref_axis',(5.00596043931499E-16,1.,-1.45117688885522E-12));
#41394=DIRECTION('center_axis',(1.,-3.61818165858207E-16,-3.34404360992185E-15));
#41395=DIRECTION('ref_axis',(-3.34404360992238E-15,-1.45117688885522E-12,
-1.));
#41396=DIRECTION('',(3.61818165853354E-16,1.,-1.45117688885522E-12));
#41397=DIRECTION('',(3.34404360992238E-15,1.45117688885522E-12,1.));
#41398=DIRECTION('',(3.61818165853354E-16,1.,-1.45117688885522E-12));
#41399=DIRECTION('center_axis',(3.34404360992238E-15,1.45117688885522E-12,
1.));
#41400=DIRECTION('ref_axis',(-1.,5.00596043936352E-16,3.34404360992165E-15));
#41401=DIRECTION('center_axis',(3.34404360992238E-15,1.45117688885522E-12,
1.));
#41402=DIRECTION('ref_axis',(-1.,5.00596043936352E-16,3.34404360992165E-15));
#41403=DIRECTION('',(3.34404360992238E-15,1.45117688885522E-12,1.));
#41404=DIRECTION('center_axis',(3.34404360992238E-15,1.45117688885522E-12,
1.));
#41405=DIRECTION('ref_axis',(-1.,5.00596043936352E-16,3.34404360992165E-15));
#41406=DIRECTION('center_axis',(1.,-6.39373922014497E-16,-3.34404360992145E-15));
#41407=DIRECTION('ref_axis',(-3.34404360992238E-15,-1.45117688885522E-12,
-1.));
#41408=DIRECTION('',(-6.39373922009644E-16,-1.,1.45117688885522E-12));
#41409=DIRECTION('',(3.34404360992238E-15,1.45117688885522E-12,1.));
#41410=DIRECTION('',(-6.39373922009644E-16,-1.,1.45117688885522E-12));
#41411=DIRECTION('',(3.34404360992238E-15,1.45117688885522E-12,1.));
#41412=DIRECTION('center_axis',(3.34404360992238E-15,1.45117688885522E-12,
1.));
#41413=DIRECTION('ref_axis',(-5.45154683810787E-17,1.,-1.45117688885522E-12));
#41414=DIRECTION('center_axis',(-3.34404360992238E-15,-1.45117688885522E-12,
-1.));
#41415=DIRECTION('ref_axis',(-5.45154683810787E-17,1.,-1.45117688885522E-12));
#41416=DIRECTION('',(3.34404360992238E-15,1.45117688885522E-12,1.));
#41417=DIRECTION('center_axis',(-3.34404360992238E-15,-1.45117688885522E-12,
-1.));
#41418=DIRECTION('ref_axis',(-5.45154683810787E-17,1.,-1.45117688885522E-12));
#41419=DIRECTION('center_axis',(-5.00596043931499E-16,-1.,1.45117688885522E-12));
#41420=DIRECTION('ref_axis',(-3.34404360992238E-15,-1.45117688885522E-12,
-1.));
#41421=DIRECTION('',(-1.,5.00596043936352E-16,3.34404360992165E-15));
#41422=DIRECTION('',(3.34404360992238E-15,1.45117688885522E-12,1.));
#41423=DIRECTION('',(-1.,5.00596043936352E-16,3.34404360992165E-15));
#41424=DIRECTION('center_axis',(3.34404360992238E-15,1.45117688885522E-12,
1.));
#41425=DIRECTION('ref_axis',(1.,-5.00596043936352E-16,-3.34404360992165E-15));
#41426=DIRECTION('center_axis',(-3.34404360992238E-15,-1.45117688885522E-12,
-1.));
#41427=DIRECTION('ref_axis',(1.,-5.00596043936352E-16,-3.34404360992165E-15));
#41428=DIRECTION('',(3.34404360992238E-15,1.45117688885522E-12,1.));
#41429=DIRECTION('center_axis',(-3.34404360992238E-15,-1.45117688885522E-12,
-1.));
#41430=DIRECTION('ref_axis',(1.,-5.00596043936352E-16,-3.34404360992165E-15));
#41431=DIRECTION('center_axis',(3.61818165853354E-16,1.,-1.45117688885522E-12));
#41432=DIRECTION('ref_axis',(3.34404360992238E-15,1.45117688885522E-12,
1.));
#41433=DIRECTION('',(-1.,3.61818165858207E-16,3.34404360992185E-15));
#41434=DIRECTION('',(3.34404360992238E-15,1.45117688885522E-12,1.));
#41435=DIRECTION('',(-1.,3.61818165858207E-16,3.34404360992185E-15));
#41436=DIRECTION('center_axis',(3.34404360992238E-15,1.45117688885522E-12,
1.));
#41437=DIRECTION('ref_axis',(1.,-5.00596043936352E-16,-3.34404360992165E-15));
#41438=DIRECTION('center_axis',(3.34404360992238E-15,1.45117688885522E-12,
1.));
#41439=DIRECTION('ref_axis',(1.,-5.00596043936352E-16,-3.34404360992165E-15));
#41440=DIRECTION('center_axis',(3.34404360992238E-15,1.45117688885522E-12,
1.));
#41441=DIRECTION('ref_axis',(1.,-5.00596043936352E-16,-3.34404360992165E-15));
#41442=DIRECTION('',(3.34404360992238E-15,1.45117688885522E-12,1.));
#41443=DIRECTION('center_axis',(-1.,3.61818165858207E-16,3.34404360992185E-15));
#41444=DIRECTION('ref_axis',(3.34404360992238E-15,1.45117688885522E-12,
1.));
#41445=DIRECTION('',(-3.61818165853354E-16,-1.,1.45117688885522E-12));
#41446=DIRECTION('',(-3.61818165853354E-16,-1.,1.45117688885522E-12));
#41447=DIRECTION('',(3.34404360992238E-15,1.45117688885522E-12,1.));
#41448=DIRECTION('center_axis',(3.34404360992238E-15,1.45117688885522E-12,
1.));
#41449=DIRECTION('ref_axis',(-5.00596043931499E-16,-1.,1.45117688885522E-12));
#41450=DIRECTION('center_axis',(3.34404360992238E-15,1.45117688885522E-12,
1.));
#41451=DIRECTION('ref_axis',(-5.00596043931499E-16,-1.,1.45117688885522E-12));
#41452=DIRECTION('center_axis',(3.34404360992238E-15,1.45117688885522E-12,
1.));
#41453=DIRECTION('ref_axis',(-5.00596043931499E-16,-1.,1.45117688885522E-12));
#41454=DIRECTION('center_axis',(-1.,5.00596043936352E-16,3.34404360992165E-15));
#41455=DIRECTION('ref_axis',(3.34404360992238E-15,1.45117688885522E-12,
1.));
#41456=DIRECTION('',(5.00596043931499E-16,1.,-1.45117688885522E-12));
#41457=DIRECTION('',(3.34404360992238E-15,1.45117688885522E-12,1.));
#41458=DIRECTION('',(5.00596043931499E-16,1.,-1.45117688885522E-12));
#41459=DIRECTION('center_axis',(3.34404360992238E-15,1.45117688885522E-12,
1.));
#41460=DIRECTION('ref_axis',(-5.00596043931499E-16,-1.,1.45117688885522E-12));
#41461=DIRECTION('center_axis',(-3.34404360992238E-15,-1.45117688885522E-12,
-1.));
#41462=DIRECTION('ref_axis',(-5.00596043931499E-16,-1.,1.45117688885522E-12));
#41463=DIRECTION('',(3.34404360992238E-15,1.45117688885522E-12,1.));
#41464=DIRECTION('center_axis',(-3.34404360992238E-15,-1.45117688885522E-12,
-1.));
#41465=DIRECTION('ref_axis',(-5.00596043931499E-16,-1.,1.45117688885522E-12));
#41466=DIRECTION('center_axis',(-5.45154683810787E-17,1.,-1.45117688885522E-12));
#41467=DIRECTION('ref_axis',(3.34404360992238E-15,1.45117688885522E-12,
1.));
#41468=DIRECTION('',(1.,5.45154683762259E-17,-3.34404360992246E-15));
#41469=DIRECTION('',(3.34404360992238E-15,1.45117688885522E-12,1.));
#41470=DIRECTION('',(1.,5.45154683762259E-17,-3.34404360992246E-15));
#41471=DIRECTION('center_axis',(3.34404360992238E-15,1.45117688885522E-12,
1.));
#41472=DIRECTION('ref_axis',(-1.,5.00596043936352E-16,3.34404360992165E-15));
#41473=DIRECTION('center_axis',(-3.34404360992238E-15,-1.45117688885522E-12,
-1.));
#41474=DIRECTION('ref_axis',(-1.,5.00596043936352E-16,3.34404360992165E-15));
#41475=DIRECTION('center_axis',(-3.34404360992238E-15,-1.45117688885522E-12,
-1.));
#41476=DIRECTION('ref_axis',(-1.,5.00596043936352E-16,3.34404360992165E-15));
#41477=DIRECTION('center_axis',(3.34404360992238E-15,1.45117688885522E-12,
1.));
#41478=DIRECTION('ref_axis',(1.,-5.00596043936352E-16,-3.34404360992165E-15));
#41479=DIRECTION('center_axis',(3.34404360992238E-15,1.45117688885522E-12,
1.));
#41480=DIRECTION('ref_axis',(1.,-5.00596043936352E-16,-3.34404360992165E-15));
#41481=DIRECTION('center_axis',(-0.707106781186547,0.707106781186548,-1.02377242289756E-12));
#41482=DIRECTION('ref_axis',(-0.707106781186548,-0.707106781186547,1.02850161472388E-12));
#41483=DIRECTION('center_axis',(-0.707106781186547,0.707106781186548,-1.02377242289756E-12));
#41484=DIRECTION('ref_axis',(-0.707106781186548,-0.707106781186547,1.02850161472388E-12));
#41485=DIRECTION('',(0.707106781186548,0.707106781186547,-1.02889413783855E-12));
#41486=DIRECTION('center_axis',(-0.707106781186547,0.707106781186548,-1.02377242289756E-12));
#41487=DIRECTION('ref_axis',(0.707106781186548,0.707106781186547,-1.02850161472388E-12));
#41488=DIRECTION('',(-3.20526573184424E-15,-1.45117688885522E-12,-1.));
#41489=DIRECTION('center_axis',(-0.707106781186547,0.707106781186548,-1.02377242289756E-12));
#41490=DIRECTION('ref_axis',(0.707106781186548,0.707106781186547,-1.02889413783855E-12));
#41491=DIRECTION('',(-0.707106781186548,-0.707106781186547,1.02850161472388E-12));
#41492=DIRECTION('center_axis',(-0.707106781186547,0.707106781186548,-1.02377242289756E-12));
#41493=DIRECTION('ref_axis',(-0.707106781186548,-0.707106781186547,1.02850161472388E-12));
#41494=DIRECTION('',(-3.34404360992239E-15,-1.45117688885522E-12,-1.));
#41495=DIRECTION('',(-0.707106781186548,-0.707106781186547,1.02859974550255E-12));
#41496=DIRECTION('center_axis',(0.707106781186547,-0.707106781186548,1.02377242289756E-12));
#41497=DIRECTION('ref_axis',(-0.707106781186548,-0.707106781186547,1.02850161472388E-12));
#41498=DIRECTION('',(3.48282148800053E-15,1.4513156667333E-12,1.));
#41499=DIRECTION('center_axis',(0.707106781186547,-0.707106781186548,1.02377242289756E-12));
#41500=DIRECTION('ref_axis',(-0.707106781186548,-0.707106781186547,1.02850161472388E-12));
#41501=DIRECTION('',(0.707106781186548,0.707106781186547,-1.02874694167055E-12));
#41502=DIRECTION('center_axis',(0.707106781186547,-0.707106781186548,1.02377242289756E-12));
#41503=DIRECTION('ref_axis',(0.707106781186548,0.707106781186547,-1.02850161472388E-12));
#41504=DIRECTION('',(-3.48282148800053E-15,-1.4513156667333E-12,-1.));
#41505=DIRECTION('center_axis',(0.707106781186547,-0.707106781186548,1.02377242289756E-12));
#41506=DIRECTION('ref_axis',(0.707106781186548,0.707106781186547,-1.02850161472388E-12));
#41507=DIRECTION('center_axis',(-3.69098830511775E-15,-1.45117688885522E-12,
-1.));
#41508=DIRECTION('ref_axis',(-5.00596043931499E-16,-1.,1.45117688885522E-12));
#41509=DIRECTION('',(5.00596043931499E-16,1.,-1.45117688885522E-12));
#41510=DIRECTION('',(-0.707106781186304,0.707106781186791,-1.02352709595125E-12));
#41511=DIRECTION('',(5.00596043931499E-16,1.,-1.45117688885522E-12));
#41512=DIRECTION('center_axis',(5.00596043931499E-16,1.,-1.45117688885522E-12));
#41513=DIRECTION('ref_axis',(-1.,5.00596043936352E-16,3.34404360992166E-15));
#41514=DIRECTION('',(5.00596043931499E-16,1.,-1.45117688885522E-12));
#41515=DIRECTION('center_axis',(0.707106781186791,0.707106781186304,-1.02850161472353E-12));
#41516=DIRECTION('ref_axis',(-0.707106781186304,0.707106781186791,-1.02377242289792E-12));
#41517=DIRECTION('center_axis',(1.,-5.00596043936553E-16,-3.48282148799981E-15));
#41518=DIRECTION('ref_axis',(5.00596043931499E-16,1.,-1.45117688885522E-12));
#41519=DIRECTION('',(5.00596043931499E-16,1.,-1.45117688885522E-12));
#41520=DIRECTION('',(-3.48282148800053E-15,-1.45103811097714E-12,-1.));
#41521=DIRECTION('center_axis',(5.00596043931499E-16,1.,-1.45117688885522E-12));
#41522=DIRECTION('ref_axis',(-3.34404360992239E-15,-1.45117688885522E-12,
-1.));
#41523=DIRECTION('',(5.00596043931499E-16,1.,-1.45117688885522E-12));
#41524=DIRECTION('center_axis',(0.707106781186791,0.707106781186304,-1.02850161472353E-12));
#41525=DIRECTION('ref_axis',(-0.707106781186304,0.707106781186791,-1.02377242289792E-12));
#41526=DIRECTION('center_axis',(5.00596043931499E-16,1.,-1.45117688885522E-12));
#41527=DIRECTION('ref_axis',(3.89915512223497E-15,1.45117688885522E-12,
1.));
#41528=DIRECTION('',(5.00596043931499E-16,1.,-1.45117688885522E-12));
#41529=DIRECTION('center_axis',(-0.707106781186791,-0.707106781186304,1.02850161472353E-12));
#41530=DIRECTION('ref_axis',(0.707106781186304,-0.707106781186791,1.02337989978325E-12));
#41531=DIRECTION('',(5.00596043931499E-16,1.,-1.45117688885522E-12));
#41532=DIRECTION('center_axis',(5.00596043931499E-16,1.,-1.45117688885522E-12));
#41533=DIRECTION('ref_axis',(1.,-5.00596043936352E-16,-3.34404360992166E-15));
#41534=DIRECTION('',(5.00596043931499E-16,1.,-1.45117688885522E-12));
#41535=DIRECTION('center_axis',(-0.707106781186791,-0.707106781186304,1.02850161472353E-12));
#41536=DIRECTION('ref_axis',(0.707106781186304,-0.707106781186791,1.02377242289792E-12));
#41537=DIRECTION('',(5.00596043931499E-16,1.,-1.45117688885522E-12));
#41538=DIRECTION('center_axis',(3.89915512223496E-15,1.45117688885522E-12,
1.));
#41539=DIRECTION('ref_axis',(5.00596043931499E-16,1.,-1.45117688885522E-12));
#41540=DIRECTION('',(5.00596043931499E-16,1.,-1.45117688885522E-12));
#41541=DIRECTION('',(-0.707106781186304,0.707106781186791,-1.02337989978325E-12));
#41542=DIRECTION('center_axis',(-0.707106781186791,-0.707106781186304,1.02850161472353E-12));
#41543=DIRECTION('ref_axis',(0.707106781186304,-0.707106781186791,1.02377242289792E-12));
#41544=DIRECTION('',(-3.20526573184424E-15,-1.45117688885522E-12,-1.));
#41545=DIRECTION('center_axis',(-0.707106781186791,-0.707106781186304,1.02850161472353E-12));
#41546=DIRECTION('ref_axis',(-0.707106781186304,0.707106781186791,-1.02377242289792E-12));
#41547=DIRECTION('',(3.34404360992239E-15,1.45117688885522E-12,1.));
#41548=DIRECTION('center_axis',(-0.707106781186791,-0.707106781186304,1.02850161472353E-12));
#41549=DIRECTION('ref_axis',(-0.707106781186304,0.707106781186791,-1.02377242289792E-12));
#41550=DIRECTION('',(0.707106781186304,-0.707106781186791,1.02377242289792E-12));
#41551=DIRECTION('',(0.707106781186304,-0.707106781186791,1.02367429211925E-12));
#41552=DIRECTION('center_axis',(0.707106781186791,0.707106781186304,-1.02850161472353E-12));
#41553=DIRECTION('ref_axis',(0.707106781186304,-0.707106781186791,1.02377242289792E-12));
#41554=DIRECTION('',(3.48282148800053E-15,1.45103811097714E-12,1.));
#41555=DIRECTION('center_axis',(0.707106781186791,0.707106781186304,-1.02850161472353E-12));
#41556=DIRECTION('ref_axis',(0.707106781186304,-0.707106781186791,1.02377242289792E-12));
#41557=DIRECTION('center_axis',(3.48282148800053E-15,1.45117688885522E-12,
1.));
#41558=DIRECTION('ref_axis',(5.00596043931499E-16,1.,-1.45117688885522E-12));
#41559=DIRECTION('',(5.00596043931499E-16,1.,-1.45117688885522E-12));
#41560=DIRECTION('center_axis',(5.00596043931499E-16,1.,-1.45117688885522E-12));
#41561=DIRECTION('ref_axis',(-3.34404360992239E-15,-1.45117688885522E-12,
-1.));
#41562=DIRECTION('',(5.00596043931499E-16,1.,-1.45117688885522E-12));
#41563=DIRECTION('center_axis',(5.00596043931499E-16,1.,-1.45117688885522E-12));
#41564=DIRECTION('ref_axis',(3.34404360992239E-15,1.45117688885522E-12,
1.));
#41565=DIRECTION('',(5.00596043931499E-16,1.,-1.45117688885522E-12));
#41566=DIRECTION('center_axis',(-1.,5.00596043936553E-16,3.48282148799981E-15));
#41567=DIRECTION('ref_axis',(-5.00596043931499E-16,-1.,1.45117688885522E-12));
#41568=DIRECTION('',(5.00596043931499E-16,1.,-1.45117688885522E-12));
#41569=DIRECTION('center_axis',(5.00596043931499E-16,1.,-1.45117688885522E-12));
#41570=DIRECTION('ref_axis',(1.,-5.00596043936352E-16,-3.34404360992166E-15));
#41571=DIRECTION('center_axis',(-1.,5.0059604393615E-16,3.20526573184352E-15));
#41572=DIRECTION('ref_axis',(-5.00596043931499E-16,-1.,1.45117688885522E-12));
#41573=DIRECTION('center_axis',(-3.34404360992239E-15,-1.45117688885522E-12,
-1.));
#41574=DIRECTION('ref_axis',(-5.00596043931499E-16,-1.,1.45117688885522E-12));
#41575=DIRECTION('',(5.00596043931499E-16,1.,-1.45117688885522E-12));
#41576=DIRECTION('center_axis',(5.00596043931499E-16,1.,-1.45117688885522E-12));
#41577=DIRECTION('ref_axis',(-1.,5.00596043936352E-16,3.34404360992166E-15));
#41578=DIRECTION('',(5.00596043931499E-16,1.,-1.45117688885522E-12));
#41579=DIRECTION('center_axis',(1.,-5.00596043936352E-16,-3.34404360992166E-15));
#41580=DIRECTION('ref_axis',(5.00596043931499E-16,1.,-1.45117688885522E-12));
#41581=DIRECTION('center_axis',(0.707106781186548,0.707106781186547,-1.02850161472388E-12));
#41582=DIRECTION('ref_axis',(-0.707106781186547,0.707106781186548,-1.02377242289756E-12));
#41583=DIRECTION('center_axis',(0.707106781186548,0.707106781186547,-1.02850161472388E-12));
#41584=DIRECTION('ref_axis',(-0.707106781186547,0.707106781186548,-1.02377242289756E-12));
#41585=DIRECTION('',(0.707106781186547,-0.707106781186548,1.02337989978289E-12));
#41586=DIRECTION('center_axis',(0.707106781186548,0.707106781186547,-1.02850161472388E-12));
#41587=DIRECTION('ref_axis',(0.707106781186547,-0.707106781186548,1.02377242289756E-12));
#41588=DIRECTION('',(3.20526573184424E-15,1.4513156667333E-12,1.));
#41589=DIRECTION('center_axis',(0.707106781186548,0.707106781186547,-1.02850161472388E-12));
#41590=DIRECTION('ref_axis',(0.707106781186547,-0.707106781186548,1.02337989978289E-12));
#41591=DIRECTION('',(-0.707106781186547,0.707106781186548,-1.02377242289756E-12));
#41592=DIRECTION('center_axis',(0.707106781186548,0.707106781186547,-1.02850161472388E-12));
#41593=DIRECTION('ref_axis',(-0.707106781186547,0.707106781186548,-1.02377242289756E-12));
#41594=DIRECTION('',(3.34404360992239E-15,1.45117688885522E-12,1.));
#41595=DIRECTION('',(-0.707106781186547,0.707106781186548,-1.0236742921189E-12));
#41596=DIRECTION('center_axis',(-0.707106781186548,-0.707106781186547,1.02850161472388E-12));
#41597=DIRECTION('ref_axis',(-0.707106781186547,0.707106781186548,-1.02377242289756E-12));
#41598=DIRECTION('',(3.48282148800053E-15,1.45103811097714E-12,1.));
#41599=DIRECTION('center_axis',(-0.707106781186548,-0.707106781186547,1.02850161472388E-12));
#41600=DIRECTION('ref_axis',(-0.707106781186547,0.707106781186548,-1.02377242289756E-12));
#41601=DIRECTION('',(0.707106781186547,-0.707106781186548,1.0235270959509E-12));
#41602=DIRECTION('center_axis',(-0.707106781186548,-0.707106781186547,1.02850161472388E-12));
#41603=DIRECTION('ref_axis',(0.707106781186547,-0.707106781186548,1.02377242289756E-12));
#41604=DIRECTION('',(-3.48282148800053E-15,-1.45103811097714E-12,-1.));
#41605=DIRECTION('center_axis',(-0.707106781186548,-0.707106781186547,1.02850161472388E-12));
#41606=DIRECTION('ref_axis',(0.707106781186547,-0.707106781186548,1.02377242289756E-12));
#41607=DIRECTION('center_axis',(-3.69098830511775E-15,-1.45117688885522E-12,
-1.));
#41608=DIRECTION('ref_axis',(-5.00596043931499E-16,-1.,1.45117688885522E-12));
#41609=DIRECTION('',(5.00596043931499E-16,1.,-1.45117688885522E-12));
#41610=DIRECTION('',(-0.707106781186304,-0.707106781186791,1.0287469416709E-12));
#41611=DIRECTION('',(5.00596043931499E-16,1.,-1.45117688885522E-12));
#41612=DIRECTION('center_axis',(5.00596043931499E-16,1.,-1.45117688885522E-12));
#41613=DIRECTION('ref_axis',(-1.,5.00596043936352E-16,3.34404360992166E-15));
#41614=DIRECTION('',(5.00596043931499E-16,1.,-1.45117688885522E-12));
#41615=DIRECTION('center_axis',(-0.707106781186791,0.707106781186304,-1.02377242289721E-12));
#41616=DIRECTION('ref_axis',(-0.707106781186304,-0.707106781186791,1.02850161472423E-12));
#41617=DIRECTION('center_axis',(1.,-5.00596043936553E-16,-3.48282148799981E-15));
#41618=DIRECTION('ref_axis',(5.00596043931499E-16,1.,-1.45117688885522E-12));
#41619=DIRECTION('',(5.00596043931499E-16,1.,-1.45117688885522E-12));
#41620=DIRECTION('',(-3.48282148800053E-15,-1.4513156667333E-12,-1.));
#41621=DIRECTION('center_axis',(5.00596043931499E-16,1.,-1.45117688885522E-12));
#41622=DIRECTION('ref_axis',(-3.34404360992239E-15,-1.45117688885522E-12,
-1.));
#41623=DIRECTION('',(5.00596043931499E-16,1.,-1.45117688885522E-12));
#41624=DIRECTION('center_axis',(-0.707106781186791,0.707106781186304,-1.02377242289721E-12));
#41625=DIRECTION('ref_axis',(-0.707106781186304,-0.707106781186791,1.02850161472423E-12));
#41626=DIRECTION('center_axis',(5.00596043931499E-16,1.,-1.45117688885522E-12));
#41627=DIRECTION('ref_axis',(3.89915512223497E-15,1.45117688885522E-12,
1.));
#41628=DIRECTION('',(5.00596043931499E-16,1.,-1.45117688885522E-12));
#41629=DIRECTION('center_axis',(0.707106781186791,-0.707106781186304,1.02377242289721E-12));
#41630=DIRECTION('ref_axis',(0.707106781186304,0.707106781186791,-1.02889413783891E-12));
#41631=DIRECTION('',(5.00596043931499E-16,1.,-1.45117688885522E-12));
#41632=DIRECTION('center_axis',(-1.,5.0059604393615E-16,3.20526573184352E-15));
#41633=DIRECTION('ref_axis',(-5.00596043931499E-16,-1.,1.45117688885522E-12));
#41634=DIRECTION('',(5.00596043931499E-16,1.,-1.45117688885522E-12));
#41635=DIRECTION('',(-3.20526573184424E-15,-1.45103811097714E-12,-1.));
#41636=DIRECTION('center_axis',(5.00596043931499E-16,1.,-1.45117688885522E-12));
#41637=DIRECTION('ref_axis',(1.,-5.00596043936352E-16,-3.34404360992166E-15));
#41638=DIRECTION('',(5.00596043931499E-16,1.,-1.45117688885522E-12));
#41639=DIRECTION('center_axis',(0.707106781186791,-0.707106781186304,1.02377242289721E-12));
#41640=DIRECTION('ref_axis',(0.707106781186304,0.707106781186791,-1.02850161472423E-12));
#41641=DIRECTION('center_axis',(3.89915512223496E-15,1.45117688885522E-12,
1.));
#41642=DIRECTION('ref_axis',(5.00596043931499E-16,1.,-1.45117688885522E-12));
#41643=DIRECTION('',(5.00596043931499E-16,1.,-1.45117688885522E-12));
#41644=DIRECTION('',(-0.707106781186304,-0.707106781186791,1.02889413783891E-12));
#41645=DIRECTION('center_axis',(0.707106781186791,-0.707106781186304,1.02377242289721E-12));
#41646=DIRECTION('ref_axis',(0.707106781186304,0.707106781186791,-1.02850161472423E-12));
#41647=DIRECTION('center_axis',(0.707106781186791,-0.707106781186304,1.02377242289721E-12));
#41648=DIRECTION('ref_axis',(-0.707106781186304,-0.707106781186791,1.02850161472423E-12));
#41649=DIRECTION('',(3.34404360992239E-15,1.45117688885522E-12,1.));
#41650=DIRECTION('center_axis',(0.707106781186791,-0.707106781186304,1.02377242289721E-12));
#41651=DIRECTION('ref_axis',(-0.707106781186304,-0.707106781186791,1.02850161472423E-12));
#41652=DIRECTION('',(0.707106781186304,0.707106781186791,-1.02850161472423E-12));
#41653=DIRECTION('',(0.707106781186304,0.707106781186791,-1.0285997455029E-12));
#41654=DIRECTION('center_axis',(-0.707106781186791,0.707106781186304,-1.02377242289721E-12));
#41655=DIRECTION('ref_axis',(0.707106781186304,0.707106781186791,-1.02850161472423E-12));
#41656=DIRECTION('',(3.48282148800053E-15,1.4513156667333E-12,1.));
#41657=DIRECTION('center_axis',(-0.707106781186791,0.707106781186304,-1.02377242289721E-12));
#41658=DIRECTION('ref_axis',(0.707106781186304,0.707106781186791,-1.02850161472423E-12));
#41659=DIRECTION('center_axis',(3.48282148800053E-15,1.45117688885522E-12,
1.));
#41660=DIRECTION('ref_axis',(5.00596043931499E-16,1.,-1.45117688885522E-12));
#41661=DIRECTION('',(5.00596043931499E-16,1.,-1.45117688885522E-12));
#41662=DIRECTION('center_axis',(5.00596043931499E-16,1.,-1.45117688885522E-12));
#41663=DIRECTION('ref_axis',(-3.34404360992239E-15,-1.45117688885522E-12,
-1.));
#41664=DIRECTION('',(5.00596043931499E-16,1.,-1.45117688885522E-12));
#41665=DIRECTION('center_axis',(5.00596043931499E-16,1.,-1.45117688885522E-12));
#41666=DIRECTION('ref_axis',(3.34404360992239E-15,1.45117688885522E-12,
1.));
#41667=DIRECTION('',(5.00596043931499E-16,1.,-1.45117688885522E-12));
#41668=DIRECTION('center_axis',(-1.,5.00596043936553E-16,3.48282148799981E-15));
#41669=DIRECTION('ref_axis',(-5.00596043931499E-16,-1.,1.45117688885522E-12));
#41670=DIRECTION('',(5.00596043931499E-16,1.,-1.45117688885522E-12));
#41671=DIRECTION('center_axis',(5.00596043931499E-16,1.,-1.45117688885522E-12));
#41672=DIRECTION('ref_axis',(1.,-5.00596043936352E-16,-3.34404360992166E-15));
#41673=DIRECTION('center_axis',(-3.34404360992239E-15,-1.45117688885522E-12,
-1.));
#41674=DIRECTION('ref_axis',(-5.00596043931499E-16,-1.,1.45117688885522E-12));
#41675=DIRECTION('',(5.00596043931499E-16,1.,-1.45117688885522E-12));
#41676=DIRECTION('center_axis',(5.00596043931499E-16,1.,-1.45117688885522E-12));
#41677=DIRECTION('ref_axis',(-1.,5.00596043936352E-16,3.34404360992166E-15));
#41678=DIRECTION('',(5.00596043931499E-16,1.,-1.45117688885522E-12));
#41679=DIRECTION('center_axis',(1.,-5.00596043936352E-16,-3.34404360992166E-15));
#41680=DIRECTION('ref_axis',(5.00596043931499E-16,1.,-1.45117688885522E-12));
#41681=DIRECTION('center_axis',(-0.707106781186792,0.707106781186303,-1.02360964389904E-12));
#41682=DIRECTION('ref_axis',(-8.58100867314579E-13,5.89501773663249E-13,
1.));
#41683=DIRECTION('',(0.707106781186303,0.707106781186792,-4.19016418634642E-13));
#41684=DIRECTION('center_axis',(-0.707106781186792,0.707106781186303,-1.02360964389904E-12));
#41685=DIRECTION('ref_axis',(0.707106781186303,0.707106781186792,-4.19016418634642E-13));
#41686=DIRECTION('',(-8.58367982497838E-13,5.89234658479989E-13,1.));
#41687=DIRECTION('center_axis',(-0.707106781186792,0.707106781186303,-1.02360964389904E-12));
#41688=DIRECTION('ref_axis',(0.707106781186303,0.707106781186792,-4.18623895519971E-13));
#41689=DIRECTION('',(-0.707106781186303,-0.707106781186792,4.1911454941331E-13));
#41690=DIRECTION('center_axis',(-0.707106781186792,0.707106781186303,-1.02360964389904E-12));
#41691=DIRECTION('ref_axis',(-0.707106781186303,-0.707106781186792,4.19016418634642E-13));
#41692=DIRECTION('',(-3.34404360992195E-15,-5.88679546967676E-13,-1.));
#41693=DIRECTION('center_axis',(-0.707106781186792,0.707106781186303,-1.02360964389904E-12));
#41694=DIRECTION('ref_axis',(-0.707106781186303,-0.707106781186792,4.19016418634642E-13));
#41695=DIRECTION('',(-8.58506760375916E-13,5.89095880601911E-13,1.));
#41696=DIRECTION('center_axis',(0.707106781186792,-0.707106781186303,1.02360964389904E-12));
#41697=DIRECTION('ref_axis',(-0.707106781186303,-0.707106781186792,4.19016418634642E-13));
#41698=DIRECTION('',(0.707106781186303,0.707106781186792,-4.18918287855974E-13));
#41699=DIRECTION('center_axis',(0.707106781186792,-0.707106781186303,1.02360964389904E-12));
#41700=DIRECTION('ref_axis',(0.707106781186303,0.707106781186792,-4.19016418634642E-13));
#41701=DIRECTION('',(8.58714927193033E-13,-5.88887713784794E-13,-1.));
#41702=DIRECTION('center_axis',(0.707106781186792,-0.707106781186303,1.02360964389904E-12));
#41703=DIRECTION('ref_axis',(0.707106781186303,0.707106781186792,-4.19016418634642E-13));
#41704=DIRECTION('',(-0.707106781186303,-0.707106781186792,4.18918287855974E-13));
#41705=DIRECTION('center_axis',(0.707106781186792,-0.707106781186303,1.02360964389904E-12));
#41706=DIRECTION('ref_axis',(-0.707106781186303,-0.707106781186792,4.19016418634642E-13));
#41707=DIRECTION('center_axis',(-5.00596043934383E-16,-1.,5.88887713784794E-13));
#41708=DIRECTION('ref_axis',(-1.,5.00596043936352E-16,3.34404360992166E-15));
#41709=DIRECTION('',(-1.,5.00596043936352E-16,3.34404360992166E-15));
#41710=DIRECTION('',(8.65180980907738E-13,5.88887713784793E-13,1.));
#41711=DIRECTION('',(-1.,5.00596043936352E-16,3.34404360992166E-15));
#41712=DIRECTION('center_axis',(1.,-5.00596043936352E-16,-3.34404360992166E-15));
#41713=DIRECTION('ref_axis',(5.00596043934382E-16,1.,-5.89234658479989E-13));
#41714=DIRECTION('',(-1.,5.00596043936352E-16,3.34404360992166E-15));
#41715=DIRECTION('center_axis',(-0.707106781186791,-0.707106781186304,1.02818183432823E-12));
#41716=DIRECTION('ref_axis',(-0.707106781186304,0.707106781186791,-4.14287226808325E-13));
#41717=DIRECTION('center_axis',(-3.34404360992196E-15,-5.89095880601911E-13,
-1.));
#41718=DIRECTION('ref_axis',(-1.,5.00596043936352E-16,3.34404360992166E-15));
#41719=DIRECTION('',(-1.,5.00596043936352E-16,3.34404360992166E-15));
#41720=DIRECTION('',(0.707106781186304,-0.707106781186791,4.14189096029657E-13));
#41721=DIRECTION('center_axis',(1.,-5.00596043936352E-16,-3.34404360992166E-15));
#41722=DIRECTION('ref_axis',(3.34404360992196E-15,5.89234658479989E-13,
1.));
#41723=DIRECTION('',(-1.,5.00596043936352E-16,3.34404360992166E-15));
#41724=DIRECTION('center_axis',(-0.707106781186791,-0.707106781186304,1.02818183432823E-12));
#41725=DIRECTION('ref_axis',(0.707106781186304,-0.707106781186791,4.14287226808325E-13));
#41726=DIRECTION('center_axis',(-3.34404360992196E-15,-5.89373436358067E-13,
-1.));
#41727=DIRECTION('ref_axis',(-1.,5.00596043936352E-16,3.34404360992166E-15));
#41728=DIRECTION('',(-1.,5.00596043936352E-16,3.34404360992166E-15));
#41729=DIRECTION('',(-0.707106781186304,0.707106781186791,-4.14385357586993E-13));
#41730=DIRECTION('',(-1.,5.00596043936352E-16,3.34404360992166E-15));
#41731=DIRECTION('center_axis',(1.,-5.00596043936352E-16,-3.34404360992166E-15));
#41732=DIRECTION('ref_axis',(5.00596043934384E-16,1.,-5.88679546967676E-13));
#41733=DIRECTION('',(-1.,5.00596043936352E-16,3.34404360992166E-15));
#41734=DIRECTION('center_axis',(0.707106781186791,0.707106781186304,-1.02818183432823E-12));
#41735=DIRECTION('ref_axis',(-0.707106781186304,0.707106781186791,-4.13894703693654E-13));
#41736=DIRECTION('center_axis',(-5.00596043934382E-16,-1.,5.89234658479989E-13));
#41737=DIRECTION('ref_axis',(-1.,5.00596043936352E-16,3.34404360992166E-15));
#41738=DIRECTION('',(1.,-5.00596043936352E-16,-3.34404360992166E-15));
#41739=DIRECTION('',(-8.64834036212544E-13,-5.89234658479989E-13,-1.));
#41740=DIRECTION('center_axis',(1.,-5.00596043936352E-16,-3.34404360992166E-15));
#41741=DIRECTION('ref_axis',(-3.34404360992196E-15,-5.89234658479989E-13,
-1.));
#41742=DIRECTION('',(-1.,5.00596043936352E-16,3.34404360992166E-15));
#41743=DIRECTION('center_axis',(0.707106781186791,0.707106781186304,-1.02818183432823E-12));
#41744=DIRECTION('ref_axis',(-0.707106781186304,0.707106781186791,-4.14287226808325E-13));
#41745=DIRECTION('center_axis',(0.707106781186791,0.707106781186304,-1.02818183432823E-12));
#41746=DIRECTION('ref_axis',(-8.64855573465793E-13,-5.89213121226739E-13,
-1.));
#41747=DIRECTION('',(0.707106781186304,-0.707106781186791,4.14287226808325E-13));
#41748=DIRECTION('center_axis',(0.707106781186791,0.707106781186304,-1.02818183432823E-12));
#41749=DIRECTION('ref_axis',(0.707106781186304,-0.707106781186791,4.14287226808325E-13));
#41750=DIRECTION('',(-3.34404360992195E-15,-5.88679546967676E-13,-1.));
#41751=DIRECTION('center_axis',(0.707106781186791,0.707106781186304,-1.02818183432823E-12));
#41752=DIRECTION('ref_axis',(0.707106781186304,-0.707106781186791,4.14287226808325E-13));
#41753=DIRECTION('',(-8.64972814090621E-13,-5.8909588060191E-13,-1.));
#41754=DIRECTION('center_axis',(-0.707106781186791,-0.707106781186304,1.02818183432823E-12));
#41755=DIRECTION('ref_axis',(0.707106781186304,-0.707106781186791,4.14287226808325E-13));
#41756=DIRECTION('',(-0.707106781186304,0.707106781186791,-4.14189096029657E-13));
#41757=DIRECTION('center_axis',(-0.707106781186791,-0.707106781186304,1.02818183432823E-12));
#41758=DIRECTION('ref_axis',(-0.707106781186304,0.707106781186791,-4.14287226808325E-13));
#41759=DIRECTION('center_axis',(5.00596043934382E-16,1.,-5.89095880601911E-13));
#41760=DIRECTION('ref_axis',(1.,-5.00596043936352E-16,-3.34404360992166E-15));
#41761=DIRECTION('',(-1.,5.00596043936352E-16,3.34404360992166E-15));
#41762=DIRECTION('center_axis',(3.34404360992196E-15,5.89234658479989E-13,
1.));
#41763=DIRECTION('ref_axis',(1.,-5.00596043936352E-16,-3.34404360992166E-15));
#41764=DIRECTION('',(-1.,5.00596043936352E-16,3.34404360992166E-15));
#41765=DIRECTION('center_axis',(1.,-5.00596043936352E-16,-3.34404360992166E-15));
#41766=DIRECTION('ref_axis',(-3.34404360992196E-15,-5.89234658479989E-13,
-1.));
#41767=DIRECTION('',(-1.,5.00596043936352E-16,3.34404360992166E-15));
#41768=DIRECTION('center_axis',(3.34404360992196E-15,5.89095880601911E-13,
1.));
#41769=DIRECTION('ref_axis',(1.,-5.00596043936352E-16,-3.34404360992166E-15));
#41770=DIRECTION('',(1.,-5.00596043936352E-16,-3.34404360992166E-15));
#41771=DIRECTION('center_axis',(1.,-5.00596043936352E-16,-3.34404360992166E-15));
#41772=DIRECTION('ref_axis',(-5.00596043934382E-16,-1.,5.89234658479989E-13));
#41773=DIRECTION('center_axis',(1.,-5.00596043936352E-16,-3.34404360992166E-15));
#41774=DIRECTION('ref_axis',(-5.00596043934382E-16,-1.,5.89234658479989E-13));
#41775=DIRECTION('',(-1.,5.00596043936352E-16,3.34404360992166E-15));
#41776=DIRECTION('center_axis',(5.00596043934384E-16,1.,-5.88679546967676E-13));
#41777=DIRECTION('ref_axis',(1.,-5.00596043936352E-16,-3.34404360992166E-15));
#41778=DIRECTION('',(-1.,5.00596043936352E-16,3.34404360992166E-15));
#41779=DIRECTION('center_axis',(1.,-5.00596043936352E-16,-3.34404360992166E-15));
#41780=DIRECTION('ref_axis',(3.34404360992196E-15,5.89234658479989E-13,
1.));
#41781=DIRECTION('center_axis',(-0.707106781186547,-0.707106781186548,1.02850161472388E-12));
#41782=DIRECTION('ref_axis',(3.34404360992239E-15,1.45117688885522E-12,
1.));
#41783=DIRECTION('',(0.707106781186548,-0.707106781186547,1.02377242289756E-12));
#41784=DIRECTION('center_axis',(-0.707106781186547,-0.707106781186548,1.02850161472388E-12));
#41785=DIRECTION('ref_axis',(0.707106781186548,-0.707106781186547,1.02377242289756E-12));
#41786=DIRECTION('',(-2.78893209760981E-15,-1.45173200036753E-12,-1.));
#41787=DIRECTION('center_axis',(-0.707106781186547,-0.707106781186548,1.02850161472388E-12));
#41788=DIRECTION('ref_axis',(0.707106781186548,-0.707106781186547,1.02377242289756E-12));
#41789=DIRECTION('',(-0.707106781186548,0.707106781186547,-1.0236742921189E-12));
#41790=DIRECTION('center_axis',(-0.707106781186547,-0.707106781186548,1.02850161472388E-12));
#41791=DIRECTION('ref_axis',(-0.707106781186548,0.707106781186547,-1.02416494601223E-12));
#41792=DIRECTION('',(-3.34404360992239E-15,-1.45117688885522E-12,-1.));
#41793=DIRECTION('center_axis',(-0.707106781186547,-0.707106781186548,1.02850161472388E-12));
#41794=DIRECTION('ref_axis',(-0.707106781186548,0.707106781186547,-1.02377242289756E-12));
#41795=DIRECTION('',(3.20526573184424E-15,1.4513156667333E-12,1.));
#41796=DIRECTION('center_axis',(0.707106781186547,0.707106781186548,-1.02850161472388E-12));
#41797=DIRECTION('ref_axis',(0.707106781186548,-0.707106781186547,1.02377242289756E-12));
#41798=DIRECTION('',(-0.707106781186548,0.707106781186547,-1.02387055367623E-12));
#41799=DIRECTION('center_axis',(0.707106781186547,0.707106781186548,-1.02850161472388E-12));
#41800=DIRECTION('ref_axis',(-0.707106781186548,0.707106781186547,-1.02377242289756E-12));
#41801=DIRECTION('',(-2.99709891472702E-15,-1.45152383355042E-12,-1.));
#41802=DIRECTION('center_axis',(0.707106781186547,0.707106781186548,-1.02850161472388E-12));
#41803=DIRECTION('ref_axis',(-0.707106781186548,0.707106781186547,-1.02377242289756E-12));
#41804=DIRECTION('',(0.707106781186548,-0.707106781186547,1.02387055367623E-12));
#41805=DIRECTION('center_axis',(0.707106781186547,0.707106781186548,-1.02850161472388E-12));
#41806=DIRECTION('ref_axis',(0.707106781186548,-0.707106781186547,1.02377242289756E-12));
#41807=DIRECTION('center_axis',(-5.00596043931498E-16,-1.,1.45152383355042E-12));
#41808=DIRECTION('ref_axis',(1.,-5.00596043936352E-16,-3.34404360992166E-15));
#41809=DIRECTION('',(-1.,5.00596043936352E-16,3.34404360992166E-15));
#41810=DIRECTION('',(3.69098830511775E-15,1.45152383355042E-12,1.));
#41811=DIRECTION('',(-1.,5.00596043936352E-16,3.34404360992166E-15));
#41812=DIRECTION('center_axis',(-1.,5.00596043936352E-16,3.34404360992166E-15));
#41813=DIRECTION('ref_axis',(3.34404360992239E-15,1.45117688885522E-12,
1.));
#41814=DIRECTION('',(-1.,5.00596043936352E-16,3.34404360992166E-15));
#41815=DIRECTION('center_axis',(-0.707106781186547,0.707106781186548,-1.02377242289756E-12));
#41816=DIRECTION('ref_axis',(0.707106781186548,0.707106781186547,-1.02850161472388E-12));
#41817=DIRECTION('center_axis',(-3.34404360992239E-15,-1.4513156667333E-12,
-1.));
#41818=DIRECTION('ref_axis',(-1.,5.00596043936352E-16,3.34404360992166E-15));
#41819=DIRECTION('',(-1.,5.00596043936352E-16,3.34404360992166E-15));
#41820=DIRECTION('',(-0.707106781186548,-0.707106781186547,1.02859974550255E-12));
#41821=DIRECTION('center_axis',(-1.,5.00596043936352E-16,3.34404360992166E-15));
#41822=DIRECTION('ref_axis',(-5.00596043931499E-16,-1.,1.45117688885522E-12));
#41823=DIRECTION('',(-1.,5.00596043936352E-16,3.34404360992166E-15));
#41824=DIRECTION('center_axis',(-0.707106781186547,0.707106781186548,-1.02377242289756E-12));
#41825=DIRECTION('ref_axis',(-0.707106781186548,-0.707106781186547,1.02850161472388E-12));
#41826=DIRECTION('center_axis',(3.34404360992239E-15,1.45103811097714E-12,
1.));
#41827=DIRECTION('ref_axis',(1.,-5.00596043936352E-16,-3.34404360992166E-15));
#41828=DIRECTION('',(-1.,5.00596043936352E-16,3.34404360992166E-15));
#41829=DIRECTION('',(-0.707106781186548,-0.707106781186547,1.02840348394521E-12));
#41830=DIRECTION('',(-1.,5.00596043936352E-16,3.34404360992166E-15));
#41831=DIRECTION('center_axis',(-1.,5.00596043936352E-16,3.34404360992166E-15));
#41832=DIRECTION('ref_axis',(-3.34404360992239E-15,-1.45117688885522E-12,
-1.));
#41833=DIRECTION('',(-1.,5.00596043936352E-16,3.34404360992166E-15));
#41834=DIRECTION('center_axis',(0.707106781186547,-0.707106781186548,1.02377242289756E-12));
#41835=DIRECTION('ref_axis',(-0.707106781186548,-0.707106781186547,1.02850161472388E-12));
#41836=DIRECTION('center_axis',(5.00596043931497E-16,1.,-1.45173200036753E-12));
#41837=DIRECTION('ref_axis',(-1.,5.00596043936352E-16,3.34404360992166E-15));
#41838=DIRECTION('',(-1.,5.00596043936352E-16,3.34404360992166E-15));
#41839=DIRECTION('',(3.89915512223497E-15,1.45173200036753E-12,1.));
#41840=DIRECTION('center_axis',(-1.,5.00596043936352E-16,3.34404360992166E-15));
#41841=DIRECTION('ref_axis',(-5.00596043931499E-16,-1.,1.45117688885522E-12));
#41842=DIRECTION('',(-1.,5.00596043936352E-16,3.34404360992166E-15));
#41843=DIRECTION('center_axis',(0.707106781186547,-0.707106781186548,1.02377242289756E-12));
#41844=DIRECTION('ref_axis',(-0.707106781186548,-0.707106781186547,1.02850161472388E-12));
#41845=DIRECTION('center_axis',(0.707106781186547,-0.707106781186548,1.02377242289756E-12));
#41846=DIRECTION('ref_axis',(-3.34404360992239E-15,-1.45117688885522E-12,
-1.));
#41847=DIRECTION('',(0.707106781186548,0.707106781186547,-1.02850161472388E-12));
#41848=DIRECTION('center_axis',(0.707106781186547,-0.707106781186548,1.02377242289756E-12));
#41849=DIRECTION('ref_axis',(0.707106781186548,0.707106781186547,-1.02850161472388E-12));
#41850=DIRECTION('',(-3.34404360992239E-15,-1.45117688885522E-12,-1.));
#41851=DIRECTION('center_axis',(0.707106781186547,-0.707106781186548,1.02377242289756E-12));
#41852=DIRECTION('ref_axis',(0.707106781186548,0.707106781186547,-1.02889413783855E-12));
#41853=DIRECTION('',(-3.48282148800053E-15,-1.4513156667333E-12,-1.));
#41854=DIRECTION('center_axis',(-0.707106781186547,0.707106781186548,-1.02377242289756E-12));
#41855=DIRECTION('ref_axis',(-0.707106781186548,-0.707106781186547,1.02850161472388E-12));
#41856=DIRECTION('',(0.707106781186548,0.707106781186547,-1.02859974550255E-12));
#41857=DIRECTION('center_axis',(-0.707106781186547,0.707106781186548,-1.02377242289756E-12));
#41858=DIRECTION('ref_axis',(0.707106781186548,0.707106781186547,-1.02850161472388E-12));
#41859=DIRECTION('center_axis',(5.00596043931499E-16,1.,-1.4513156667333E-12));
#41860=DIRECTION('ref_axis',(-1.,5.00596043936352E-16,3.34404360992166E-15));
#41861=DIRECTION('',(-1.,5.00596043936352E-16,3.34404360992166E-15));
#41862=DIRECTION('center_axis',(-3.34404360992239E-15,-1.45117688885522E-12,
-1.));
#41863=DIRECTION('ref_axis',(-1.,5.00596043936352E-16,3.34404360992166E-15));
#41864=DIRECTION('',(-1.,5.00596043936352E-16,3.34404360992166E-15));
#41865=DIRECTION('center_axis',(-1.,5.00596043936352E-16,3.34404360992166E-15));
#41866=DIRECTION('ref_axis',(5.00596043931499E-16,1.,-1.45117688885522E-12));
#41867=DIRECTION('',(-1.,5.00596043936352E-16,3.34404360992166E-15));
#41868=DIRECTION('center_axis',(3.34404360992239E-15,1.4513156667333E-12,
1.));
#41869=DIRECTION('ref_axis',(1.,-5.00596043936352E-16,-3.34404360992166E-15));
#41870=DIRECTION('',(-1.,5.00596043936352E-16,3.34404360992166E-15));
#41871=DIRECTION('center_axis',(-1.,5.00596043936352E-16,3.34404360992166E-15));
#41872=DIRECTION('ref_axis',(-3.34404360992239E-15,-1.45117688885522E-12,
-1.));
#41873=DIRECTION('center_axis',(-1.,5.00596043936352E-16,3.34404360992166E-15));
#41874=DIRECTION('ref_axis',(5.00596043931497E-16,1.,-1.45173200036753E-12));
#41875=DIRECTION('',(-1.,5.00596043936352E-16,3.34404360992166E-15));
#41876=DIRECTION('center_axis',(-5.00596043931499E-16,-1.,1.45117688885522E-12));
#41877=DIRECTION('ref_axis',(1.,-5.00596043936352E-16,-3.34404360992166E-15));
#41878=DIRECTION('',(-1.,5.00596043936352E-16,3.34404360992166E-15));
#41879=DIRECTION('center_axis',(-1.,5.00596043936352E-16,3.34404360992166E-15));
#41880=DIRECTION('ref_axis',(3.34404360992239E-15,1.45117688885522E-12,
1.));
#41881=DIRECTION('center_axis',(-5.00596043934463E-16,-1.,-1.46803972383759E-15));
#41882=DIRECTION('ref_axis',(-1.,5.00596043934458E-16,3.60315789384389E-15));
#41883=DIRECTION('',(-3.60315789384389E-15,1.46803972383759E-15,-1.));
#41884=DIRECTION('',(1.,-5.00596043934458E-16,-3.60315789384389E-15));
#41885=DIRECTION('',(-3.60315789384389E-15,1.46803972383759E-15,-1.));
#41886=DIRECTION('',(1.,-5.00596043934458E-16,-3.60315789384389E-15));
#41887=DIRECTION('center_axis',(1.,-5.00596043934458E-16,-3.60315789384389E-15));
#41888=DIRECTION('ref_axis',(5.00596043934462E-16,1.,1.12109502864223E-15));
#41889=DIRECTION('center_axis',(1.,-5.00596043934458E-16,-3.60315789384389E-15));
#41890=DIRECTION('ref_axis',(5.00596043934462E-16,1.,1.12109502864223E-15));
#41891=DIRECTION('',(1.,-5.00596043934458E-16,-3.60315789384389E-15));
#41892=DIRECTION('center_axis',(1.,-5.00596043934458E-16,-3.60315789384389E-15));
#41893=DIRECTION('ref_axis',(5.00596043934462E-16,1.,1.12109502864223E-15));
#41894=DIRECTION('center_axis',(-3.60315789384389E-15,1.25987290672038E-15,
-1.));
#41895=DIRECTION('ref_axis',(-1.,5.00596043934458E-16,3.60315789384389E-15));
#41896=DIRECTION('',(5.00596043934463E-16,1.,1.25987290672037E-15));
#41897=DIRECTION('',(1.,-5.00596043934458E-16,-3.60315789384389E-15));
#41898=DIRECTION('',(5.00596043934463E-16,1.,1.25987290672037E-15));
#41899=DIRECTION('center_axis',(1.,-5.00596043934458E-16,-3.60315789384389E-15));
#41900=DIRECTION('ref_axis',(3.60315789384389E-15,-1.12109502864223E-15,
1.));
#41901=DIRECTION('center_axis',(1.,-5.00596043934458E-16,-3.60315789384389E-15));
#41902=DIRECTION('ref_axis',(3.60315789384389E-15,-1.12109502864223E-15,
1.));
#41903=DIRECTION('',(1.,-5.00596043934458E-16,-3.60315789384389E-15));
#41904=DIRECTION('center_axis',(1.,-5.00596043934458E-16,-3.60315789384389E-15));
#41905=DIRECTION('ref_axis',(3.60315789384389E-15,-1.12109502864223E-15,
1.));
#41906=DIRECTION('center_axis',(-3.60315789384389E-15,9.82317150564085E-16,
-1.));
#41907=DIRECTION('ref_axis',(-1.,5.00596043934458E-16,3.60315789384389E-15));
#41908=DIRECTION('',(-5.00596043934462E-16,-1.,-9.82317150564083E-16));
#41909=DIRECTION('',(1.,-5.00596043934458E-16,-3.60315789384389E-15));
#41910=DIRECTION('',(-5.00596043934462E-16,-1.,-9.82317150564083E-16));
#41911=DIRECTION('',(1.,-5.00596043934458E-16,-3.60315789384389E-15));
#41912=DIRECTION('center_axis',(1.,-5.00596043934458E-16,-3.60315789384389E-15));
#41913=DIRECTION('ref_axis',(5.00596043934464E-16,1.,1.67620654095481E-15));
#41914=DIRECTION('center_axis',(-1.,5.00596043934458E-16,3.60315789384389E-15));
#41915=DIRECTION('ref_axis',(5.00596043934464E-16,1.,1.67620654095481E-15));
#41916=DIRECTION('',(1.,-5.00596043934458E-16,-3.60315789384389E-15));
#41917=DIRECTION('center_axis',(-1.,5.00596043934458E-16,3.60315789384389E-15));
#41918=DIRECTION('ref_axis',(5.00596043934464E-16,1.,1.67620654095481E-15));
#41919=DIRECTION('center_axis',(-5.00596043934462E-16,-1.,-1.12109502864223E-15));
#41920=DIRECTION('ref_axis',(-1.,5.00596043934458E-16,3.60315789384389E-15));
#41921=DIRECTION('',(3.60315789384389E-15,-1.12109502864223E-15,1.));
#41922=DIRECTION('',(1.,-5.00596043934458E-16,-3.60315789384389E-15));
#41923=DIRECTION('',(3.60315789384389E-15,-1.12109502864223E-15,1.));
#41924=DIRECTION('center_axis',(1.,-5.00596043934458E-16,-3.60315789384389E-15));
#41925=DIRECTION('ref_axis',(-3.60315789384389E-15,1.12109502864223E-15,
-1.));
#41926=DIRECTION('center_axis',(-1.,5.00596043934458E-16,3.60315789384389E-15));
#41927=DIRECTION('ref_axis',(-3.60315789384389E-15,1.12109502864223E-15,
-1.));
#41928=DIRECTION('',(1.,-5.00596043934458E-16,-3.60315789384389E-15));
#41929=DIRECTION('center_axis',(-1.,5.00596043934458E-16,3.60315789384389E-15));
#41930=DIRECTION('ref_axis',(-3.60315789384389E-15,1.12109502864223E-15,
-1.));
#41931=DIRECTION('center_axis',(5.00596043934463E-16,1.,1.25987290672037E-15));
#41932=DIRECTION('ref_axis',(1.,-5.00596043934458E-16,-3.60315789384389E-15));
#41933=DIRECTION('',(3.60315789384389E-15,-1.25987290672038E-15,1.));
#41934=DIRECTION('',(1.,-5.00596043934458E-16,-3.60315789384389E-15));
#41935=DIRECTION('',(3.60315789384389E-15,-1.25987290672038E-15,1.));
#41936=DIRECTION('center_axis',(1.,-5.00596043934458E-16,-3.60315789384389E-15));
#41937=DIRECTION('ref_axis',(-3.60315789384389E-15,1.12109502864223E-15,
-1.));
#41938=DIRECTION('center_axis',(1.,-5.00596043934458E-16,-3.60315789384389E-15));
#41939=DIRECTION('ref_axis',(-3.60315789384389E-15,1.12109502864223E-15,
-1.));
#41940=DIRECTION('center_axis',(1.,-5.00596043934458E-16,-3.60315789384389E-15));
#41941=DIRECTION('ref_axis',(-3.60315789384389E-15,1.12109502864223E-15,
-1.));
#41942=DIRECTION('',(1.,-5.00596043934458E-16,-3.60315789384389E-15));
#41943=DIRECTION('center_axis',(3.60315789384389E-15,-1.25987290672038E-15,
1.));
#41944=DIRECTION('ref_axis',(1.,-5.00596043934458E-16,-3.60315789384389E-15));
#41945=DIRECTION('',(-5.00596043934463E-16,-1.,-1.25987290672037E-15));
#41946=DIRECTION('',(-5.00596043934463E-16,-1.,-1.25987290672037E-15));
#41947=DIRECTION('',(1.,-5.00596043934458E-16,-3.60315789384389E-15));
#41948=DIRECTION('center_axis',(1.,-5.00596043934458E-16,-3.60315789384389E-15));
#41949=DIRECTION('ref_axis',(-5.00596043934462E-16,-1.,-1.12109502864223E-15));
#41950=DIRECTION('center_axis',(1.,-5.00596043934458E-16,-3.60315789384389E-15));
#41951=DIRECTION('ref_axis',(-5.00596043934462E-16,-1.,-1.12109502864223E-15));
#41952=DIRECTION('center_axis',(1.,-5.00596043934458E-16,-3.60315789384389E-15));
#41953=DIRECTION('ref_axis',(-5.00596043934462E-16,-1.,-1.12109502864223E-15));
#41954=DIRECTION('center_axis',(3.60315789384389E-15,-1.12109502864223E-15,
1.));
#41955=DIRECTION('ref_axis',(1.,-5.00596043934458E-16,-3.60315789384389E-15));
#41956=DIRECTION('',(5.00596043934462E-16,1.,1.12109502864223E-15));
#41957=DIRECTION('',(1.,-5.00596043934458E-16,-3.60315789384389E-15));
#41958=DIRECTION('',(5.00596043934462E-16,1.,1.12109502864223E-15));
#41959=DIRECTION('center_axis',(1.,-5.00596043934458E-16,-3.60315789384389E-15));
#41960=DIRECTION('ref_axis',(-5.00596043934462E-16,-1.,-1.12109502864223E-15));
#41961=DIRECTION('center_axis',(-1.,5.00596043934458E-16,3.60315789384389E-15));
#41962=DIRECTION('ref_axis',(-5.00596043934462E-16,-1.,-1.12109502864223E-15));
#41963=DIRECTION('',(1.,-5.00596043934458E-16,-3.60315789384389E-15));
#41964=DIRECTION('center_axis',(-1.,5.00596043934458E-16,3.60315789384389E-15));
#41965=DIRECTION('ref_axis',(-5.00596043934462E-16,-1.,-1.12109502864223E-15));
#41966=DIRECTION('center_axis',(5.00596043934464E-16,1.,1.67620654095481E-15));
#41967=DIRECTION('ref_axis',(1.,-5.00596043934458E-16,-3.60315789384389E-15));
#41968=DIRECTION('',(-3.60315789384389E-15,1.67620654095481E-15,-1.));
#41969=DIRECTION('',(1.,-5.00596043934458E-16,-3.60315789384389E-15));
#41970=DIRECTION('',(-3.60315789384389E-15,1.67620654095481E-15,-1.));
#41971=DIRECTION('center_axis',(1.,-5.00596043934458E-16,-3.60315789384389E-15));
#41972=DIRECTION('ref_axis',(3.60315789384389E-15,-1.12109502864223E-15,
1.));
#41973=DIRECTION('center_axis',(-1.,5.00596043934458E-16,3.60315789384389E-15));
#41974=DIRECTION('ref_axis',(3.60315789384389E-15,-1.12109502864223E-15,
1.));
#41975=DIRECTION('center_axis',(-1.,5.00596043934458E-16,3.60315789384389E-15));
#41976=DIRECTION('ref_axis',(3.60315789384389E-15,-1.12109502864223E-15,
1.));
#41977=DIRECTION('center_axis',(1.,-5.00596043934458E-16,-3.60315789384389E-15));
#41978=DIRECTION('ref_axis',(-3.60315789384389E-15,1.12109502864223E-15,
-1.));
#41979=DIRECTION('center_axis',(1.,-5.00596043934458E-16,-3.60315789384389E-15));
#41980=DIRECTION('ref_axis',(-3.60315789384389E-15,1.12109502864223E-15,
-1.));
#41981=DIRECTION('center_axis',(-5.00596043934463E-16,-1.,-1.46803972383759E-15));
#41982=DIRECTION('ref_axis',(-1.,5.00596043934458E-16,3.60315789384389E-15));
#41983=DIRECTION('',(-3.60315789384389E-15,1.46803972383759E-15,-1.));
#41984=DIRECTION('',(1.,-5.00596043934458E-16,-3.60315789384389E-15));
#41985=DIRECTION('',(-3.60315789384389E-15,1.46803972383759E-15,-1.));
#41986=DIRECTION('',(1.,-5.00596043934458E-16,-3.60315789384389E-15));
#41987=DIRECTION('center_axis',(1.,-5.00596043934458E-16,-3.60315789384389E-15));
#41988=DIRECTION('ref_axis',(5.00596043934462E-16,1.,1.12109502864223E-15));
#41989=DIRECTION('center_axis',(1.,-5.00596043934458E-16,-3.60315789384389E-15));
#41990=DIRECTION('ref_axis',(5.00596043934462E-16,1.,1.12109502864223E-15));
#41991=DIRECTION('',(1.,-5.00596043934458E-16,-3.60315789384389E-15));
#41992=DIRECTION('center_axis',(1.,-5.00596043934458E-16,-3.60315789384389E-15));
#41993=DIRECTION('ref_axis',(5.00596043934462E-16,1.,1.12109502864223E-15));
#41994=DIRECTION('center_axis',(-3.60315789384389E-15,1.25987290672038E-15,
-1.));
#41995=DIRECTION('ref_axis',(-1.,5.00596043934458E-16,3.60315789384389E-15));
#41996=DIRECTION('',(5.00596043934463E-16,1.,1.25987290672037E-15));
#41997=DIRECTION('',(1.,-5.00596043934458E-16,-3.60315789384389E-15));
#41998=DIRECTION('',(5.00596043934463E-16,1.,1.25987290672037E-15));
#41999=DIRECTION('center_axis',(1.,-5.00596043934458E-16,-3.60315789384389E-15));
#42000=DIRECTION('ref_axis',(3.60315789384389E-15,-1.12109502864223E-15,
1.));
#42001=DIRECTION('center_axis',(1.,-5.00596043934458E-16,-3.60315789384389E-15));
#42002=DIRECTION('ref_axis',(3.60315789384389E-15,-1.12109502864223E-15,
1.));
#42003=DIRECTION('',(1.,-5.00596043934458E-16,-3.60315789384389E-15));
#42004=DIRECTION('center_axis',(1.,-5.00596043934458E-16,-3.60315789384389E-15));
#42005=DIRECTION('ref_axis',(3.60315789384389E-15,-1.12109502864223E-15,
1.));
#42006=DIRECTION('center_axis',(-3.60315789384389E-15,9.82317150564085E-16,
-1.));
#42007=DIRECTION('ref_axis',(-1.,5.00596043934458E-16,3.60315789384389E-15));
#42008=DIRECTION('',(-5.00596043934462E-16,-1.,-9.82317150564083E-16));
#42009=DIRECTION('',(1.,-5.00596043934458E-16,-3.60315789384389E-15));
#42010=DIRECTION('',(-5.00596043934462E-16,-1.,-9.82317150564083E-16));
#42011=DIRECTION('',(1.,-5.00596043934458E-16,-3.60315789384389E-15));
#42012=DIRECTION('center_axis',(1.,-5.00596043934458E-16,-3.60315789384389E-15));
#42013=DIRECTION('ref_axis',(5.00596043934464E-16,1.,1.67620654095481E-15));
#42014=DIRECTION('center_axis',(-1.,5.00596043934458E-16,3.60315789384389E-15));
#42015=DIRECTION('ref_axis',(5.00596043934464E-16,1.,1.67620654095481E-15));
#42016=DIRECTION('',(1.,-5.00596043934458E-16,-3.60315789384389E-15));
#42017=DIRECTION('center_axis',(-1.,5.00596043934458E-16,3.60315789384389E-15));
#42018=DIRECTION('ref_axis',(5.00596043934464E-16,1.,1.67620654095481E-15));
#42019=DIRECTION('center_axis',(-5.00596043934462E-16,-1.,-1.12109502864223E-15));
#42020=DIRECTION('ref_axis',(-1.,5.00596043934458E-16,3.60315789384389E-15));
#42021=DIRECTION('',(3.60315789384389E-15,-1.12109502864223E-15,1.));
#42022=DIRECTION('',(1.,-5.00596043934458E-16,-3.60315789384389E-15));
#42023=DIRECTION('',(3.60315789384389E-15,-1.12109502864223E-15,1.));
#42024=DIRECTION('center_axis',(1.,-5.00596043934458E-16,-3.60315789384389E-15));
#42025=DIRECTION('ref_axis',(-3.60315789384389E-15,1.12109502864223E-15,
-1.));
#42026=DIRECTION('center_axis',(-1.,5.00596043934458E-16,3.60315789384389E-15));
#42027=DIRECTION('ref_axis',(-3.60315789384389E-15,1.12109502864223E-15,
-1.));
#42028=DIRECTION('',(1.,-5.00596043934458E-16,-3.60315789384389E-15));
#42029=DIRECTION('center_axis',(-1.,5.00596043934458E-16,3.60315789384389E-15));
#42030=DIRECTION('ref_axis',(-3.60315789384389E-15,1.12109502864223E-15,
-1.));
#42031=DIRECTION('center_axis',(5.00596043934463E-16,1.,1.25987290672037E-15));
#42032=DIRECTION('ref_axis',(1.,-5.00596043934458E-16,-3.60315789384389E-15));
#42033=DIRECTION('',(3.60315789384389E-15,-1.25987290672038E-15,1.));
#42034=DIRECTION('',(1.,-5.00596043934458E-16,-3.60315789384389E-15));
#42035=DIRECTION('',(3.60315789384389E-15,-1.25987290672038E-15,1.));
#42036=DIRECTION('center_axis',(1.,-5.00596043934458E-16,-3.60315789384389E-15));
#42037=DIRECTION('ref_axis',(-3.60315789384389E-15,1.12109502864223E-15,
-1.));
#42038=DIRECTION('center_axis',(1.,-5.00596043934458E-16,-3.60315789384389E-15));
#42039=DIRECTION('ref_axis',(-3.60315789384389E-15,1.12109502864223E-15,
-1.));
#42040=DIRECTION('center_axis',(1.,-5.00596043934458E-16,-3.60315789384389E-15));
#42041=DIRECTION('ref_axis',(-3.60315789384389E-15,1.12109502864223E-15,
-1.));
#42042=DIRECTION('',(1.,-5.00596043934458E-16,-3.60315789384389E-15));
#42043=DIRECTION('center_axis',(3.60315789384389E-15,-1.25987290672038E-15,
1.));
#42044=DIRECTION('ref_axis',(1.,-5.00596043934458E-16,-3.60315789384389E-15));
#42045=DIRECTION('',(-5.00596043934463E-16,-1.,-1.25987290672037E-15));
#42046=DIRECTION('',(-5.00596043934463E-16,-1.,-1.25987290672037E-15));
#42047=DIRECTION('',(1.,-5.00596043934458E-16,-3.60315789384389E-15));
#42048=DIRECTION('center_axis',(1.,-5.00596043934458E-16,-3.60315789384389E-15));
#42049=DIRECTION('ref_axis',(-5.00596043934462E-16,-1.,-1.12109502864223E-15));
#42050=DIRECTION('center_axis',(1.,-5.00596043934458E-16,-3.60315789384389E-15));
#42051=DIRECTION('ref_axis',(-5.00596043934462E-16,-1.,-1.12109502864223E-15));
#42052=DIRECTION('center_axis',(1.,-5.00596043934458E-16,-3.60315789384389E-15));
#42053=DIRECTION('ref_axis',(-5.00596043934462E-16,-1.,-1.12109502864223E-15));
#42054=DIRECTION('center_axis',(3.60315789384389E-15,-1.12109502864223E-15,
1.));
#42055=DIRECTION('ref_axis',(1.,-5.00596043934458E-16,-3.60315789384389E-15));
#42056=DIRECTION('',(5.00596043934462E-16,1.,1.12109502864223E-15));
#42057=DIRECTION('',(1.,-5.00596043934458E-16,-3.60315789384389E-15));
#42058=DIRECTION('',(5.00596043934462E-16,1.,1.12109502864223E-15));
#42059=DIRECTION('center_axis',(1.,-5.00596043934458E-16,-3.60315789384389E-15));
#42060=DIRECTION('ref_axis',(-5.00596043934462E-16,-1.,-1.12109502864223E-15));
#42061=DIRECTION('center_axis',(-1.,5.00596043934458E-16,3.60315789384389E-15));
#42062=DIRECTION('ref_axis',(-5.00596043934462E-16,-1.,-1.12109502864223E-15));
#42063=DIRECTION('',(1.,-5.00596043934458E-16,-3.60315789384389E-15));
#42064=DIRECTION('center_axis',(-1.,5.00596043934458E-16,3.60315789384389E-15));
#42065=DIRECTION('ref_axis',(-5.00596043934462E-16,-1.,-1.12109502864223E-15));
#42066=DIRECTION('center_axis',(5.00596043934464E-16,1.,1.67620654095481E-15));
#42067=DIRECTION('ref_axis',(1.,-5.00596043934458E-16,-3.60315789384389E-15));
#42068=DIRECTION('',(-3.60315789384389E-15,1.67620654095481E-15,-1.));
#42069=DIRECTION('',(1.,-5.00596043934458E-16,-3.60315789384389E-15));
#42070=DIRECTION('',(-3.60315789384389E-15,1.67620654095481E-15,-1.));
#42071=DIRECTION('center_axis',(1.,-5.00596043934458E-16,-3.60315789384389E-15));
#42072=DIRECTION('ref_axis',(3.60315789384389E-15,-1.12109502864223E-15,
1.));
#42073=DIRECTION('center_axis',(-1.,5.00596043934458E-16,3.60315789384389E-15));
#42074=DIRECTION('ref_axis',(3.60315789384389E-15,-1.12109502864223E-15,
1.));
#42075=DIRECTION('center_axis',(-1.,5.00596043934458E-16,3.60315789384389E-15));
#42076=DIRECTION('ref_axis',(3.60315789384389E-15,-1.12109502864223E-15,
1.));
#42077=DIRECTION('center_axis',(1.,-5.00596043934458E-16,-3.60315789384389E-15));
#42078=DIRECTION('ref_axis',(-3.60315789384389E-15,1.12109502864223E-15,
-1.));
#42079=DIRECTION('center_axis',(1.,-5.00596043934458E-16,-3.60315789384389E-15));
#42080=DIRECTION('ref_axis',(-3.60315789384389E-15,1.12109502864223E-15,
-1.));
#42081=DIRECTION('center_axis',(3.25621319864853E-15,-1.12109502864222E-15,
1.));
#42082=DIRECTION('ref_axis',(4.72840468318833E-16,1.,1.12109502864222E-15));
#42083=DIRECTION('',(-1.,4.72840468318829E-16,3.25621319864853E-15));
#42084=DIRECTION('',(-4.72840468318833E-16,-1.,-1.12109502864222E-15));
#42085=DIRECTION('',(-1.,4.72840468318829E-16,3.25621319864853E-15));
#42086=DIRECTION('',(-4.72840468318833E-16,-1.,-1.12109502864222E-15));
#42087=DIRECTION('center_axis',(-4.72840468318833E-16,-1.,-1.12109502864222E-15));
#42088=DIRECTION('ref_axis',(-3.60315789384389E-15,1.12109502864222E-15,
-1.));
#42089=DIRECTION('center_axis',(-4.72840468318833E-16,-1.,-1.12109502864222E-15));
#42090=DIRECTION('ref_axis',(-3.60315789384389E-15,1.12109502864222E-15,
-1.));
#42091=DIRECTION('',(-4.72840468318833E-16,-1.,-1.12109502864222E-15));
#42092=DIRECTION('center_axis',(-4.72840468318833E-16,-1.,-1.12109502864222E-15));
#42093=DIRECTION('ref_axis',(-3.60315789384389E-15,1.12109502864222E-15,
-1.));
#42094=DIRECTION('center_axis',(-1.,4.72840468318829E-16,3.46438001576575E-15));
#42095=DIRECTION('ref_axis',(4.72840468318833E-16,1.,1.12109502864222E-15));
#42096=DIRECTION('',(-3.46438001576574E-15,1.12109502864222E-15,-1.));
#42097=DIRECTION('',(-4.72840468318833E-16,-1.,-1.12109502864222E-15));
#42098=DIRECTION('',(-3.46438001576574E-15,1.12109502864222E-15,-1.));
#42099=DIRECTION('center_axis',(-4.72840468318833E-16,-1.,-1.12109502864222E-15));
#42100=DIRECTION('ref_axis',(1.,-4.72840468318829E-16,-3.60315789384389E-15));
#42101=DIRECTION('center_axis',(-4.72840468318833E-16,-1.,-1.12109502864222E-15));
#42102=DIRECTION('ref_axis',(1.,-4.72840468318829E-16,-3.60315789384389E-15));
#42103=DIRECTION('',(-4.72840468318833E-16,-1.,-1.12109502864222E-15));
#42104=DIRECTION('center_axis',(-4.72840468318833E-16,-1.,-1.12109502864222E-15));
#42105=DIRECTION('ref_axis',(1.,-4.72840468318829E-16,-3.60315789384389E-15));
#42106=DIRECTION('center_axis',(-1.,4.72840468318829E-16,3.74193577192204E-15));
#42107=DIRECTION('ref_axis',(4.72840468318833E-16,1.,1.12109502864222E-15));
#42108=DIRECTION('',(3.74193577192203E-15,-1.12109502864222E-15,1.));
#42109=DIRECTION('',(-4.72840468318833E-16,-1.,-1.12109502864222E-15));
#42110=DIRECTION('',(3.74193577192203E-15,-1.12109502864222E-15,1.));
#42111=DIRECTION('',(-4.72840468318833E-16,-1.,-1.12109502864222E-15));
#42112=DIRECTION('center_axis',(-4.72840468318833E-16,-1.,-1.12109502864222E-15));
#42113=DIRECTION('ref_axis',(-3.04804638153131E-15,1.12109502864222E-15,
-1.));
#42114=DIRECTION('center_axis',(4.72840468318833E-16,1.,1.12109502864222E-15));
#42115=DIRECTION('ref_axis',(-3.04804638153131E-15,1.12109502864222E-15,
-1.));
#42116=DIRECTION('',(-4.72840468318833E-16,-1.,-1.12109502864222E-15));
#42117=DIRECTION('center_axis',(4.72840468318833E-16,1.,1.12109502864222E-15));
#42118=DIRECTION('ref_axis',(-3.04804638153131E-15,1.12109502864222E-15,
-1.));
#42119=DIRECTION('center_axis',(3.60315789384389E-15,-1.12109502864222E-15,
1.));
#42120=DIRECTION('ref_axis',(4.72840468318833E-16,1.,1.12109502864222E-15));
#42121=DIRECTION('',(1.,-4.72840468318829E-16,-3.60315789384389E-15));
#42122=DIRECTION('',(-4.72840468318833E-16,-1.,-1.12109502864222E-15));
#42123=DIRECTION('',(1.,-4.72840468318829E-16,-3.60315789384389E-15));
#42124=DIRECTION('center_axis',(-4.72840468318833E-16,-1.,-1.12109502864222E-15));
#42125=DIRECTION('ref_axis',(-1.,4.72840468318829E-16,3.60315789384389E-15));
#42126=DIRECTION('center_axis',(4.72840468318833E-16,1.,1.12109502864222E-15));
#42127=DIRECTION('ref_axis',(-1.,4.72840468318829E-16,3.60315789384389E-15));
#42128=DIRECTION('',(-4.72840468318833E-16,-1.,-1.12109502864222E-15));
#42129=DIRECTION('center_axis',(4.72840468318833E-16,1.,1.12109502864222E-15));
#42130=DIRECTION('ref_axis',(-1.,4.72840468318829E-16,3.60315789384389E-15));
#42131=DIRECTION('center_axis',(-3.46438001576574E-15,1.12109502864222E-15,
-1.));
#42132=DIRECTION('ref_axis',(-4.72840468318833E-16,-1.,-1.12109502864222E-15));
#42133=DIRECTION('',(1.,-4.72840468318829E-16,-3.46438001576575E-15));
#42134=DIRECTION('',(-4.72840468318833E-16,-1.,-1.12109502864222E-15));
#42135=DIRECTION('',(1.,-4.72840468318829E-16,-3.46438001576575E-15));
#42136=DIRECTION('center_axis',(-4.72840468318833E-16,-1.,-1.12109502864222E-15));
#42137=DIRECTION('ref_axis',(-1.,4.72840468318829E-16,3.60315789384389E-15));
#42138=DIRECTION('center_axis',(-4.72840468318833E-16,-1.,-1.12109502864222E-15));
#42139=DIRECTION('ref_axis',(-1.,4.72840468318829E-16,3.60315789384389E-15));
#42140=DIRECTION('center_axis',(-4.72840468318833E-16,-1.,-1.12109502864222E-15));
#42141=DIRECTION('ref_axis',(-1.,4.72840468318829E-16,3.60315789384389E-15));
#42142=DIRECTION('',(-4.72840468318833E-16,-1.,-1.12109502864222E-15));
#42143=DIRECTION('center_axis',(1.,-4.72840468318829E-16,-3.46438001576575E-15));
#42144=DIRECTION('ref_axis',(-4.72840468318833E-16,-1.,-1.12109502864222E-15));
#42145=DIRECTION('',(3.46438001576574E-15,-1.12109502864222E-15,1.));
#42146=DIRECTION('',(3.46438001576574E-15,-1.12109502864222E-15,1.));
#42147=DIRECTION('',(-4.72840468318833E-16,-1.,-1.12109502864222E-15));
#42148=DIRECTION('center_axis',(-4.72840468318833E-16,-1.,-1.12109502864222E-15));
#42149=DIRECTION('ref_axis',(3.60315789384389E-15,-1.12109502864222E-15,
1.));
#42150=DIRECTION('center_axis',(-4.72840468318833E-16,-1.,-1.12109502864222E-15));
#42151=DIRECTION('ref_axis',(3.60315789384389E-15,-1.12109502864222E-15,
1.));
#42152=DIRECTION('center_axis',(-4.72840468318833E-16,-1.,-1.12109502864222E-15));
#42153=DIRECTION('ref_axis',(3.60315789384389E-15,-1.12109502864222E-15,
1.));
#42154=DIRECTION('center_axis',(1.,-4.72840468318829E-16,-3.60315789384389E-15));
#42155=DIRECTION('ref_axis',(-4.72840468318833E-16,-1.,-1.12109502864222E-15));
#42156=DIRECTION('',(-3.60315789384389E-15,1.12109502864222E-15,-1.));
#42157=DIRECTION('',(-4.72840468318833E-16,-1.,-1.12109502864222E-15));
#42158=DIRECTION('',(-3.60315789384389E-15,1.12109502864222E-15,-1.));
#42159=DIRECTION('center_axis',(-4.72840468318833E-16,-1.,-1.12109502864222E-15));
#42160=DIRECTION('ref_axis',(3.60315789384389E-15,-1.12109502864222E-15,
1.));
#42161=DIRECTION('center_axis',(4.72840468318833E-16,1.,1.12109502864222E-15));
#42162=DIRECTION('ref_axis',(3.60315789384389E-15,-1.12109502864222E-15,
1.));
#42163=DIRECTION('',(-4.72840468318833E-16,-1.,-1.12109502864222E-15));
#42164=DIRECTION('center_axis',(4.72840468318833E-16,1.,1.12109502864222E-15));
#42165=DIRECTION('ref_axis',(3.60315789384389E-15,-1.12109502864222E-15,
1.));
#42166=DIRECTION('center_axis',(-3.04804638153131E-15,1.12109502864222E-15,
-1.));
#42167=DIRECTION('ref_axis',(-4.72840468318833E-16,-1.,-1.12109502864222E-15));
#42168=DIRECTION('',(-1.,4.7284046831883E-16,3.04804638153131E-15));
#42169=DIRECTION('',(-4.72840468318833E-16,-1.,-1.12109502864222E-15));
#42170=DIRECTION('',(-1.,4.7284046831883E-16,3.04804638153131E-15));
#42171=DIRECTION('center_axis',(-4.72840468318833E-16,-1.,-1.12109502864222E-15));
#42172=DIRECTION('ref_axis',(1.,-4.72840468318829E-16,-3.60315789384389E-15));
#42173=DIRECTION('center_axis',(4.72840468318833E-16,1.,1.12109502864222E-15));
#42174=DIRECTION('ref_axis',(1.,-4.72840468318829E-16,-3.60315789384389E-15));
#42175=DIRECTION('center_axis',(4.72840468318833E-16,1.,1.12109502864222E-15));
#42176=DIRECTION('ref_axis',(1.,-4.72840468318829E-16,-3.60315789384389E-15));
#42177=DIRECTION('center_axis',(-4.72840468318833E-16,-1.,-1.12109502864222E-15));
#42178=DIRECTION('ref_axis',(-1.,4.72840468318829E-16,3.60315789384389E-15));
#42179=DIRECTION('center_axis',(-4.72840468318833E-16,-1.,-1.12109502864222E-15));
#42180=DIRECTION('ref_axis',(-1.,4.72840468318829E-16,3.60315789384389E-15));
#42181=DIRECTION('center_axis',(-3.34404360992238E-15,-1.45117688885522E-12,
-1.));
#42182=DIRECTION('ref_axis',(-5.00596043931499E-16,-1.,1.45117688885522E-12));
#42183=DIRECTION('center_axis',(-3.34404360992238E-15,-1.45117688885522E-12,
-1.));
#42184=DIRECTION('ref_axis',(-5.00596043931499E-16,-1.,1.45117688885522E-12));
#42185=DIRECTION('',(-3.34404360992238E-15,-1.45117688885522E-12,-1.));
#42186=DIRECTION('center_axis',(3.34404360992238E-15,1.45117688885522E-12,
1.));
#42187=DIRECTION('ref_axis',(-5.00596043931499E-16,-1.,1.45117688885522E-12));
#42188=DIRECTION('',(-3.34404360992238E-15,-1.45117688885522E-12,-1.));
#42189=DIRECTION('center_axis',(-2.72104209318181E-15,-1.,1.45117688885522E-12));
#42190=DIRECTION('ref_axis',(-1.,2.72104209318666E-15,3.34404360991843E-15));
#42191=DIRECTION('',(-1.,2.72104209318666E-15,3.34404360991843E-15));
#42192=DIRECTION('',(-3.34404360992238E-15,-1.45117688885522E-12,-1.));
#42193=DIRECTION('',(1.,-2.72104209318666E-15,-3.34404360991843E-15));
#42194=DIRECTION('center_axis',(-3.34404360992238E-15,-1.45117688885522E-12,
-1.));
#42195=DIRECTION('ref_axis',(1.,-5.00596043936352E-16,-3.34404360992165E-15));
#42196=DIRECTION('center_axis',(-3.34404360992238E-15,-1.45117688885522E-12,
-1.));
#42197=DIRECTION('ref_axis',(1.,-5.00596043936352E-16,-3.34404360992165E-15));
#42198=DIRECTION('',(-3.34404360992238E-15,-1.45117688885522E-12,-1.));
#42199=DIRECTION('center_axis',(3.34404360992238E-15,1.45117688885522E-12,
1.));
#42200=DIRECTION('ref_axis',(1.,-5.00596043936352E-16,-3.34404360992165E-15));
#42201=DIRECTION('center_axis',(1.,-5.00596043936352E-16,-3.34404360992165E-15));
#42202=DIRECTION('ref_axis',(-5.00596043931499E-16,-1.,1.45117688885522E-12));
#42203=DIRECTION('',(-5.00596043931499E-16,-1.,1.45117688885522E-12));
#42204=DIRECTION('',(-3.34404360992238E-15,-1.45117688885522E-12,-1.));
#42205=DIRECTION('',(5.00596043931499E-16,1.,-1.45117688885522E-12));
#42206=DIRECTION('center_axis',(-3.34404360992238E-15,-1.45117688885522E-12,
-1.));
#42207=DIRECTION('ref_axis',(-1.72629723500711E-14,1.,-1.45117688885522E-12));
#42208=DIRECTION('center_axis',(-3.34404360992238E-15,-1.45117688885522E-12,
-1.));
#42209=DIRECTION('ref_axis',(-1.72629723500711E-14,1.,-1.45117688885522E-12));
#42210=DIRECTION('',(-3.34404360992238E-15,-1.45117688885522E-12,-1.));
#42211=DIRECTION('center_axis',(3.34404360992238E-15,1.45117688885522E-12,
1.));
#42212=DIRECTION('ref_axis',(-1.72629723500711E-14,1.,-1.45117688885522E-12));
#42213=DIRECTION('center_axis',(5.00596043931499E-16,1.,-1.45117688885522E-12));
#42214=DIRECTION('ref_axis',(1.,-5.00596043936352E-16,-3.34404360992165E-15));
#42215=DIRECTION('',(1.,-5.00596043936352E-16,-3.34404360992165E-15));
#42216=DIRECTION('',(-3.34404360992238E-15,-1.45117688885522E-12,-1.));
#42217=DIRECTION('',(-1.,5.00596043936352E-16,3.34404360992165E-15));
#42218=DIRECTION('center_axis',(-3.34404360992238E-15,-1.45117688885522E-12,
-1.));
#42219=DIRECTION('ref_axis',(-1.,5.00596043936352E-16,3.34404360992165E-15));
#42220=DIRECTION('center_axis',(-3.34404360992238E-15,-1.45117688885522E-12,
-1.));
#42221=DIRECTION('ref_axis',(-1.,5.00596043936352E-16,3.34404360992165E-15));
#42222=DIRECTION('',(-3.34404360992238E-15,-1.45117688885522E-12,-1.));
#42223=DIRECTION('center_axis',(3.34404360992238E-15,1.45117688885522E-12,
1.));
#42224=DIRECTION('ref_axis',(-1.,5.00596043936352E-16,3.34404360992165E-15));
#42225=DIRECTION('center_axis',(-1.,5.00596043936352E-16,3.34404360992165E-15));
#42226=DIRECTION('ref_axis',(5.00596043931499E-16,1.,-1.45117688885522E-12));
#42227=DIRECTION('',(5.00596043931499E-16,1.,-1.45117688885522E-12));
#42228=DIRECTION('',(-5.00596043931499E-16,-1.,1.45117688885522E-12));
#42229=DIRECTION('center_axis',(-3.34404360992238E-15,-1.45117688885522E-12,
-1.));
#42230=DIRECTION('ref_axis',(1.,-2.49924255013345E-12,-3.34404360629554E-15));
#42231=DIRECTION('center_axis',(3.34404360992238E-15,1.45117688885522E-12,
1.));
#42232=DIRECTION('ref_axis',(1.,-2.49924255013345E-12,-3.34404360629554E-15));
#42233=DIRECTION('',(-3.34404360992238E-15,-1.45117688885522E-12,-1.));
#42234=DIRECTION('center_axis',(-3.34404360992238E-15,-1.45117688885522E-12,
-1.));
#42235=DIRECTION('ref_axis',(1.,-2.49924255013345E-12,-3.34404360629554E-15));
#42236=DIRECTION('',(-3.34404360992238E-15,-1.45117688885522E-12,-1.));
#42237=DIRECTION('center_axis',(-1.,5.00596043936352E-16,3.34404360992165E-15));
#42238=DIRECTION('ref_axis',(5.00596043931499E-16,1.,-1.45117688885522E-12));
#42239=DIRECTION('',(-5.00596043931499E-16,-1.,1.45117688885522E-12));
#42240=DIRECTION('',(5.00596043931499E-16,1.,-1.45117688885522E-12));
#42241=DIRECTION('',(-3.34404360992238E-15,-1.45117688885522E-12,-1.));
#42242=DIRECTION('center_axis',(-3.34404360992238E-15,-1.45117688885522E-12,
-1.));
#42243=DIRECTION('ref_axis',(9.41969720926E-13,1.,-1.45117688885522E-12));
#42244=DIRECTION('center_axis',(3.34404360992238E-15,1.45117688885522E-12,
1.));
#42245=DIRECTION('ref_axis',(9.41969720926E-13,1.,-1.45117688885522E-12));
#42246=DIRECTION('center_axis',(-3.34404360992238E-15,-1.45117688885522E-12,
-1.));
#42247=DIRECTION('ref_axis',(9.41969720926E-13,1.,-1.45117688885522E-12));
#42248=DIRECTION('',(-3.34404360992238E-15,-1.45117688885522E-12,-1.));
#42249=DIRECTION('center_axis',(-5.00596043931499E-16,-1.,1.45117688885522E-12));
#42250=DIRECTION('ref_axis',(-1.,5.00596043936352E-16,3.34404360992165E-15));
#42251=DIRECTION('',(1.,-5.00596043936352E-16,-3.34404360992165E-15));
#42252=DIRECTION('',(-1.,5.00596043936352E-16,3.34404360992165E-15));
#42253=DIRECTION('',(-3.34404360992238E-15,-1.45117688885522E-12,-1.));
#42254=DIRECTION('center_axis',(-3.34404360992238E-15,-1.45117688885522E-12,
-1.));
#42255=DIRECTION('ref_axis',(-1.,2.35121281351676E-12,3.34404360651035E-15));
#42256=DIRECTION('center_axis',(3.34404360992238E-15,1.45117688885522E-12,
1.));
#42257=DIRECTION('ref_axis',(-1.,2.35121281351676E-12,3.34404360651035E-15));
#42258=DIRECTION('center_axis',(-3.34404360992238E-15,-1.45117688885522E-12,
-1.));
#42259=DIRECTION('ref_axis',(-1.,2.35121281351676E-12,3.34404360651035E-15));
#42260=DIRECTION('',(-3.34404360992238E-15,-1.45117688885522E-12,-1.));
#42261=DIRECTION('center_axis',(1.,-5.00596043936352E-16,-3.34404360992165E-15));
#42262=DIRECTION('ref_axis',(-5.00596043931499E-16,-1.,1.45117688885522E-12));
#42263=DIRECTION('',(5.00596043931499E-16,1.,-1.45117688885522E-12));
#42264=DIRECTION('',(-5.00596043931499E-16,-1.,1.45117688885522E-12));
#42265=DIRECTION('',(-3.34404360992238E-15,-1.45117688885522E-12,-1.));
#42266=DIRECTION('center_axis',(-3.34404360992238E-15,-1.45117688885522E-12,
-1.));
#42267=DIRECTION('ref_axis',(2.15629266646105E-12,-1.,1.45117688885521E-12));
#42268=DIRECTION('center_axis',(3.34404360992238E-15,1.45117688885522E-12,
1.));
#42269=DIRECTION('ref_axis',(2.15629266646105E-12,-1.,1.45117688885521E-12));
#42270=DIRECTION('center_axis',(-3.34404360992238E-15,-1.45117688885522E-12,
-1.));
#42271=DIRECTION('ref_axis',(2.15629266646105E-12,-1.,1.45117688885521E-12));
#42272=DIRECTION('',(-3.34404360992238E-15,-1.45117688885522E-12,-1.));
#42273=DIRECTION('center_axis',(5.00596043931499E-16,1.,-1.45117688885522E-12));
#42274=DIRECTION('ref_axis',(1.,-5.00596043936352E-16,-3.34404360992165E-15));
#42275=DIRECTION('',(-1.,5.00596043936352E-16,3.34404360992165E-15));
#42276=DIRECTION('',(1.,-5.00596043936352E-16,-3.34404360992165E-15));
#42277=DIRECTION('center_axis',(-3.34404360992238E-15,-1.45117688885522E-12,
-1.));
#42278=DIRECTION('ref_axis',(-1.,5.00596043936352E-16,3.34404360992165E-15));
#42279=DIRECTION('center_axis',(-3.34404360992238E-15,-1.45117688885522E-12,
-1.));
#42280=DIRECTION('ref_axis',(-1.,5.00596043936352E-16,3.34404360992165E-15));
#42281=DIRECTION('center_axis',(-3.34404360992238E-15,-1.45117688885522E-12,
-1.));
#42282=DIRECTION('ref_axis',(-5.00596043931499E-16,-1.,1.45117688885522E-12));
#42283=DIRECTION('center_axis',(-3.34404360992238E-15,-1.45117688885522E-12,
-1.));
#42284=DIRECTION('ref_axis',(-5.00596043931499E-16,-1.,1.45117688885522E-12));
#42285=DIRECTION('',(-3.34404360992238E-15,-1.45117688885522E-12,-1.));
#42286=DIRECTION('center_axis',(3.34404360992238E-15,1.45117688885522E-12,
1.));
#42287=DIRECTION('ref_axis',(-5.00596043931499E-16,-1.,1.45117688885522E-12));
#42288=DIRECTION('',(-3.34404360992238E-15,-1.45117688885522E-12,-1.));
#42289=DIRECTION('center_axis',(-2.72104209318181E-15,-1.,1.45117688885522E-12));
#42290=DIRECTION('ref_axis',(-1.,2.72104209318666E-15,3.34404360991843E-15));
#42291=DIRECTION('',(-1.,2.72104209318666E-15,3.34404360991843E-15));
#42292=DIRECTION('',(-3.34404360992238E-15,-1.45117688885522E-12,-1.));
#42293=DIRECTION('',(1.,-2.72104209318666E-15,-3.34404360991843E-15));
#42294=DIRECTION('center_axis',(-3.34404360992238E-15,-1.45117688885522E-12,
-1.));
#42295=DIRECTION('ref_axis',(1.,-5.00596043936352E-16,-3.34404360992165E-15));
#42296=DIRECTION('center_axis',(-3.34404360992238E-15,-1.45117688885522E-12,
-1.));
#42297=DIRECTION('ref_axis',(1.,-5.00596043936352E-16,-3.34404360992165E-15));
#42298=DIRECTION('',(-3.34404360992238E-15,-1.45117688885522E-12,-1.));
#42299=DIRECTION('center_axis',(3.34404360992238E-15,1.45117688885522E-12,
1.));
#42300=DIRECTION('ref_axis',(1.,-5.00596043936352E-16,-3.34404360992165E-15));
#42301=DIRECTION('center_axis',(1.,-5.00596043936352E-16,-3.34404360992165E-15));
#42302=DIRECTION('ref_axis',(-5.00596043931499E-16,-1.,1.45117688885522E-12));
#42303=DIRECTION('',(-5.00596043931499E-16,-1.,1.45117688885522E-12));
#42304=DIRECTION('',(-3.34404360992238E-15,-1.45117688885522E-12,-1.));
#42305=DIRECTION('',(5.00596043931499E-16,1.,-1.45117688885522E-12));
#42306=DIRECTION('center_axis',(-3.34404360992238E-15,-1.45117688885522E-12,
-1.));
#42307=DIRECTION('ref_axis',(-1.72629723500711E-14,1.,-1.45117688885522E-12));
#42308=DIRECTION('center_axis',(-3.34404360992238E-15,-1.45117688885522E-12,
-1.));
#42309=DIRECTION('ref_axis',(-1.72629723500711E-14,1.,-1.45117688885522E-12));
#42310=DIRECTION('',(-3.34404360992238E-15,-1.45117688885522E-12,-1.));
#42311=DIRECTION('center_axis',(3.34404360992238E-15,1.45117688885522E-12,
1.));
#42312=DIRECTION('ref_axis',(-1.72629723500711E-14,1.,-1.45117688885522E-12));
#42313=DIRECTION('center_axis',(5.00596043931499E-16,1.,-1.45117688885522E-12));
#42314=DIRECTION('ref_axis',(1.,-5.00596043936352E-16,-3.34404360992165E-15));
#42315=DIRECTION('',(1.,-5.00596043936352E-16,-3.34404360992165E-15));
#42316=DIRECTION('',(-3.34404360992238E-15,-1.45117688885522E-12,-1.));
#42317=DIRECTION('',(-1.,5.00596043936352E-16,3.34404360992165E-15));
#42318=DIRECTION('center_axis',(-3.34404360992238E-15,-1.45117688885522E-12,
-1.));
#42319=DIRECTION('ref_axis',(-1.,5.00596043936352E-16,3.34404360992165E-15));
#42320=DIRECTION('center_axis',(-3.34404360992238E-15,-1.45117688885522E-12,
-1.));
#42321=DIRECTION('ref_axis',(-1.,5.00596043936352E-16,3.34404360992165E-15));
#42322=DIRECTION('',(-3.34404360992238E-15,-1.45117688885522E-12,-1.));
#42323=DIRECTION('center_axis',(3.34404360992238E-15,1.45117688885522E-12,
1.));
#42324=DIRECTION('ref_axis',(-1.,5.00596043936352E-16,3.34404360992165E-15));
#42325=DIRECTION('center_axis',(-1.,5.00596043936352E-16,3.34404360992165E-15));
#42326=DIRECTION('ref_axis',(5.00596043931499E-16,1.,-1.45117688885522E-12));
#42327=DIRECTION('',(5.00596043931499E-16,1.,-1.45117688885522E-12));
#42328=DIRECTION('',(-5.00596043931499E-16,-1.,1.45117688885522E-12));
#42329=DIRECTION('center_axis',(-3.34404360992238E-15,-1.45117688885522E-12,
-1.));
#42330=DIRECTION('ref_axis',(1.,-2.49924255013345E-12,-3.34404360629554E-15));
#42331=DIRECTION('center_axis',(3.34404360992238E-15,1.45117688885522E-12,
1.));
#42332=DIRECTION('ref_axis',(1.,-2.49924255013345E-12,-3.34404360629554E-15));
#42333=DIRECTION('',(-3.34404360992238E-15,-1.45117688885522E-12,-1.));
#42334=DIRECTION('center_axis',(-3.34404360992238E-15,-1.45117688885522E-12,
-1.));
#42335=DIRECTION('ref_axis',(1.,-2.49924255013345E-12,-3.34404360629554E-15));
#42336=DIRECTION('',(-3.34404360992238E-15,-1.45117688885522E-12,-1.));
#42337=DIRECTION('center_axis',(-1.,5.00596043936352E-16,3.34404360992165E-15));
#42338=DIRECTION('ref_axis',(5.00596043931499E-16,1.,-1.45117688885522E-12));
#42339=DIRECTION('',(-5.00596043931499E-16,-1.,1.45117688885522E-12));
#42340=DIRECTION('',(5.00596043931499E-16,1.,-1.45117688885522E-12));
#42341=DIRECTION('',(-3.34404360992238E-15,-1.45117688885522E-12,-1.));
#42342=DIRECTION('center_axis',(-3.34404360992238E-15,-1.45117688885522E-12,
-1.));
#42343=DIRECTION('ref_axis',(9.41969720926E-13,1.,-1.45117688885522E-12));
#42344=DIRECTION('center_axis',(3.34404360992238E-15,1.45117688885522E-12,
1.));
#42345=DIRECTION('ref_axis',(9.41969720926E-13,1.,-1.45117688885522E-12));
#42346=DIRECTION('center_axis',(-3.34404360992238E-15,-1.45117688885522E-12,
-1.));
#42347=DIRECTION('ref_axis',(9.41969720926E-13,1.,-1.45117688885522E-12));
#42348=DIRECTION('',(-3.34404360992238E-15,-1.45117688885522E-12,-1.));
#42349=DIRECTION('center_axis',(-5.00596043931499E-16,-1.,1.45117688885522E-12));
#42350=DIRECTION('ref_axis',(-1.,5.00596043936352E-16,3.34404360992165E-15));
#42351=DIRECTION('',(1.,-5.00596043936352E-16,-3.34404360992165E-15));
#42352=DIRECTION('',(-1.,5.00596043936352E-16,3.34404360992165E-15));
#42353=DIRECTION('',(-3.34404360992238E-15,-1.45117688885522E-12,-1.));
#42354=DIRECTION('center_axis',(-3.34404360992238E-15,-1.45117688885522E-12,
-1.));
#42355=DIRECTION('ref_axis',(-1.,2.35121281351676E-12,3.34404360651035E-15));
#42356=DIRECTION('center_axis',(3.34404360992238E-15,1.45117688885522E-12,
1.));
#42357=DIRECTION('ref_axis',(-1.,2.35121281351676E-12,3.34404360651035E-15));
#42358=DIRECTION('center_axis',(-3.34404360992238E-15,-1.45117688885522E-12,
-1.));
#42359=DIRECTION('ref_axis',(-1.,2.35121281351676E-12,3.34404360651035E-15));
#42360=DIRECTION('',(-3.34404360992238E-15,-1.45117688885522E-12,-1.));
#42361=DIRECTION('center_axis',(1.,-5.00596043936352E-16,-3.34404360992165E-15));
#42362=DIRECTION('ref_axis',(-5.00596043931499E-16,-1.,1.45117688885522E-12));
#42363=DIRECTION('',(5.00596043931499E-16,1.,-1.45117688885522E-12));
#42364=DIRECTION('',(-5.00596043931499E-16,-1.,1.45117688885522E-12));
#42365=DIRECTION('',(-3.34404360992238E-15,-1.45117688885522E-12,-1.));
#42366=DIRECTION('center_axis',(-3.34404360992238E-15,-1.45117688885522E-12,
-1.));
#42367=DIRECTION('ref_axis',(2.15629266646105E-12,-1.,1.45117688885521E-12));
#42368=DIRECTION('center_axis',(3.34404360992238E-15,1.45117688885522E-12,
1.));
#42369=DIRECTION('ref_axis',(2.15629266646105E-12,-1.,1.45117688885521E-12));
#42370=DIRECTION('center_axis',(-3.34404360992238E-15,-1.45117688885522E-12,
-1.));
#42371=DIRECTION('ref_axis',(2.15629266646105E-12,-1.,1.45117688885521E-12));
#42372=DIRECTION('',(-3.34404360992238E-15,-1.45117688885522E-12,-1.));
#42373=DIRECTION('center_axis',(5.00596043931499E-16,1.,-1.45117688885522E-12));
#42374=DIRECTION('ref_axis',(1.,-5.00596043936352E-16,-3.34404360992165E-15));
#42375=DIRECTION('',(-1.,5.00596043936352E-16,3.34404360992165E-15));
#42376=DIRECTION('',(1.,-5.00596043936352E-16,-3.34404360992165E-15));
#42377=DIRECTION('center_axis',(-3.34404360992238E-15,-1.45117688885522E-12,
-1.));
#42378=DIRECTION('ref_axis',(-1.,5.00596043936352E-16,3.34404360992165E-15));
#42379=DIRECTION('center_axis',(-3.34404360992238E-15,-1.45117688885522E-12,
-1.));
#42380=DIRECTION('ref_axis',(-1.,5.00596043936352E-16,3.34404360992165E-15));
#42381=DIRECTION('center_axis',(-3.34404360992238E-15,-1.45117688885522E-12,
-1.));
#42382=DIRECTION('ref_axis',(-5.00596043931499E-16,-1.,1.45117688885522E-12));
#42383=DIRECTION('center_axis',(-3.34404360992238E-15,-1.45117688885522E-12,
-1.));
#42384=DIRECTION('ref_axis',(-5.00596043931499E-16,-1.,1.45117688885522E-12));
#42385=DIRECTION('',(-3.34404360992238E-15,-1.45117688885522E-12,-1.));
#42386=DIRECTION('center_axis',(3.34404360992238E-15,1.45117688885522E-12,
1.));
#42387=DIRECTION('ref_axis',(-5.00596043931499E-16,-1.,1.45117688885522E-12));
#42388=DIRECTION('',(-3.34404360992238E-15,-1.45117688885522E-12,-1.));
#42389=DIRECTION('center_axis',(-2.72104209318181E-15,-1.,1.45117688885522E-12));
#42390=DIRECTION('ref_axis',(-1.,2.72104209318666E-15,3.34404360991843E-15));
#42391=DIRECTION('',(-1.,2.72104209318666E-15,3.34404360991843E-15));
#42392=DIRECTION('',(-3.34404360992238E-15,-1.45117688885522E-12,-1.));
#42393=DIRECTION('',(1.,-2.72104209318666E-15,-3.34404360991843E-15));
#42394=DIRECTION('center_axis',(-3.34404360992238E-15,-1.45117688885522E-12,
-1.));
#42395=DIRECTION('ref_axis',(1.,-5.00596043936352E-16,-3.34404360992165E-15));
#42396=DIRECTION('center_axis',(-3.34404360992238E-15,-1.45117688885522E-12,
-1.));
#42397=DIRECTION('ref_axis',(1.,-5.00596043936352E-16,-3.34404360992165E-15));
#42398=DIRECTION('',(-3.34404360992238E-15,-1.45117688885522E-12,-1.));
#42399=DIRECTION('center_axis',(3.34404360992238E-15,1.45117688885522E-12,
1.));
#42400=DIRECTION('ref_axis',(1.,-5.00596043936352E-16,-3.34404360992165E-15));
#42401=DIRECTION('center_axis',(1.,-5.00596043936352E-16,-3.34404360992165E-15));
#42402=DIRECTION('ref_axis',(-5.00596043931499E-16,-1.,1.45117688885522E-12));
#42403=DIRECTION('',(-5.00596043931499E-16,-1.,1.45117688885522E-12));
#42404=DIRECTION('',(-3.34404360992238E-15,-1.45117688885522E-12,-1.));
#42405=DIRECTION('',(5.00596043931499E-16,1.,-1.45117688885522E-12));
#42406=DIRECTION('center_axis',(-3.34404360992238E-15,-1.45117688885522E-12,
-1.));
#42407=DIRECTION('ref_axis',(-1.72629723500711E-14,1.,-1.45117688885522E-12));
#42408=DIRECTION('center_axis',(-3.34404360992238E-15,-1.45117688885522E-12,
-1.));
#42409=DIRECTION('ref_axis',(-1.72629723500711E-14,1.,-1.45117688885522E-12));
#42410=DIRECTION('',(-3.34404360992238E-15,-1.45117688885522E-12,-1.));
#42411=DIRECTION('center_axis',(3.34404360992238E-15,1.45117688885522E-12,
1.));
#42412=DIRECTION('ref_axis',(-1.72629723500711E-14,1.,-1.45117688885522E-12));
#42413=DIRECTION('center_axis',(5.00596043931499E-16,1.,-1.45117688885522E-12));
#42414=DIRECTION('ref_axis',(1.,-5.00596043936352E-16,-3.34404360992165E-15));
#42415=DIRECTION('',(1.,-5.00596043936352E-16,-3.34404360992165E-15));
#42416=DIRECTION('',(-3.34404360992238E-15,-1.45117688885522E-12,-1.));
#42417=DIRECTION('',(-1.,5.00596043936352E-16,3.34404360992165E-15));
#42418=DIRECTION('center_axis',(-3.34404360992238E-15,-1.45117688885522E-12,
-1.));
#42419=DIRECTION('ref_axis',(-1.,5.00596043936352E-16,3.34404360992165E-15));
#42420=DIRECTION('center_axis',(-3.34404360992238E-15,-1.45117688885522E-12,
-1.));
#42421=DIRECTION('ref_axis',(-1.,5.00596043936352E-16,3.34404360992165E-15));
#42422=DIRECTION('',(-3.34404360992238E-15,-1.45117688885522E-12,-1.));
#42423=DIRECTION('center_axis',(3.34404360992238E-15,1.45117688885522E-12,
1.));
#42424=DIRECTION('ref_axis',(-1.,5.00596043936352E-16,3.34404360992165E-15));
#42425=DIRECTION('center_axis',(-1.,5.00596043936352E-16,3.34404360992165E-15));
#42426=DIRECTION('ref_axis',(5.00596043931499E-16,1.,-1.45117688885522E-12));
#42427=DIRECTION('',(5.00596043931499E-16,1.,-1.45117688885522E-12));
#42428=DIRECTION('',(-5.00596043931499E-16,-1.,1.45117688885522E-12));
#42429=DIRECTION('center_axis',(-3.34404360992238E-15,-1.45117688885522E-12,
-1.));
#42430=DIRECTION('ref_axis',(1.,-2.49924255013345E-12,-3.34404360629554E-15));
#42431=DIRECTION('center_axis',(3.34404360992238E-15,1.45117688885522E-12,
1.));
#42432=DIRECTION('ref_axis',(1.,-2.49924255013345E-12,-3.34404360629554E-15));
#42433=DIRECTION('',(-3.34404360992238E-15,-1.45117688885522E-12,-1.));
#42434=DIRECTION('center_axis',(-3.34404360992238E-15,-1.45117688885522E-12,
-1.));
#42435=DIRECTION('ref_axis',(1.,-2.49924255013345E-12,-3.34404360629554E-15));
#42436=DIRECTION('',(-3.34404360992238E-15,-1.45117688885522E-12,-1.));
#42437=DIRECTION('center_axis',(-1.,5.00596043936352E-16,3.34404360992165E-15));
#42438=DIRECTION('ref_axis',(5.00596043931499E-16,1.,-1.45117688885522E-12));
#42439=DIRECTION('',(-5.00596043931499E-16,-1.,1.45117688885522E-12));
#42440=DIRECTION('',(5.00596043931499E-16,1.,-1.45117688885522E-12));
#42441=DIRECTION('',(-3.34404360992238E-15,-1.45117688885522E-12,-1.));
#42442=DIRECTION('center_axis',(-3.34404360992238E-15,-1.45117688885522E-12,
-1.));
#42443=DIRECTION('ref_axis',(9.41969720926E-13,1.,-1.45117688885522E-12));
#42444=DIRECTION('center_axis',(3.34404360992238E-15,1.45117688885522E-12,
1.));
#42445=DIRECTION('ref_axis',(9.41969720926E-13,1.,-1.45117688885522E-12));
#42446=DIRECTION('center_axis',(-3.34404360992238E-15,-1.45117688885522E-12,
-1.));
#42447=DIRECTION('ref_axis',(9.41969720926E-13,1.,-1.45117688885522E-12));
#42448=DIRECTION('',(-3.34404360992238E-15,-1.45117688885522E-12,-1.));
#42449=DIRECTION('center_axis',(-5.00596043931499E-16,-1.,1.45117688885522E-12));
#42450=DIRECTION('ref_axis',(-1.,5.00596043936352E-16,3.34404360992165E-15));
#42451=DIRECTION('',(1.,-5.00596043936352E-16,-3.34404360992165E-15));
#42452=DIRECTION('',(-1.,5.00596043936352E-16,3.34404360992165E-15));
#42453=DIRECTION('',(-3.34404360992238E-15,-1.45117688885522E-12,-1.));
#42454=DIRECTION('center_axis',(-3.34404360992238E-15,-1.45117688885522E-12,
-1.));
#42455=DIRECTION('ref_axis',(-1.,2.35121281351676E-12,3.34404360651035E-15));
#42456=DIRECTION('center_axis',(3.34404360992238E-15,1.45117688885522E-12,
1.));
#42457=DIRECTION('ref_axis',(-1.,2.35121281351676E-12,3.34404360651035E-15));
#42458=DIRECTION('center_axis',(-3.34404360992238E-15,-1.45117688885522E-12,
-1.));
#42459=DIRECTION('ref_axis',(-1.,2.35121281351676E-12,3.34404360651035E-15));
#42460=DIRECTION('',(-3.34404360992238E-15,-1.45117688885522E-12,-1.));
#42461=DIRECTION('center_axis',(1.,-5.00596043936352E-16,-3.34404360992165E-15));
#42462=DIRECTION('ref_axis',(-5.00596043931499E-16,-1.,1.45117688885522E-12));
#42463=DIRECTION('',(5.00596043931499E-16,1.,-1.45117688885522E-12));
#42464=DIRECTION('',(-5.00596043931499E-16,-1.,1.45117688885522E-12));
#42465=DIRECTION('',(-3.34404360992238E-15,-1.45117688885522E-12,-1.));
#42466=DIRECTION('center_axis',(-3.34404360992238E-15,-1.45117688885522E-12,
-1.));
#42467=DIRECTION('ref_axis',(2.15629266646105E-12,-1.,1.45117688885521E-12));
#42468=DIRECTION('center_axis',(3.34404360992238E-15,1.45117688885522E-12,
1.));
#42469=DIRECTION('ref_axis',(2.15629266646105E-12,-1.,1.45117688885521E-12));
#42470=DIRECTION('center_axis',(-3.34404360992238E-15,-1.45117688885522E-12,
-1.));
#42471=DIRECTION('ref_axis',(2.15629266646105E-12,-1.,1.45117688885521E-12));
#42472=DIRECTION('',(-3.34404360992238E-15,-1.45117688885522E-12,-1.));
#42473=DIRECTION('center_axis',(5.00596043931499E-16,1.,-1.45117688885522E-12));
#42474=DIRECTION('ref_axis',(1.,-5.00596043936352E-16,-3.34404360992165E-15));
#42475=DIRECTION('',(-1.,5.00596043936352E-16,3.34404360992165E-15));
#42476=DIRECTION('',(1.,-5.00596043936352E-16,-3.34404360992165E-15));
#42477=DIRECTION('center_axis',(-3.34404360992238E-15,-1.45117688885522E-12,
-1.));
#42478=DIRECTION('ref_axis',(-1.,5.00596043936352E-16,3.34404360992165E-15));
#42479=DIRECTION('center_axis',(-3.34404360992238E-15,-1.45117688885522E-12,
-1.));
#42480=DIRECTION('ref_axis',(-1.,5.00596043936352E-16,3.34404360992165E-15));
#42481=DIRECTION('center_axis',(-3.34404360992238E-15,-1.45117688885522E-12,
-1.));
#42482=DIRECTION('ref_axis',(-5.00596043931499E-16,-1.,1.45117688885522E-12));
#42483=DIRECTION('center_axis',(-3.34404360992238E-15,-1.45117688885522E-12,
-1.));
#42484=DIRECTION('ref_axis',(-5.00596043931499E-16,-1.,1.45117688885522E-12));
#42485=DIRECTION('',(-3.34404360992238E-15,-1.45117688885522E-12,-1.));
#42486=DIRECTION('center_axis',(3.34404360992238E-15,1.45117688885522E-12,
1.));
#42487=DIRECTION('ref_axis',(-5.00596043931499E-16,-1.,1.45117688885522E-12));
#42488=DIRECTION('',(-3.34404360992238E-15,-1.45117688885522E-12,-1.));
#42489=DIRECTION('center_axis',(-2.72104209318181E-15,-1.,1.45117688885522E-12));
#42490=DIRECTION('ref_axis',(-1.,2.72104209318666E-15,3.34404360991843E-15));
#42491=DIRECTION('',(-1.,2.72104209318666E-15,3.34404360991843E-15));
#42492=DIRECTION('',(-3.34404360992238E-15,-1.45117688885522E-12,-1.));
#42493=DIRECTION('',(1.,-2.72104209318666E-15,-3.34404360991843E-15));
#42494=DIRECTION('center_axis',(-3.34404360992238E-15,-1.45117688885522E-12,
-1.));
#42495=DIRECTION('ref_axis',(1.,-5.00596043936352E-16,-3.34404360992165E-15));
#42496=DIRECTION('center_axis',(-3.34404360992238E-15,-1.45117688885522E-12,
-1.));
#42497=DIRECTION('ref_axis',(1.,-5.00596043936352E-16,-3.34404360992165E-15));
#42498=DIRECTION('',(-3.34404360992238E-15,-1.45117688885522E-12,-1.));
#42499=DIRECTION('center_axis',(3.34404360992238E-15,1.45117688885522E-12,
1.));
#42500=DIRECTION('ref_axis',(1.,-5.00596043936352E-16,-3.34404360992165E-15));
#42501=DIRECTION('center_axis',(1.,-5.00596043936352E-16,-3.34404360992165E-15));
#42502=DIRECTION('ref_axis',(-5.00596043931499E-16,-1.,1.45117688885522E-12));
#42503=DIRECTION('',(-5.00596043931499E-16,-1.,1.45117688885522E-12));
#42504=DIRECTION('',(-3.34404360992238E-15,-1.45117688885522E-12,-1.));
#42505=DIRECTION('',(5.00596043931499E-16,1.,-1.45117688885522E-12));
#42506=DIRECTION('center_axis',(-3.34404360992238E-15,-1.45117688885522E-12,
-1.));
#42507=DIRECTION('ref_axis',(-1.72629723500711E-14,1.,-1.45117688885522E-12));
#42508=DIRECTION('center_axis',(-3.34404360992238E-15,-1.45117688885522E-12,
-1.));
#42509=DIRECTION('ref_axis',(-1.72629723500711E-14,1.,-1.45117688885522E-12));
#42510=DIRECTION('',(-3.34404360992238E-15,-1.45117688885522E-12,-1.));
#42511=DIRECTION('center_axis',(3.34404360992238E-15,1.45117688885522E-12,
1.));
#42512=DIRECTION('ref_axis',(-1.72629723500711E-14,1.,-1.45117688885522E-12));
#42513=DIRECTION('center_axis',(5.00596043931499E-16,1.,-1.45117688885522E-12));
#42514=DIRECTION('ref_axis',(1.,-5.00596043936352E-16,-3.34404360992165E-15));
#42515=DIRECTION('',(1.,-5.00596043936352E-16,-3.34404360992165E-15));
#42516=DIRECTION('',(-3.34404360992238E-15,-1.45117688885522E-12,-1.));
#42517=DIRECTION('',(-1.,5.00596043936352E-16,3.34404360992165E-15));
#42518=DIRECTION('center_axis',(-3.34404360992238E-15,-1.45117688885522E-12,
-1.));
#42519=DIRECTION('ref_axis',(-1.,5.00596043936352E-16,3.34404360992165E-15));
#42520=DIRECTION('center_axis',(-3.34404360992238E-15,-1.45117688885522E-12,
-1.));
#42521=DIRECTION('ref_axis',(-1.,5.00596043936352E-16,3.34404360992165E-15));
#42522=DIRECTION('',(-3.34404360992238E-15,-1.45117688885522E-12,-1.));
#42523=DIRECTION('center_axis',(3.34404360992238E-15,1.45117688885522E-12,
1.));
#42524=DIRECTION('ref_axis',(-1.,5.00596043936352E-16,3.34404360992165E-15));
#42525=DIRECTION('center_axis',(-1.,5.00596043936352E-16,3.34404360992165E-15));
#42526=DIRECTION('ref_axis',(5.00596043931499E-16,1.,-1.45117688885522E-12));
#42527=DIRECTION('',(5.00596043931499E-16,1.,-1.45117688885522E-12));
#42528=DIRECTION('',(-5.00596043931499E-16,-1.,1.45117688885522E-12));
#42529=DIRECTION('center_axis',(-3.34404360992238E-15,-1.45117688885522E-12,
-1.));
#42530=DIRECTION('ref_axis',(1.,-2.49924255013345E-12,-3.34404360629554E-15));
#42531=DIRECTION('center_axis',(3.34404360992238E-15,1.45117688885522E-12,
1.));
#42532=DIRECTION('ref_axis',(1.,-2.49924255013345E-12,-3.34404360629554E-15));
#42533=DIRECTION('',(-3.34404360992238E-15,-1.45117688885522E-12,-1.));
#42534=DIRECTION('center_axis',(-3.34404360992238E-15,-1.45117688885522E-12,
-1.));
#42535=DIRECTION('ref_axis',(1.,-2.49924255013345E-12,-3.34404360629554E-15));
#42536=DIRECTION('',(-3.34404360992238E-15,-1.45117688885522E-12,-1.));
#42537=DIRECTION('center_axis',(-1.,5.00596043936352E-16,3.34404360992165E-15));
#42538=DIRECTION('ref_axis',(5.00596043931499E-16,1.,-1.45117688885522E-12));
#42539=DIRECTION('',(-5.00596043931499E-16,-1.,1.45117688885522E-12));
#42540=DIRECTION('',(5.00596043931499E-16,1.,-1.45117688885522E-12));
#42541=DIRECTION('',(-3.34404360992238E-15,-1.45117688885522E-12,-1.));
#42542=DIRECTION('center_axis',(-3.34404360992238E-15,-1.45117688885522E-12,
-1.));
#42543=DIRECTION('ref_axis',(9.41969720926E-13,1.,-1.45117688885522E-12));
#42544=DIRECTION('center_axis',(3.34404360992238E-15,1.45117688885522E-12,
1.));
#42545=DIRECTION('ref_axis',(9.41969720926E-13,1.,-1.45117688885522E-12));
#42546=DIRECTION('center_axis',(-3.34404360992238E-15,-1.45117688885522E-12,
-1.));
#42547=DIRECTION('ref_axis',(9.41969720926E-13,1.,-1.45117688885522E-12));
#42548=DIRECTION('',(-3.34404360992238E-15,-1.45117688885522E-12,-1.));
#42549=DIRECTION('center_axis',(-5.00596043931499E-16,-1.,1.45117688885522E-12));
#42550=DIRECTION('ref_axis',(-1.,5.00596043936352E-16,3.34404360992165E-15));
#42551=DIRECTION('',(1.,-5.00596043936352E-16,-3.34404360992165E-15));
#42552=DIRECTION('',(-1.,5.00596043936352E-16,3.34404360992165E-15));
#42553=DIRECTION('',(-3.34404360992238E-15,-1.45117688885522E-12,-1.));
#42554=DIRECTION('center_axis',(-3.34404360992238E-15,-1.45117688885522E-12,
-1.));
#42555=DIRECTION('ref_axis',(-1.,2.35121281351676E-12,3.34404360651035E-15));
#42556=DIRECTION('center_axis',(3.34404360992238E-15,1.45117688885522E-12,
1.));
#42557=DIRECTION('ref_axis',(-1.,2.35121281351676E-12,3.34404360651035E-15));
#42558=DIRECTION('center_axis',(-3.34404360992238E-15,-1.45117688885522E-12,
-1.));
#42559=DIRECTION('ref_axis',(-1.,2.35121281351676E-12,3.34404360651035E-15));
#42560=DIRECTION('',(-3.34404360992238E-15,-1.45117688885522E-12,-1.));
#42561=DIRECTION('center_axis',(1.,-5.00596043936352E-16,-3.34404360992165E-15));
#42562=DIRECTION('ref_axis',(-5.00596043931499E-16,-1.,1.45117688885522E-12));
#42563=DIRECTION('',(5.00596043931499E-16,1.,-1.45117688885522E-12));
#42564=DIRECTION('',(-5.00596043931499E-16,-1.,1.45117688885522E-12));
#42565=DIRECTION('',(-3.34404360992238E-15,-1.45117688885522E-12,-1.));
#42566=DIRECTION('center_axis',(-3.34404360992238E-15,-1.45117688885522E-12,
-1.));
#42567=DIRECTION('ref_axis',(2.15629266646105E-12,-1.,1.45117688885521E-12));
#42568=DIRECTION('center_axis',(3.34404360992238E-15,1.45117688885522E-12,
1.));
#42569=DIRECTION('ref_axis',(2.15629266646105E-12,-1.,1.45117688885521E-12));
#42570=DIRECTION('center_axis',(-3.34404360992238E-15,-1.45117688885522E-12,
-1.));
#42571=DIRECTION('ref_axis',(2.15629266646105E-12,-1.,1.45117688885521E-12));
#42572=DIRECTION('',(-3.34404360992238E-15,-1.45117688885522E-12,-1.));
#42573=DIRECTION('center_axis',(5.00596043931499E-16,1.,-1.45117688885522E-12));
#42574=DIRECTION('ref_axis',(1.,-5.00596043936352E-16,-3.34404360992165E-15));
#42575=DIRECTION('',(-1.,5.00596043936352E-16,3.34404360992165E-15));
#42576=DIRECTION('',(1.,-5.00596043936352E-16,-3.34404360992165E-15));
#42577=DIRECTION('center_axis',(-3.34404360992238E-15,-1.45117688885522E-12,
-1.));
#42578=DIRECTION('ref_axis',(-1.,5.00596043936352E-16,3.34404360992165E-15));
#42579=DIRECTION('center_axis',(-3.34404360992238E-15,-1.45117688885522E-12,
-1.));
#42580=DIRECTION('ref_axis',(-1.,5.00596043936352E-16,3.34404360992165E-15));
#53781=CARTESIAN_POINT('',(0.,0.,0.));
#53782=CARTESIAN_POINT('Origin',(489.615917770968,-307.972007269816,-379.220287241398));
#53783=CARTESIAN_POINT('',(457.61591777097,-307.972007268858,280.779712758602));
#53784=CARTESIAN_POINT('',(489.61591777097,-307.972007268858,280.779712758602));
#53785=CARTESIAN_POINT('',(481.61591777097,-307.972007268858,280.779712758602));
#53786=CARTESIAN_POINT('',(489.615917770968,-307.972007269816,-379.220287241398));
#53787=CARTESIAN_POINT('',(489.615917770968,-307.972007269816,-379.220287241398));
#53788=CARTESIAN_POINT('',(457.615917770968,-307.972007269816,-379.220287241398));
#53789=CARTESIAN_POINT('',(481.615917770968,-307.972007269816,-379.220287241398));
#53790=CARTESIAN_POINT('',(457.615917770968,-307.972007269816,-379.220287241398));
#53791=CARTESIAN_POINT('Origin',(489.615917770968,-305.972007269816,-379.220287241401));
#53792=CARTESIAN_POINT('',(491.61591777097,-305.972007268858,280.779712758599));
#53793=CARTESIAN_POINT('Origin',(489.61591777097,-305.972007268858,280.779712758599));
#53794=CARTESIAN_POINT('',(491.615917770968,-305.972007269816,-379.220287241401));
#53795=CARTESIAN_POINT('',(491.615917770968,-305.972007269816,-379.220287241401));
#53796=CARTESIAN_POINT('Origin',(489.615917770968,-305.972007269816,-379.220287241401));
#53797=CARTESIAN_POINT('Origin',(491.615917770968,-273.972007269816,-379.220287241447));
#53798=CARTESIAN_POINT('',(491.61591777097,-273.972007268858,280.779712758553));
#53799=CARTESIAN_POINT('',(491.61591777097,-281.972007268858,280.779712758564));
#53800=CARTESIAN_POINT('',(491.615917770968,-273.972007269816,-379.220287241447));
#53801=CARTESIAN_POINT('',(491.615917770968,-273.972007269816,-379.220287241447));
#53802=CARTESIAN_POINT('',(491.615917770968,-281.972007269816,-379.220287241436));
#53803=CARTESIAN_POINT('Origin',(489.615917770968,-273.972007269816,-379.220287241447));
#53804=CARTESIAN_POINT('',(489.61591777097,-271.972007268858,280.77971275855));
#53805=CARTESIAN_POINT('Origin',(489.61591777097,-273.972007268858,280.779712758553));
#53806=CARTESIAN_POINT('',(489.615917770968,-271.972007269816,-379.22028724145));
#53807=CARTESIAN_POINT('',(489.615917770968,-271.972007269816,-379.22028724145));
#53808=CARTESIAN_POINT('Origin',(489.615917770968,-273.972007269816,-379.220287241447));
#53809=CARTESIAN_POINT('Origin',(493.615917770968,-273.972007269816,-379.220287241447));
#53810=CARTESIAN_POINT('',(493.61591777097,-273.972007268858,280.779712758553));
#53811=CARTESIAN_POINT('',(493.61591777097,-305.972007268858,280.779712758599));
#53812=CARTESIAN_POINT('',(493.61591777097,-281.972007268858,280.779712758564));
#53813=CARTESIAN_POINT('',(493.615917770968,-305.972007269816,-379.220287241401));
#53814=CARTESIAN_POINT('',(493.615917770968,-305.972007269816,-379.220287241401));
#53815=CARTESIAN_POINT('',(493.615917770968,-273.972007269816,-379.220287241447));
#53816=CARTESIAN_POINT('',(493.615917770968,-281.972007269816,-379.220287241436));
#53817=CARTESIAN_POINT('',(493.615917770968,-273.972007269816,-379.220287241447));
#53818=CARTESIAN_POINT('Origin',(489.615917770968,-305.972007269816,-379.220287241401));
#53819=CARTESIAN_POINT('',(489.61591777097,-309.972007268858,280.779712758605));
#53820=CARTESIAN_POINT('Origin',(489.61591777097,-305.972007268858,280.779712758599));
#53821=CARTESIAN_POINT('',(489.615917770968,-309.972007269816,-379.220287241395));
#53822=CARTESIAN_POINT('',(489.615917770968,-309.972007269816,-379.220287241395));
#53823=CARTESIAN_POINT('Origin',(489.615917770968,-305.972007269816,-379.220287241401));
#53824=CARTESIAN_POINT('Origin',(489.615917770968,-309.972007269816,-379.220287241395));
#53825=CARTESIAN_POINT('',(457.61591777097,-309.972007268858,280.779712758605));
#53826=CARTESIAN_POINT('',(481.61591777097,-309.972007268858,280.779712758605));
#53827=CARTESIAN_POINT('',(457.615917770968,-309.972007269816,-379.220287241395));
#53828=CARTESIAN_POINT('',(457.615917770968,-309.972007269816,-379.220287241395));
#53829=CARTESIAN_POINT('',(481.615917770968,-309.972007269816,-379.220287241395));
#53830=CARTESIAN_POINT('Origin',(457.615917770968,-305.972007269816,-379.220287241401));
#53831=CARTESIAN_POINT('',(453.61591777097,-305.972007268858,280.779712758599));
#53832=CARTESIAN_POINT('Origin',(457.61591777097,-305.972007268858,280.779712758599));
#53833=CARTESIAN_POINT('',(453.615917770968,-305.972007269816,-379.220287241401));
#53834=CARTESIAN_POINT('',(453.615917770968,-305.972007269816,-379.220287241401));
#53835=CARTESIAN_POINT('Origin',(457.615917770968,-305.972007269816,-379.220287241401));
#53836=CARTESIAN_POINT('Origin',(457.615917770968,-271.972007269816,-379.22028724145));
#53837=CARTESIAN_POINT('',(457.61591777097,-271.972007268858,280.77971275855));
#53838=CARTESIAN_POINT('',(465.61591777097,-271.972007268858,280.77971275855));
#53839=CARTESIAN_POINT('',(457.615917770968,-271.972007269816,-379.22028724145));
#53840=CARTESIAN_POINT('',(457.615917770968,-271.972007269816,-379.22028724145));
#53841=CARTESIAN_POINT('',(465.615917770968,-271.972007269816,-379.22028724145));
#53842=CARTESIAN_POINT('Origin',(457.615917770968,-305.972007269816,-379.220287241401));
#53843=CARTESIAN_POINT('',(455.61591777097,-305.972007268858,280.779712758599));
#53844=CARTESIAN_POINT('Origin',(457.61591777097,-305.972007268858,280.779712758599));
#53845=CARTESIAN_POINT('',(455.615917770968,-305.972007269816,-379.220287241401));
#53846=CARTESIAN_POINT('Origin',(457.615917770968,-305.972007269816,-379.220287241401));
#53847=CARTESIAN_POINT('',(455.615917770968,-305.972007269816,-379.220287241401));
#53848=CARTESIAN_POINT('Origin',(455.615917770968,-305.972007269816,-379.220287241401));
#53849=CARTESIAN_POINT('',(455.61591777097,-273.972007268858,280.779712758553));
#53850=CARTESIAN_POINT('',(455.61591777097,-297.972007268858,280.779712758588));
#53851=CARTESIAN_POINT('',(455.615917770968,-273.972007269816,-379.220287241447));
#53852=CARTESIAN_POINT('',(455.615917770968,-297.972007269816,-379.220287241412));
#53853=CARTESIAN_POINT('',(455.615917770968,-273.972007269816,-379.220287241447));
#53854=CARTESIAN_POINT('Origin',(457.615917770968,-273.972007269816,-379.220287241447));
#53855=CARTESIAN_POINT('Origin',(457.61591777097,-273.972007268858,280.779712758553));
#53856=CARTESIAN_POINT('Origin',(457.615917770968,-273.972007269816,-379.220287241447));
#53857=CARTESIAN_POINT('Origin',(453.615917770968,-305.972007269816,-379.220287241401));
#53858=CARTESIAN_POINT('',(453.61591777097,-273.972007268858,280.779712758553));
#53859=CARTESIAN_POINT('',(453.61591777097,-297.972007268858,280.779712758588));
#53860=CARTESIAN_POINT('',(453.615917770968,-273.972007269816,-379.220287241447));
#53861=CARTESIAN_POINT('',(453.615917770968,-273.972007269816,-379.220287241447));
#53862=CARTESIAN_POINT('',(453.615917770968,-297.972007269816,-379.220287241412));
#53863=CARTESIAN_POINT('Origin',(457.615917770968,-273.972007269816,-379.220287241447));
#53864=CARTESIAN_POINT('',(457.61591777097,-269.972007268858,280.779712758547));
#53865=CARTESIAN_POINT('Origin',(457.61591777097,-273.972007268858,280.779712758553));
#53866=CARTESIAN_POINT('',(457.615917770968,-269.972007269816,-379.220287241453));
#53867=CARTESIAN_POINT('',(457.615917770968,-269.972007269816,-379.220287241453));
#53868=CARTESIAN_POINT('Origin',(457.615917770968,-273.972007269816,-379.220287241447));
#53869=CARTESIAN_POINT('Origin',(457.615917770968,-269.972007269816,-379.220287241453));
#53870=CARTESIAN_POINT('',(489.61591777097,-269.972007268858,280.779712758547));
#53871=CARTESIAN_POINT('',(465.61591777097,-269.972007268858,280.779712758547));
#53872=CARTESIAN_POINT('',(489.615917770968,-269.972007269816,-379.220287241453));
#53873=CARTESIAN_POINT('',(489.615917770968,-269.972007269816,-379.220287241453));
#53874=CARTESIAN_POINT('',(465.615917770968,-269.972007269816,-379.220287241453));
#53875=CARTESIAN_POINT('Origin',(489.615917770968,-273.972007269816,-379.220287241447));
#53876=CARTESIAN_POINT('Origin',(489.61591777097,-273.972007268858,280.779712758553));
#53877=CARTESIAN_POINT('Origin',(489.615917770968,-273.972007269816,-379.220287241447));
#53878=CARTESIAN_POINT('Origin',(473.615917770968,-289.972007269816,-379.220287241424));
#53879=CARTESIAN_POINT('Origin',(473.61591777097,-289.972007268858,280.779712758576));
#53880=CARTESIAN_POINT('Origin',(489.615917770968,292.027992730186,-379.220287242269));
#53881=CARTESIAN_POINT('',(457.61591777097,292.027992731145,281.279712757731));
#53882=CARTESIAN_POINT('',(489.61591777097,292.027992731144,281.279712757731));
#53883=CARTESIAN_POINT('',(481.61591777097,292.027992731145,281.279712757731));
#53884=CARTESIAN_POINT('',(489.615917770968,292.027992730186,-379.220287242269));
#53885=CARTESIAN_POINT('',(489.615917770968,292.027992730186,-379.220287242269));
#53886=CARTESIAN_POINT('',(457.615917770968,292.027992730186,-379.220287242269));
#53887=CARTESIAN_POINT('',(481.615917770968,292.027992730186,-379.220287242269));
#53888=CARTESIAN_POINT('',(457.615917770968,292.027992730186,-379.220287242269));
#53889=CARTESIAN_POINT('Origin',(489.615917770968,294.027992730186,-379.220287242272));
#53890=CARTESIAN_POINT('',(491.61591777097,294.027992731144,281.279712757728));
#53891=CARTESIAN_POINT('Origin',(489.61591777097,294.027992731144,281.279712757728));
#53892=CARTESIAN_POINT('',(491.615917770968,294.027992730186,-379.220287242272));
#53893=CARTESIAN_POINT('',(491.615917770968,294.027992730186,-379.220287242272));
#53894=CARTESIAN_POINT('Origin',(489.615917770968,294.027992730186,-379.220287242272));
#53895=CARTESIAN_POINT('Origin',(491.615917770968,326.027992730186,-379.220287242318));
#53896=CARTESIAN_POINT('',(491.61591777097,326.027992731144,281.279712757682));
#53897=CARTESIAN_POINT('',(491.61591777097,318.027992731144,281.279712757693));
#53898=CARTESIAN_POINT('',(491.615917770968,326.027992730186,-379.220287242318));
#53899=CARTESIAN_POINT('',(491.615917770968,326.027992730186,-379.220287242318));
#53900=CARTESIAN_POINT('',(491.615917770968,318.027992730186,-379.220287242307));
#53901=CARTESIAN_POINT('Origin',(489.615917770968,326.027992730186,-379.220287242318));
#53902=CARTESIAN_POINT('',(489.61591777097,328.027992731144,281.279712757679));
#53903=CARTESIAN_POINT('Origin',(489.61591777097,326.027992731144,281.279712757682));
#53904=CARTESIAN_POINT('',(489.615917770968,328.027992730186,-379.220287242321));
#53905=CARTESIAN_POINT('',(489.615917770968,328.027992730186,-379.220287242321));
#53906=CARTESIAN_POINT('Origin',(489.615917770968,326.027992730186,-379.220287242318));
#53907=CARTESIAN_POINT('Origin',(493.615917770968,326.027992730186,-379.220287242318));
#53908=CARTESIAN_POINT('',(493.61591777097,326.027992731144,281.279712757682));
#53909=CARTESIAN_POINT('',(493.61591777097,294.027992731144,281.279712757728));
#53910=CARTESIAN_POINT('',(493.61591777097,318.027992731144,281.279712757693));
#53911=CARTESIAN_POINT('',(493.615917770968,294.027992730186,-379.220287242272));
#53912=CARTESIAN_POINT('',(493.615917770968,294.027992730186,-379.220287242272));
#53913=CARTESIAN_POINT('',(493.615917770968,326.027992730186,-379.220287242318));
#53914=CARTESIAN_POINT('',(493.615917770968,318.027992730186,-379.220287242307));
#53915=CARTESIAN_POINT('',(493.615917770968,326.027992730186,-379.220287242318));
#53916=CARTESIAN_POINT('Origin',(489.615917770968,294.027992730186,-379.220287242272));
#53917=CARTESIAN_POINT('',(489.61591777097,290.027992731144,281.279712757734));
#53918=CARTESIAN_POINT('Origin',(489.61591777097,294.027992731144,281.279712757728));
#53919=CARTESIAN_POINT('',(489.615917770968,290.027992730186,-379.220287242266));
#53920=CARTESIAN_POINT('',(489.615917770968,290.027992730186,-379.220287242266));
#53921=CARTESIAN_POINT('Origin',(489.615917770968,294.027992730186,-379.220287242272));
#53922=CARTESIAN_POINT('Origin',(489.615917770968,290.027992730186,-379.220287242266));
#53923=CARTESIAN_POINT('',(457.61591777097,290.027992731145,281.279712757734));
#53924=CARTESIAN_POINT('',(481.61591777097,290.027992731144,281.279712757734));
#53925=CARTESIAN_POINT('',(457.615917770968,290.027992730186,-379.220287242266));
#53926=CARTESIAN_POINT('',(457.615917770968,290.027992730186,-379.220287242266));
#53927=CARTESIAN_POINT('',(481.615917770968,290.027992730186,-379.220287242266));
#53928=CARTESIAN_POINT('Origin',(457.615917770968,294.027992730186,-379.220287242272));
#53929=CARTESIAN_POINT('',(453.61591777097,294.027992731144,281.279712757728));
#53930=CARTESIAN_POINT('Origin',(457.61591777097,294.027992731144,281.279712757728));
#53931=CARTESIAN_POINT('',(453.615917770968,294.027992730186,-379.220287242272));
#53932=CARTESIAN_POINT('',(453.615917770968,294.027992730186,-379.220287242272));
#53933=CARTESIAN_POINT('Origin',(457.615917770968,294.027992730186,-379.220287242272));
#53934=CARTESIAN_POINT('Origin',(457.615917770968,328.027992730186,-379.220287242321));
#53935=CARTESIAN_POINT('',(457.61591777097,328.027992731145,281.279712757679));
#53936=CARTESIAN_POINT('',(465.61591777097,328.027992731145,281.279712757679));
#53937=CARTESIAN_POINT('',(457.615917770968,328.027992730186,-379.220287242321));
#53938=CARTESIAN_POINT('',(457.615917770968,328.027992730186,-379.220287242321));
#53939=CARTESIAN_POINT('',(465.615917770968,328.027992730186,-379.220287242321));
#53940=CARTESIAN_POINT('Origin',(457.615917770968,294.027992730186,-379.220287242272));
#53941=CARTESIAN_POINT('',(455.61591777097,294.027992731144,281.279712757728));
#53942=CARTESIAN_POINT('Origin',(457.61591777097,294.027992731144,281.279712757728));
#53943=CARTESIAN_POINT('',(455.615917770968,294.027992730186,-379.220287242272));
#53944=CARTESIAN_POINT('Origin',(457.615917770968,294.027992730186,-379.220287242272));
#53945=CARTESIAN_POINT('',(455.615917770968,294.027992730186,-379.220287242272));
#53946=CARTESIAN_POINT('Origin',(455.615917770968,294.027992730186,-379.220287242272));
#53947=CARTESIAN_POINT('',(455.61591777097,326.027992731144,281.279712757682));
#53948=CARTESIAN_POINT('',(455.61591777097,302.027992731145,281.279712757717));
#53949=CARTESIAN_POINT('',(455.615917770968,326.027992730186,-379.220287242318));
#53950=CARTESIAN_POINT('',(455.615917770968,302.027992730186,-379.220287242283));
#53951=CARTESIAN_POINT('',(455.615917770968,326.027992730186,-379.220287242318));
#53952=CARTESIAN_POINT('Origin',(457.615917770968,326.027992730186,-379.220287242318));
#53953=CARTESIAN_POINT('Origin',(457.61591777097,326.027992731144,281.279712757682));
#53954=CARTESIAN_POINT('Origin',(457.615917770968,326.027992730186,-379.220287242318));
#53955=CARTESIAN_POINT('Origin',(453.615917770968,294.027992730186,-379.220287242272));
#53956=CARTESIAN_POINT('',(453.61591777097,326.027992731144,281.279712757682));
#53957=CARTESIAN_POINT('',(453.61591777097,302.027992731145,281.279712757717));
#53958=CARTESIAN_POINT('',(453.615917770968,326.027992730186,-379.220287242318));
#53959=CARTESIAN_POINT('',(453.615917770968,326.027992730186,-379.220287242318));
#53960=CARTESIAN_POINT('',(453.615917770968,302.027992730186,-379.220287242283));
#53961=CARTESIAN_POINT('Origin',(457.615917770968,326.027992730186,-379.220287242318));
#53962=CARTESIAN_POINT('',(457.61591777097,330.027992731144,281.279712757676));
#53963=CARTESIAN_POINT('Origin',(457.61591777097,326.027992731144,281.279712757682));
#53964=CARTESIAN_POINT('',(457.615917770968,330.027992730186,-379.220287242324));
#53965=CARTESIAN_POINT('',(457.615917770968,330.027992730186,-379.220287242324));
#53966=CARTESIAN_POINT('Origin',(457.615917770968,326.027992730186,-379.220287242318));
#53967=CARTESIAN_POINT('Origin',(457.615917770968,330.027992730186,-379.220287242324));
#53968=CARTESIAN_POINT('',(489.61591777097,330.027992731144,281.279712757676));
#53969=CARTESIAN_POINT('',(465.61591777097,330.027992731144,281.279712757676));
#53970=CARTESIAN_POINT('',(489.615917770968,330.027992730186,-379.220287242324));
#53971=CARTESIAN_POINT('',(489.615917770968,330.027992730186,-379.220287242324));
#53972=CARTESIAN_POINT('',(465.615917770968,330.027992730186,-379.220287242324));
#53973=CARTESIAN_POINT('Origin',(489.615917770968,326.027992730186,-379.220287242318));
#53974=CARTESIAN_POINT('Origin',(489.61591777097,326.027992731144,281.279712757682));
#53975=CARTESIAN_POINT('Origin',(489.615917770968,326.027992730186,-379.220287242318));
#53976=CARTESIAN_POINT('Origin',(473.615917770968,310.027992730186,-379.220287242295));
#53977=CARTESIAN_POINT('Origin',(473.61591777097,310.027992731145,281.279712757705));
#53978=CARTESIAN_POINT('Origin',(180.115917770962,292.027992730186,-379.220287242268));
#53979=CARTESIAN_POINT('',(148.115917770964,292.027992731145,281.279712757732));
#53980=CARTESIAN_POINT('',(180.115917770964,292.027992731144,281.279712757732));
#53981=CARTESIAN_POINT('',(172.115917770964,292.027992731145,281.279712757732));
#53982=CARTESIAN_POINT('',(180.115917770962,292.027992730186,-379.220287242268));
#53983=CARTESIAN_POINT('',(180.115917770962,292.027992730186,-379.220287242268));
#53984=CARTESIAN_POINT('',(148.115917770962,292.027992730186,-379.220287242268));
#53985=CARTESIAN_POINT('',(172.115917770962,292.027992730186,-379.220287242268));
#53986=CARTESIAN_POINT('',(148.115917770962,292.027992730186,-379.220287242268));
#53987=CARTESIAN_POINT('Origin',(180.115917770962,294.027992730186,-379.220287242271));
#53988=CARTESIAN_POINT('',(182.115917770964,294.027992731144,281.279712757729));
#53989=CARTESIAN_POINT('Origin',(180.115917770964,294.027992731144,281.279712757729));
#53990=CARTESIAN_POINT('',(182.115917770962,294.027992730186,-379.220287242271));
#53991=CARTESIAN_POINT('',(182.115917770962,294.027992730186,-379.220287242271));
#53992=CARTESIAN_POINT('Origin',(180.115917770962,294.027992730186,-379.220287242271));
#53993=CARTESIAN_POINT('Origin',(182.115917770962,326.027992730186,-379.220287242317));
#53994=CARTESIAN_POINT('',(182.115917770964,326.027992731144,281.279712757683));
#53995=CARTESIAN_POINT('',(182.115917770964,318.027992731144,281.279712757694));
#53996=CARTESIAN_POINT('',(182.115917770962,326.027992730186,-379.220287242317));
#53997=CARTESIAN_POINT('',(182.115917770962,326.027992730186,-379.220287242317));
#53998=CARTESIAN_POINT('',(182.115917770962,318.027992730186,-379.220287242306));
#53999=CARTESIAN_POINT('Origin',(180.115917770962,326.027992730186,-379.220287242317));
#54000=CARTESIAN_POINT('',(180.115917770964,328.027992731144,281.27971275768));
#54001=CARTESIAN_POINT('Origin',(180.115917770964,326.027992731144,281.279712757683));
#54002=CARTESIAN_POINT('',(180.115917770962,328.027992730186,-379.22028724232));
#54003=CARTESIAN_POINT('',(180.115917770962,328.027992730186,-379.22028724232));
#54004=CARTESIAN_POINT('Origin',(180.115917770962,326.027992730186,-379.220287242317));
#54005=CARTESIAN_POINT('Origin',(184.115917770962,326.027992730186,-379.220287242317));
#54006=CARTESIAN_POINT('',(184.115917770964,326.027992731144,281.279712757683));
#54007=CARTESIAN_POINT('',(184.115917770964,294.027992731144,281.279712757729));
#54008=CARTESIAN_POINT('',(184.115917770964,318.027992731144,281.279712757694));
#54009=CARTESIAN_POINT('',(184.115917770962,294.027992730186,-379.220287242271));
#54010=CARTESIAN_POINT('',(184.115917770962,294.027992730186,-379.220287242271));
#54011=CARTESIAN_POINT('',(184.115917770962,326.027992730186,-379.220287242317));
#54012=CARTESIAN_POINT('',(184.115917770962,318.027992730186,-379.220287242306));
#54013=CARTESIAN_POINT('',(184.115917770962,326.027992730186,-379.220287242317));
#54014=CARTESIAN_POINT('Origin',(180.115917770962,294.027992730186,-379.220287242271));
#54015=CARTESIAN_POINT('',(180.115917770964,290.027992731144,281.279712757735));
#54016=CARTESIAN_POINT('Origin',(180.115917770964,294.027992731144,281.279712757729));
#54017=CARTESIAN_POINT('',(180.115917770962,290.027992730186,-379.220287242265));
#54018=CARTESIAN_POINT('',(180.115917770962,290.027992730186,-379.220287242265));
#54019=CARTESIAN_POINT('Origin',(180.115917770962,294.027992730186,-379.220287242271));
#54020=CARTESIAN_POINT('Origin',(180.115917770962,290.027992730186,-379.220287242265));
#54021=CARTESIAN_POINT('',(148.115917770964,290.027992731145,281.279712757735));
#54022=CARTESIAN_POINT('',(172.115917770964,290.027992731144,281.279712757735));
#54023=CARTESIAN_POINT('',(148.115917770962,290.027992730186,-379.220287242265));
#54024=CARTESIAN_POINT('',(148.115917770962,290.027992730186,-379.220287242265));
#54025=CARTESIAN_POINT('',(172.115917770962,290.027992730186,-379.220287242265));
#54026=CARTESIAN_POINT('Origin',(148.115917770962,294.027992730186,-379.220287242271));
#54027=CARTESIAN_POINT('',(144.115917770964,294.027992731144,281.279712757729));
#54028=CARTESIAN_POINT('Origin',(148.115917770964,294.027992731144,281.279712757729));
#54029=CARTESIAN_POINT('',(144.115917770962,294.027992730186,-379.220287242271));
#54030=CARTESIAN_POINT('',(144.115917770962,294.027992730186,-379.220287242271));
#54031=CARTESIAN_POINT('Origin',(148.115917770962,294.027992730186,-379.220287242271));
#54032=CARTESIAN_POINT('Origin',(148.115917770962,328.027992730186,-379.22028724232));
#54033=CARTESIAN_POINT('',(148.115917770964,328.027992731145,281.27971275768));
#54034=CARTESIAN_POINT('',(156.115917770964,328.027992731145,281.27971275768));
#54035=CARTESIAN_POINT('',(148.115917770962,328.027992730186,-379.22028724232));
#54036=CARTESIAN_POINT('',(148.115917770962,328.027992730186,-379.22028724232));
#54037=CARTESIAN_POINT('',(156.115917770962,328.027992730186,-379.22028724232));
#54038=CARTESIAN_POINT('Origin',(148.115917770962,294.027992730186,-379.220287242271));
#54039=CARTESIAN_POINT('',(146.115917770964,294.027992731144,281.279712757729));
#54040=CARTESIAN_POINT('Origin',(148.115917770964,294.027992731144,281.279712757729));
#54041=CARTESIAN_POINT('',(146.115917770962,294.027992730186,-379.220287242271));
#54042=CARTESIAN_POINT('Origin',(148.115917770962,294.027992730186,-379.220287242271));
#54043=CARTESIAN_POINT('',(146.115917770962,294.027992730186,-379.220287242271));
#54044=CARTESIAN_POINT('Origin',(146.115917770962,294.027992730186,-379.220287242271));
#54045=CARTESIAN_POINT('',(146.115917770964,326.027992731144,281.279712757683));
#54046=CARTESIAN_POINT('',(146.115917770964,302.027992731145,281.279712757718));
#54047=CARTESIAN_POINT('',(146.115917770962,326.027992730186,-379.220287242317));
#54048=CARTESIAN_POINT('',(146.115917770962,302.027992730186,-379.220287242282));
#54049=CARTESIAN_POINT('',(146.115917770962,326.027992730186,-379.220287242317));
#54050=CARTESIAN_POINT('Origin',(148.115917770962,326.027992730186,-379.220287242317));
#54051=CARTESIAN_POINT('Origin',(148.115917770964,326.027992731144,281.279712757683));
#54052=CARTESIAN_POINT('Origin',(148.115917770962,326.027992730186,-379.220287242317));
#54053=CARTESIAN_POINT('Origin',(144.115917770962,294.027992730186,-379.220287242271));
#54054=CARTESIAN_POINT('',(144.115917770964,326.027992731144,281.279712757683));
#54055=CARTESIAN_POINT('',(144.115917770964,302.027992731145,281.279712757718));
#54056=CARTESIAN_POINT('',(144.115917770962,326.027992730186,-379.220287242317));
#54057=CARTESIAN_POINT('',(144.115917770962,326.027992730186,-379.220287242317));
#54058=CARTESIAN_POINT('',(144.115917770962,302.027992730186,-379.220287242282));
#54059=CARTESIAN_POINT('Origin',(148.115917770962,326.027992730186,-379.220287242317));
#54060=CARTESIAN_POINT('',(148.115917770964,330.027992731144,281.279712757677));
#54061=CARTESIAN_POINT('Origin',(148.115917770964,326.027992731144,281.279712757683));
#54062=CARTESIAN_POINT('',(148.115917770962,330.027992730186,-379.220287242323));
#54063=CARTESIAN_POINT('',(148.115917770962,330.027992730186,-379.220287242323));
#54064=CARTESIAN_POINT('Origin',(148.115917770962,326.027992730186,-379.220287242317));
#54065=CARTESIAN_POINT('Origin',(148.115917770962,330.027992730186,-379.220287242323));
#54066=CARTESIAN_POINT('',(180.115917770964,330.027992731144,281.279712757677));
#54067=CARTESIAN_POINT('',(156.115917770964,330.027992731144,281.279712757677));
#54068=CARTESIAN_POINT('',(180.115917770962,330.027992730186,-379.220287242323));
#54069=CARTESIAN_POINT('',(180.115917770962,330.027992730186,-379.220287242323));
#54070=CARTESIAN_POINT('',(156.115917770962,330.027992730186,-379.220287242323));
#54071=CARTESIAN_POINT('Origin',(180.115917770962,326.027992730186,-379.220287242317));
#54072=CARTESIAN_POINT('Origin',(180.115917770964,326.027992731144,281.279712757683));
#54073=CARTESIAN_POINT('Origin',(180.115917770962,326.027992730186,-379.220287242317));
#54074=CARTESIAN_POINT('Origin',(164.115917770962,310.027992730186,-379.220287242294));
#54075=CARTESIAN_POINT('Origin',(164.115917770964,310.027992731145,281.279712757706));
#54076=CARTESIAN_POINT('Origin',(180.115917770961,-307.972007269815,-379.220287241397));
#54077=CARTESIAN_POINT('',(148.115917770963,-307.972007268857,280.779712758603));
#54078=CARTESIAN_POINT('',(180.115917770963,-307.972007268857,280.779712758603));
#54079=CARTESIAN_POINT('',(172.115917770963,-307.972007268857,280.779712758603));
#54080=CARTESIAN_POINT('',(180.115917770961,-307.972007269815,-379.220287241397));
#54081=CARTESIAN_POINT('',(180.115917770961,-307.972007269815,-379.220287241397));
#54082=CARTESIAN_POINT('',(148.115917770961,-307.972007269815,-379.220287241397));
#54083=CARTESIAN_POINT('',(172.115917770961,-307.972007269815,-379.220287241397));
#54084=CARTESIAN_POINT('',(148.115917770961,-307.972007269815,-379.220287241397));
#54085=CARTESIAN_POINT('Origin',(180.115917770961,-305.972007269815,-379.2202872414));
#54086=CARTESIAN_POINT('',(182.115917770963,-305.972007268857,280.7797127586));
#54087=CARTESIAN_POINT('Origin',(180.115917770963,-305.972007268857,280.7797127586));
#54088=CARTESIAN_POINT('',(182.115917770961,-305.972007269815,-379.2202872414));
#54089=CARTESIAN_POINT('',(182.115917770961,-305.972007269815,-379.2202872414));
#54090=CARTESIAN_POINT('Origin',(180.115917770961,-305.972007269815,-379.2202872414));
#54091=CARTESIAN_POINT('Origin',(182.115917770961,-273.972007269815,-379.220287241446));
#54092=CARTESIAN_POINT('',(182.115917770963,-273.972007268857,280.779712758554));
#54093=CARTESIAN_POINT('',(182.115917770963,-281.972007268857,280.779712758565));
#54094=CARTESIAN_POINT('',(182.115917770961,-273.972007269815,-379.220287241446));
#54095=CARTESIAN_POINT('',(182.115917770961,-273.972007269815,-379.220287241446));
#54096=CARTESIAN_POINT('',(182.115917770961,-281.972007269815,-379.220287241435));
#54097=CARTESIAN_POINT('Origin',(180.115917770961,-273.972007269815,-379.220287241446));
#54098=CARTESIAN_POINT('',(180.115917770963,-271.972007268857,280.779712758551));
#54099=CARTESIAN_POINT('Origin',(180.115917770963,-273.972007268857,280.779712758554));
#54100=CARTESIAN_POINT('',(180.115917770961,-271.972007269815,-379.220287241449));
#54101=CARTESIAN_POINT('',(180.115917770961,-271.972007269815,-379.220287241449));
#54102=CARTESIAN_POINT('Origin',(180.115917770961,-273.972007269815,-379.220287241446));
#54103=CARTESIAN_POINT('Origin',(184.115917770961,-273.972007269815,-379.220287241446));
#54104=CARTESIAN_POINT('',(184.115917770963,-273.972007268857,280.779712758554));
#54105=CARTESIAN_POINT('',(184.115917770963,-305.972007268857,280.7797127586));
#54106=CARTESIAN_POINT('',(184.115917770963,-281.972007268857,280.779712758565));
#54107=CARTESIAN_POINT('',(184.115917770961,-305.972007269815,-379.2202872414));
#54108=CARTESIAN_POINT('',(184.115917770961,-305.972007269815,-379.2202872414));
#54109=CARTESIAN_POINT('',(184.115917770961,-273.972007269815,-379.220287241446));
#54110=CARTESIAN_POINT('',(184.115917770961,-281.972007269815,-379.220287241435));
#54111=CARTESIAN_POINT('',(184.115917770961,-273.972007269815,-379.220287241446));
#54112=CARTESIAN_POINT('Origin',(180.115917770961,-305.972007269815,-379.2202872414));
#54113=CARTESIAN_POINT('',(180.115917770963,-309.972007268857,280.779712758606));
#54114=CARTESIAN_POINT('Origin',(180.115917770963,-305.972007268857,280.7797127586));
#54115=CARTESIAN_POINT('',(180.115917770961,-309.972007269815,-379.220287241394));
#54116=CARTESIAN_POINT('',(180.115917770961,-309.972007269815,-379.220287241394));
#54117=CARTESIAN_POINT('Origin',(180.115917770961,-305.972007269815,-379.2202872414));
#54118=CARTESIAN_POINT('Origin',(180.115917770961,-309.972007269815,-379.220287241394));
#54119=CARTESIAN_POINT('',(148.115917770963,-309.972007268857,280.779712758606));
#54120=CARTESIAN_POINT('',(172.115917770963,-309.972007268857,280.779712758606));
#54121=CARTESIAN_POINT('',(148.115917770961,-309.972007269815,-379.220287241394));
#54122=CARTESIAN_POINT('',(148.115917770961,-309.972007269815,-379.220287241394));
#54123=CARTESIAN_POINT('',(172.115917770961,-309.972007269815,-379.220287241394));
#54124=CARTESIAN_POINT('Origin',(148.115917770961,-305.972007269815,-379.2202872414));
#54125=CARTESIAN_POINT('',(144.115917770963,-305.972007268857,280.7797127586));
#54126=CARTESIAN_POINT('Origin',(148.115917770963,-305.972007268857,280.7797127586));
#54127=CARTESIAN_POINT('',(144.115917770961,-305.972007269815,-379.2202872414));
#54128=CARTESIAN_POINT('',(144.115917770961,-305.972007269815,-379.2202872414));
#54129=CARTESIAN_POINT('Origin',(148.115917770961,-305.972007269815,-379.2202872414));
#54130=CARTESIAN_POINT('Origin',(148.115917770961,-271.972007269815,-379.220287241449));
#54131=CARTESIAN_POINT('',(148.115917770963,-271.972007268857,280.779712758551));
#54132=CARTESIAN_POINT('',(156.115917770963,-271.972007268857,280.779712758551));
#54133=CARTESIAN_POINT('',(148.115917770961,-271.972007269815,-379.220287241449));
#54134=CARTESIAN_POINT('',(148.115917770961,-271.972007269815,-379.220287241449));
#54135=CARTESIAN_POINT('',(156.115917770961,-271.972007269815,-379.220287241449));
#54136=CARTESIAN_POINT('Origin',(148.115917770961,-305.972007269815,-379.2202872414));
#54137=CARTESIAN_POINT('',(146.115917770963,-305.972007268857,280.7797127586));
#54138=CARTESIAN_POINT('Origin',(148.115917770963,-305.972007268857,280.7797127586));
#54139=CARTESIAN_POINT('',(146.115917770961,-305.972007269815,-379.2202872414));
#54140=CARTESIAN_POINT('Origin',(148.115917770961,-305.972007269815,-379.2202872414));
#54141=CARTESIAN_POINT('',(146.115917770961,-305.972007269815,-379.2202872414));
#54142=CARTESIAN_POINT('Origin',(146.115917770961,-305.972007269815,-379.2202872414));
#54143=CARTESIAN_POINT('',(146.115917770963,-273.972007268857,280.779712758554));
#54144=CARTESIAN_POINT('',(146.115917770963,-297.972007268857,280.779712758589));
#54145=CARTESIAN_POINT('',(146.115917770961,-273.972007269815,-379.220287241446));
#54146=CARTESIAN_POINT('',(146.115917770961,-297.972007269815,-379.220287241411));
#54147=CARTESIAN_POINT('',(146.115917770961,-273.972007269815,-379.220287241446));
#54148=CARTESIAN_POINT('Origin',(148.115917770961,-273.972007269815,-379.220287241446));
#54149=CARTESIAN_POINT('Origin',(148.115917770963,-273.972007268857,280.779712758554));
#54150=CARTESIAN_POINT('Origin',(148.115917770961,-273.972007269815,-379.220287241446));
#54151=CARTESIAN_POINT('Origin',(144.115917770961,-305.972007269815,-379.2202872414));
#54152=CARTESIAN_POINT('',(144.115917770963,-273.972007268857,280.779712758554));
#54153=CARTESIAN_POINT('',(144.115917770963,-297.972007268857,280.779712758589));
#54154=CARTESIAN_POINT('',(144.115917770961,-273.972007269815,-379.220287241446));
#54155=CARTESIAN_POINT('',(144.115917770961,-273.972007269815,-379.220287241446));
#54156=CARTESIAN_POINT('',(144.115917770961,-297.972007269815,-379.220287241411));
#54157=CARTESIAN_POINT('Origin',(148.115917770961,-273.972007269815,-379.220287241446));
#54158=CARTESIAN_POINT('',(148.115917770963,-269.972007268857,280.779712758548));
#54159=CARTESIAN_POINT('Origin',(148.115917770963,-273.972007268857,280.779712758554));
#54160=CARTESIAN_POINT('',(148.115917770961,-269.972007269815,-379.220287241452));
#54161=CARTESIAN_POINT('',(148.115917770961,-269.972007269815,-379.220287241452));
#54162=CARTESIAN_POINT('Origin',(148.115917770961,-273.972007269815,-379.220287241446));
#54163=CARTESIAN_POINT('Origin',(148.115917770961,-269.972007269815,-379.220287241452));
#54164=CARTESIAN_POINT('',(180.115917770963,-269.972007268857,280.779712758548));
#54165=CARTESIAN_POINT('',(156.115917770963,-269.972007268857,280.779712758548));
#54166=CARTESIAN_POINT('',(180.115917770961,-269.972007269815,-379.220287241452));
#54167=CARTESIAN_POINT('',(180.115917770961,-269.972007269815,-379.220287241452));
#54168=CARTESIAN_POINT('',(156.115917770961,-269.972007269815,-379.220287241452));
#54169=CARTESIAN_POINT('Origin',(180.115917770961,-273.972007269815,-379.220287241446));
#54170=CARTESIAN_POINT('Origin',(180.115917770963,-273.972007268857,280.779712758554));
#54171=CARTESIAN_POINT('Origin',(180.115917770961,-273.972007269815,-379.220287241446));
#54172=CARTESIAN_POINT('Origin',(164.115917770961,-289.972007269815,-379.220287241423));
#54173=CARTESIAN_POINT('Origin',(164.115917770963,-289.972007268857,280.779712758577));
#54174=CARTESIAN_POINT('Origin',(154.115917770964,-299.972007268829,300.779712758592));
#54175=CARTESIAN_POINT('',(180.115917770964,-273.9720072688,320.779712758554));
#54176=CARTESIAN_POINT('',(184.115917770964,-269.972007268806,316.779712758548));
#54177=CARTESIAN_POINT('Origin',(180.115917770964,-273.972007268806,316.779712758554));
#54178=CARTESIAN_POINT('',(148.115917770964,-305.9720072688,320.7797127586));
#54179=CARTESIAN_POINT('',(158.115917770964,-295.9720072688,320.779712758586));
#54180=CARTESIAN_POINT('',(144.115917770964,-309.972007268806,316.779712758606));
#54181=CARTESIAN_POINT('Origin',(148.115917770964,-305.972007268806,316.7797127586));
#54182=CARTESIAN_POINT('',(144.115917770964,-309.972007268852,284.779712758606));
#54183=CARTESIAN_POINT('',(144.115917770964,-309.972007268817,308.779712758606));
#54184=CARTESIAN_POINT('',(148.115917770964,-305.972007268858,280.7797127586));
#54185=CARTESIAN_POINT('Origin',(148.115917770964,-305.972007268852,284.7797127586));
#54186=CARTESIAN_POINT('',(180.115917770964,-273.972007268858,280.779712758554));
#54187=CARTESIAN_POINT('',(150.115917770964,-303.972007268858,280.779712758597));
#54188=CARTESIAN_POINT('',(184.115917770964,-269.972007268852,284.779712758548));
#54189=CARTESIAN_POINT('Origin',(180.115917770964,-273.972007268852,284.779712758554));
#54190=CARTESIAN_POINT('',(184.115917770964,-269.972007268841,292.779712758548));
#54191=CARTESIAN_POINT('',(180.115917770964,-273.972007268803,318.779712758554));
#54192=CARTESIAN_POINT('',(148.115917770964,-305.972007268803,318.7797127586));
#54193=CARTESIAN_POINT('',(158.115917770964,-295.972007268803,318.779712758586));
#54194=CARTESIAN_POINT('',(182.115917770964,-271.972007268806,316.779712758551));
#54195=CARTESIAN_POINT('Origin',(180.115917770964,-273.972007268806,316.779712758554));
#54196=CARTESIAN_POINT('',(182.115917770964,-271.972007268852,284.779712758551));
#54197=CARTESIAN_POINT('',(182.115917770964,-271.972007268841,292.779712758551));
#54198=CARTESIAN_POINT('',(180.115917770964,-273.972007268855,282.779712758554));
#54199=CARTESIAN_POINT('Origin',(180.115917770964,-273.972007268852,284.779712758554));
#54200=CARTESIAN_POINT('',(148.115917770964,-305.972007268855,282.7797127586));
#54201=CARTESIAN_POINT('',(150.115917770964,-303.972007268855,282.779712758597));
#54202=CARTESIAN_POINT('',(146.115917770964,-307.972007268852,284.779712758603));
#54203=CARTESIAN_POINT('Origin',(148.115917770964,-305.972007268852,284.7797127586));
#54204=CARTESIAN_POINT('',(146.115917770964,-307.972007268806,316.779712758603));
#54205=CARTESIAN_POINT('',(146.115917770964,-307.972007268817,308.779712758603));
#54206=CARTESIAN_POINT('Origin',(148.115917770964,-305.972007268806,316.7797127586));
#54207=CARTESIAN_POINT('Origin',(148.115917770964,-309.972007268855,282.779712758606));
#54208=CARTESIAN_POINT('',(180.115917770964,294.527992731153,282.779712757729));
#54209=CARTESIAN_POINT('',(180.115917770964,-309.972007268855,282.779712758606));
#54210=CARTESIAN_POINT('',(148.115917770964,326.527992731175,282.779712757682));
#54211=CARTESIAN_POINT('',(470.365917770976,4.27799273094074,282.779712758149));
#54212=CARTESIAN_POINT('',(148.115917770964,-309.972007268855,282.779712758606));
#54213=CARTESIAN_POINT('Origin',(180.115917770964,-309.972007268852,284.779712758606));
#54214=CARTESIAN_POINT('',(182.115917770964,292.527992731154,284.779712757732));
#54215=CARTESIAN_POINT('',(182.115917770964,-309.972007268852,284.779712758606));
#54216=CARTESIAN_POINT('Origin',(180.115917770964,294.527992731156,284.779712757729));
#54217=CARTESIAN_POINT('Origin',(182.115917770964,-309.972007268852,284.779712758606));
#54218=CARTESIAN_POINT('',(182.115917770964,292.5279927312,316.779712757732));
#54219=CARTESIAN_POINT('',(182.115917770964,-309.972007268806,316.779712758606));
#54220=CARTESIAN_POINT('',(182.115917770964,292.527992731166,292.779712757732));
#54221=CARTESIAN_POINT('Origin',(180.115917770964,-309.972007268806,316.779712758606));
#54222=CARTESIAN_POINT('',(180.115917770964,294.527992731205,318.779712757729));
#54223=CARTESIAN_POINT('',(180.115917770964,-309.972007268803,318.779712758606));
#54224=CARTESIAN_POINT('Origin',(180.115917770964,294.527992731202,316.779712757729));
#54225=CARTESIAN_POINT('Origin',(148.115917770964,-309.972007268852,284.779712758606));
#54226=CARTESIAN_POINT('',(144.115917770964,330.527992731148,284.779712757677));
#54227=CARTESIAN_POINT('',(144.115917770964,-309.972007268852,284.779712758606));
#54228=CARTESIAN_POINT('',(148.115917770964,326.527992731172,280.779712757682));
#54229=CARTESIAN_POINT('Origin',(148.115917770964,326.527992731178,284.779712757682));
#54230=CARTESIAN_POINT('',(148.115917770964,-309.972007268858,280.779712758606));
#54231=CARTESIAN_POINT('Origin',(148.115917770964,-309.972007268806,316.779712758606));
#54232=CARTESIAN_POINT('',(148.115917770964,326.52799273123,320.779712757682));
#54233=CARTESIAN_POINT('',(148.115917770964,-309.9720072688,320.779712758606));
#54234=CARTESIAN_POINT('',(144.115917770964,330.527992731194,316.779712757677));
#54235=CARTESIAN_POINT('Origin',(148.115917770964,326.527992731224,316.779712757682));
#54236=CARTESIAN_POINT('',(144.115917770964,-309.972007268806,316.779712758606));
#54237=CARTESIAN_POINT('Origin',(180.115917770964,-309.9720072688,320.779712758606));
#54238=CARTESIAN_POINT('',(180.115917770964,294.527992731208,320.779712757729));
#54239=CARTESIAN_POINT('',(180.115917770964,-309.9720072688,320.779712758606));
#54240=CARTESIAN_POINT('',(478.365917770971,-3.7220072690041,320.77971275816));
#54241=CARTESIAN_POINT('Origin',(474.365917770973,0.277992730966865,300.779712758155));
#54242=CARTESIAN_POINT('',(144.115917770964,330.527992731183,308.779712757677));
#54243=CARTESIAN_POINT('',(184.115917770964,290.527992731199,316.779712757735));
#54244=CARTESIAN_POINT('Origin',(180.115917770964,294.527992731202,316.779712757729));
#54245=CARTESIAN_POINT('',(184.115917770964,290.527992731153,284.779712757735));
#54246=CARTESIAN_POINT('',(184.115917770964,290.527992731164,292.779712757735));
#54247=CARTESIAN_POINT('',(180.115917770964,294.52799273115,280.779712757729));
#54248=CARTESIAN_POINT('Origin',(180.115917770964,294.527992731156,284.779712757729));
#54249=CARTESIAN_POINT('',(470.365917770976,4.27799273093786,280.779712758149));
#54250=CARTESIAN_POINT('',(148.115917770964,326.527992731227,318.779712757682));
#54251=CARTESIAN_POINT('',(478.365917770971,-3.72200726900701,318.779712758161));
#54252=CARTESIAN_POINT('',(146.115917770964,328.527992731225,316.77971275768));
#54253=CARTESIAN_POINT('Origin',(148.115917770964,326.527992731224,316.779712757682));
#54254=CARTESIAN_POINT('',(146.115917770964,328.527992731179,284.77971275768));
#54255=CARTESIAN_POINT('',(146.115917770964,328.527992731214,308.77971275768));
#54256=CARTESIAN_POINT('Origin',(148.115917770964,326.527992731178,284.779712757682));
#54257=CARTESIAN_POINT('Origin',(180.115917770964,-309.972007268803,318.779712758606));
#54258=CARTESIAN_POINT('',(148.115917770964,-309.972007268803,318.779712758606));
#54259=CARTESIAN_POINT('Origin',(180.115917770964,-309.972007268806,316.779712758606));
#54260=CARTESIAN_POINT('',(184.115917770964,-309.972007268806,316.779712758606));
#54261=CARTESIAN_POINT('Origin',(148.115917770964,-309.972007268852,284.779712758606));
#54262=CARTESIAN_POINT('',(146.115917770964,-309.972007268852,284.779712758606));
#54263=CARTESIAN_POINT('Origin',(146.115917770964,-309.972007268806,316.779712758606));
#54264=CARTESIAN_POINT('',(146.115917770964,-309.972007268806,316.779712758606));
#54265=CARTESIAN_POINT('Origin',(148.115917770964,-309.972007268806,316.779712758606));
#54266=CARTESIAN_POINT('Origin',(144.115917770964,-309.972007268806,316.779712758606));
#54267=CARTESIAN_POINT('Origin',(148.115917770964,-309.972007268858,280.779712758606));
#54268=CARTESIAN_POINT('',(180.115917770964,-309.972007268858,280.779712758606));
#54269=CARTESIAN_POINT('Origin',(180.115917770964,-309.972007268852,284.779712758606));
#54270=CARTESIAN_POINT('',(184.115917770964,-309.972007268852,284.779712758606));
#54271=CARTESIAN_POINT('Origin',(184.115917770964,-309.972007268852,284.779712758606));
#54272=CARTESIAN_POINT('Origin',(483.61591777097,-299.972007268829,300.779712758591));
#54273=CARTESIAN_POINT('',(489.61591777097,-305.9720072688,320.779712758599));
#54274=CARTESIAN_POINT('',(493.61591777097,-309.972007268806,316.779712758605));
#54275=CARTESIAN_POINT('Origin',(489.61591777097,-305.972007268806,316.779712758599));
#54276=CARTESIAN_POINT('',(457.61591777097,-273.9720072688,320.779712758553));
#54277=CARTESIAN_POINT('',(487.61591777097,-303.9720072688,320.779712758596));
#54278=CARTESIAN_POINT('',(453.61591777097,-269.972007268806,316.779712758547));
#54279=CARTESIAN_POINT('Origin',(457.61591777097,-273.972007268806,316.779712758553));
#54280=CARTESIAN_POINT('',(453.61591777097,-269.972007268852,284.779712758547));
#54281=CARTESIAN_POINT('',(453.61591777097,-269.972007268817,308.779712758547));
#54282=CARTESIAN_POINT('',(457.61591777097,-273.972007268858,280.779712758553));
#54283=CARTESIAN_POINT('Origin',(457.61591777097,-273.972007268852,284.779712758553));
#54284=CARTESIAN_POINT('',(489.61591777097,-305.972007268858,280.779712758599));
#54285=CARTESIAN_POINT('',(479.61591777097,-295.972007268858,280.779712758585));
#54286=CARTESIAN_POINT('',(493.61591777097,-309.972007268852,284.779712758605));
#54287=CARTESIAN_POINT('Origin',(489.61591777097,-305.972007268852,284.779712758599));
#54288=CARTESIAN_POINT('',(493.61591777097,-309.972007268841,292.779712758605));
#54289=CARTESIAN_POINT('',(489.61591777097,-305.972007268803,318.779712758599));
#54290=CARTESIAN_POINT('',(457.61591777097,-273.972007268803,318.779712758553));
#54291=CARTESIAN_POINT('',(487.61591777097,-303.972007268803,318.779712758596));
#54292=CARTESIAN_POINT('',(491.61591777097,-307.972007268806,316.779712758602));
#54293=CARTESIAN_POINT('Origin',(489.61591777097,-305.972007268806,316.779712758599));
#54294=CARTESIAN_POINT('',(491.61591777097,-307.972007268852,284.779712758602));
#54295=CARTESIAN_POINT('',(491.61591777097,-307.972007268841,292.779712758602));
#54296=CARTESIAN_POINT('',(489.61591777097,-305.972007268855,282.779712758599));
#54297=CARTESIAN_POINT('Origin',(489.61591777097,-305.972007268852,284.779712758599));
#54298=CARTESIAN_POINT('',(457.61591777097,-273.972007268855,282.779712758553));
#54299=CARTESIAN_POINT('',(479.61591777097,-295.972007268855,282.779712758585));
#54300=CARTESIAN_POINT('',(455.61591777097,-271.972007268852,284.77971275855));
#54301=CARTESIAN_POINT('Origin',(457.61591777097,-273.972007268852,284.779712758553));
#54302=CARTESIAN_POINT('',(455.61591777097,-271.972007268806,316.77971275855));
#54303=CARTESIAN_POINT('',(455.61591777097,-271.972007268817,308.77971275855));
#54304=CARTESIAN_POINT('Origin',(457.61591777097,-273.972007268806,316.779712758553));
#54305=CARTESIAN_POINT('Origin',(457.61591777097,-309.972007268855,282.779712758605));
#54306=CARTESIAN_POINT('',(489.61591777097,326.527992731175,282.779712757681));
#54307=CARTESIAN_POINT('',(489.61591777097,-309.972007268855,282.779712758605));
#54308=CARTESIAN_POINT('',(457.61591777097,294.527992731153,282.779712757728));
#54309=CARTESIAN_POINT('',(159.365917770963,-3.72200726905991,282.779712758162));
#54310=CARTESIAN_POINT('',(457.61591777097,-309.972007268855,282.779712758605));
#54311=CARTESIAN_POINT('Origin',(489.61591777097,-309.972007268852,284.779712758605));
#54312=CARTESIAN_POINT('',(491.61591777097,328.527992731179,284.779712757678));
#54313=CARTESIAN_POINT('',(491.61591777097,-309.972007268852,284.779712758605));
#54314=CARTESIAN_POINT('Origin',(489.61591777097,326.527992731178,284.779712757681));
#54315=CARTESIAN_POINT('Origin',(491.61591777097,-309.972007268852,284.779712758605));
#54316=CARTESIAN_POINT('',(491.61591777097,328.527992731225,316.779712757678));
#54317=CARTESIAN_POINT('',(491.61591777097,-309.972007268806,316.779712758605));
#54318=CARTESIAN_POINT('',(491.61591777097,328.52799273119,292.779712757678));
#54319=CARTESIAN_POINT('Origin',(489.61591777097,-309.972007268806,316.779712758605));
#54320=CARTESIAN_POINT('',(489.61591777097,326.527992731227,318.779712757681));
#54321=CARTESIAN_POINT('',(489.61591777097,-309.972007268803,318.779712758605));
#54322=CARTESIAN_POINT('Origin',(489.61591777097,326.527992731224,316.779712757681));
#54323=CARTESIAN_POINT('Origin',(457.61591777097,-309.972007268852,284.779712758605));
#54324=CARTESIAN_POINT('',(453.61591777097,290.527992731153,284.779712757734));
#54325=CARTESIAN_POINT('',(453.61591777097,-309.972007268852,284.779712758605));
#54326=CARTESIAN_POINT('',(457.61591777097,294.52799273115,280.779712757728));
#54327=CARTESIAN_POINT('Origin',(457.61591777097,294.527992731156,284.779712757728));
#54328=CARTESIAN_POINT('',(457.61591777097,-309.972007268858,280.779712758605));
#54329=CARTESIAN_POINT('Origin',(453.61591777097,-309.972007268806,316.779712758605));
#54330=CARTESIAN_POINT('',(453.61591777097,290.527992731199,316.779712757734));
#54331=CARTESIAN_POINT('',(453.61591777097,-309.972007268806,316.779712758605));
#54332=CARTESIAN_POINT('',(453.61591777097,290.527992731188,308.779712757734));
#54333=CARTESIAN_POINT('Origin',(457.61591777097,-309.972007268806,316.779712758605));
#54334=CARTESIAN_POINT('',(457.61591777097,294.527992731208,320.779712757728));
#54335=CARTESIAN_POINT('',(457.61591777097,-309.9720072688,320.779712758605));
#54336=CARTESIAN_POINT('Origin',(457.61591777097,294.527992731202,316.779712757728));
#54337=CARTESIAN_POINT('Origin',(489.61591777097,-309.9720072688,320.779712758605));
#54338=CARTESIAN_POINT('',(489.61591777097,326.52799273123,320.779712757681));
#54339=CARTESIAN_POINT('',(489.61591777097,-309.9720072688,320.779712758605));
#54340=CARTESIAN_POINT('',(167.365917770958,4.27799273099524,320.77971275815));
#54341=CARTESIAN_POINT('Origin',(163.365917770961,0.27799273096619,300.779712758156));
#54342=CARTESIAN_POINT('',(493.61591777097,330.527992731194,316.779712757675));
#54343=CARTESIAN_POINT('Origin',(489.61591777097,326.527992731224,316.779712757681));
#54344=CARTESIAN_POINT('',(493.61591777097,330.527992731148,284.779712757675));
#54345=CARTESIAN_POINT('',(493.61591777097,330.527992731159,292.779712757675));
#54346=CARTESIAN_POINT('',(489.61591777097,326.527992731172,280.779712757681));
#54347=CARTESIAN_POINT('Origin',(489.61591777097,326.527992731178,284.779712757681));
#54348=CARTESIAN_POINT('',(159.365917770963,-3.72200726906282,280.779712758162));
#54349=CARTESIAN_POINT('',(457.61591777097,294.527992731205,318.779712757728));
#54350=CARTESIAN_POINT('',(167.365917770958,4.27799273099236,318.77971275815));
#54351=CARTESIAN_POINT('',(455.61591777097,292.5279927312,316.779712757731));
#54352=CARTESIAN_POINT('Origin',(457.61591777097,294.527992731202,316.779712757728));
#54353=CARTESIAN_POINT('',(455.61591777097,292.527992731154,284.779712757731));
#54354=CARTESIAN_POINT('',(455.61591777097,292.527992731189,308.779712757731));
#54355=CARTESIAN_POINT('Origin',(457.61591777097,294.527992731156,284.779712757728));
#54356=CARTESIAN_POINT('Origin',(489.61591777097,-309.972007268803,318.779712758605));
#54357=CARTESIAN_POINT('',(457.61591777097,-309.972007268803,318.779712758605));
#54358=CARTESIAN_POINT('Origin',(489.61591777097,-309.972007268806,316.779712758605));
#54359=CARTESIAN_POINT('',(493.61591777097,-309.972007268806,316.779712758605));
#54360=CARTESIAN_POINT('Origin',(457.61591777097,-309.972007268852,284.779712758605));
#54361=CARTESIAN_POINT('',(455.61591777097,-309.972007268852,284.779712758605));
#54362=CARTESIAN_POINT('Origin',(455.61591777097,-309.972007268806,316.779712758605));
#54363=CARTESIAN_POINT('',(455.61591777097,-309.972007268806,316.779712758605));
#54364=CARTESIAN_POINT('Origin',(457.61591777097,-309.972007268806,316.779712758605));
#54365=CARTESIAN_POINT('Origin',(457.61591777097,-309.972007268858,280.779712758605));
#54366=CARTESIAN_POINT('',(489.61591777097,-309.972007268858,280.779712758605));
#54367=CARTESIAN_POINT('Origin',(489.61591777097,-309.972007268852,284.779712758605));
#54368=CARTESIAN_POINT('',(493.61591777097,-309.972007268852,284.779712758605));
#54369=CARTESIAN_POINT('Origin',(493.61591777097,-309.972007268852,284.779712758605));
#54370=CARTESIAN_POINT('Origin',(309.115917771081,146.027992731188,301.279712757927));
#54371=CARTESIAN_POINT('',(457.615917770964,294.527992731203,321.279712757697));
#54372=CARTESIAN_POINT('',(489.615917770942,326.527992731203,321.279712757678));
#54373=CARTESIAN_POINT('',(305.115917771072,142.027992731206,321.279712757788));
#54374=CARTESIAN_POINT('',(453.61591777097,290.5279927312,317.2797127577));
#54375=CARTESIAN_POINT('Origin',(457.615917770968,294.5279927312,317.279712757697));
#54376=CARTESIAN_POINT('',(453.615917770998,290.527992731181,285.2797127577));
#54377=CARTESIAN_POINT('',(453.615917770991,290.527992731186,293.279712757966));
#54378=CARTESIAN_POINT('',(457.615917770999,294.527992731179,281.279712757697));
#54379=CARTESIAN_POINT('Origin',(457.615917770995,294.527992731181,285.279712757697));
#54380=CARTESIAN_POINT('',(489.615917770977,326.527992731179,281.279712757678));
#54381=CARTESIAN_POINT('',(313.115917771089,150.02799273117,281.279712757783));
#54382=CARTESIAN_POINT('',(493.615917770964,330.527992731181,285.279712757676));
#54383=CARTESIAN_POINT('Origin',(489.615917770973,326.527992731181,285.279712757678));
#54384=CARTESIAN_POINT('',(493.615917770964,330.5279927312,317.279712757676));
#54385=CARTESIAN_POINT('',(493.615917770964,330.527992731196,309.279712757676));
#54386=CARTESIAN_POINT('Origin',(489.615917770946,326.5279927312,317.279712757678));
#54387=CARTESIAN_POINT('',(491.615917770972,328.527992731181,285.279712757677));
#54388=CARTESIAN_POINT('',(491.615917770944,328.5279927312,317.279712757677));
#54389=CARTESIAN_POINT('',(491.615917770951,328.527992731196,309.279712757976));
#54390=CARTESIAN_POINT('',(489.615917770975,326.52799273118,283.279712757678));
#54391=CARTESIAN_POINT('Origin',(489.615917770973,326.527992731181,285.279712757678));
#54392=CARTESIAN_POINT('',(457.615917770997,294.52799273118,283.279712757697));
#54393=CARTESIAN_POINT('',(313.115917771089,150.027992731172,283.279712757783));
#54394=CARTESIAN_POINT('',(455.615917770997,292.527992731181,285.279712757699));
#54395=CARTESIAN_POINT('Origin',(457.615917770995,294.527992731181,285.279712757697));
#54396=CARTESIAN_POINT('',(455.615917770969,292.5279927312,317.279712757699));
#54397=CARTESIAN_POINT('',(455.61591777099,292.527992731186,293.279712757967));
#54398=CARTESIAN_POINT('',(457.615917770966,294.527992731201,319.279712757697));
#54399=CARTESIAN_POINT('Origin',(457.615917770968,294.5279927312,317.279712757697));
#54400=CARTESIAN_POINT('',(489.615917770944,326.527992731201,319.279712757678));
#54401=CARTESIAN_POINT('',(305.115917771073,142.027992731204,319.279712757788));
#54402=CARTESIAN_POINT('Origin',(489.615917770946,326.5279927312,317.279712757678));
#54403=CARTESIAN_POINT('Origin',(144.615917770964,292.527992731182,285.2797127577));
#54404=CARTESIAN_POINT('',(182.115917770938,292.527992731182,285.279712757699));
#54405=CARTESIAN_POINT('',(144.615917770964,292.527992731182,285.2797127577));
#54406=CARTESIAN_POINT('',(182.115917770965,292.5279927312,317.2797127577));
#54407=CARTESIAN_POINT('',(182.115917770945,292.527992731186,293.279712757667));
#54408=CARTESIAN_POINT('',(144.615917770964,292.5279927312,317.2797127577));
#54409=CARTESIAN_POINT('Origin',(144.615917770964,294.527992731182,285.279712757698));
#54410=CARTESIAN_POINT('',(180.115917770937,294.52799273118,283.279712757698));
#54411=CARTESIAN_POINT('',(144.615917770964,294.52799273118,283.279712757698));
#54412=CARTESIAN_POINT('Origin',(180.115917770939,294.527992731182,285.279712757698));
#54413=CARTESIAN_POINT('Origin',(144.615917770964,326.52799273118,283.27971275768));
#54414=CARTESIAN_POINT('',(148.115917770959,326.52799273118,283.27971275768));
#54415=CARTESIAN_POINT('',(144.615917770964,326.52799273118,283.27971275768));
#54416=CARTESIAN_POINT('',(150.365917770963,324.277992731175,283.279712757681));
#54417=CARTESIAN_POINT('Origin',(144.615917770964,326.527992731182,285.27971275768));
#54418=CARTESIAN_POINT('',(146.115917770963,328.527992731182,285.279712757678));
#54419=CARTESIAN_POINT('',(144.615917770964,328.527992731182,285.279712757678));
#54420=CARTESIAN_POINT('Origin',(148.115917770961,326.527992731182,285.27971275768));
#54421=CARTESIAN_POINT('Origin',(144.615917770964,326.527992731179,281.27971275768));
#54422=CARTESIAN_POINT('',(180.115917770936,294.527992731179,281.279712757698));
#54423=CARTESIAN_POINT('',(144.615917770964,294.527992731179,281.279712757698));
#54424=CARTESIAN_POINT('',(148.115917770958,326.527992731179,281.27971275768));
#54425=CARTESIAN_POINT('',(150.365917770962,324.277992731173,281.279712757681));
#54426=CARTESIAN_POINT('',(144.615917770964,326.527992731179,281.27971275768));
#54427=CARTESIAN_POINT('Origin',(144.615917770964,294.527992731182,285.279712757698));
#54428=CARTESIAN_POINT('',(184.115917770936,290.527992731182,285.279712757701));
#54429=CARTESIAN_POINT('',(144.615917770964,290.527992731182,285.279712757701));
#54430=CARTESIAN_POINT('Origin',(180.115917770939,294.527992731182,285.279712757698));
#54431=CARTESIAN_POINT('Origin',(144.615917770964,290.527992731182,285.279712757701));
#54432=CARTESIAN_POINT('',(184.115917770964,290.5279927312,317.279712757701));
#54433=CARTESIAN_POINT('',(144.615917770964,290.5279927312,317.279712757701));
#54434=CARTESIAN_POINT('',(184.115917770943,290.527992731186,293.279712757667));
#54435=CARTESIAN_POINT('Origin',(144.615917770964,294.5279927312,317.279712757698));
#54436=CARTESIAN_POINT('',(180.11591777097,294.527992731203,321.279712757698));
#54437=CARTESIAN_POINT('',(144.615917770964,294.527992731203,321.279712757698));
#54438=CARTESIAN_POINT('Origin',(180.115917770967,294.5279927312,317.279712757698));
#54439=CARTESIAN_POINT('Origin',(154.365917770971,320.277992731191,301.279712757675));
#54440=CARTESIAN_POINT('',(148.115917770992,326.527992731203,321.27971275768));
#54441=CARTESIAN_POINT('',(158.365917770979,316.277992731209,321.279712757686));
#54442=CARTESIAN_POINT('',(144.115917770964,330.5279927312,317.279712757677));
#54443=CARTESIAN_POINT('Origin',(148.115917770989,326.5279927312,317.27971275768));
#54444=CARTESIAN_POINT('',(144.115917770964,330.527992731182,285.279712757677));
#54445=CARTESIAN_POINT('',(144.115917770964,330.527992731196,309.279712757677));
#54446=CARTESIAN_POINT('Origin',(148.115917770961,326.527992731182,285.27971275768));
#54447=CARTESIAN_POINT('',(146.11591777099,328.5279927312,317.279712757678));
#54448=CARTESIAN_POINT('',(146.115917770983,328.527992731196,309.279712757677));
#54449=CARTESIAN_POINT('',(148.115917770991,326.527992731202,319.27971275768));
#54450=CARTESIAN_POINT('Origin',(148.115917770989,326.5279927312,317.27971275768));
#54451=CARTESIAN_POINT('',(180.115917770969,294.527992731202,319.279712757698));
#54452=CARTESIAN_POINT('',(158.365917770979,316.277992731207,319.279712757686));
#54453=CARTESIAN_POINT('Origin',(180.115917770967,294.5279927312,317.279712757698));
#54454=CARTESIAN_POINT('Origin',(144.615917770964,328.5279927312,317.279712757678));
#54455=CARTESIAN_POINT('',(144.615917770964,328.5279927312,317.279712757678));
#54456=CARTESIAN_POINT('Origin',(144.615917770964,294.527992731203,321.279712757698));
#54457=CARTESIAN_POINT('',(144.615917770964,326.527992731203,321.27971275768));
#54458=CARTESIAN_POINT('Origin',(144.615917770964,294.5279927312,317.279712757698));
#54459=CARTESIAN_POINT('',(144.615917770964,294.527992731202,319.279712757698));
#54460=CARTESIAN_POINT('Origin',(144.615917770964,294.527992731202,319.279712757698));
#54461=CARTESIAN_POINT('',(144.615917770964,326.527992731202,319.27971275768));
#54462=CARTESIAN_POINT('Origin',(144.615917770964,326.5279927312,317.27971275768));
#54463=CARTESIAN_POINT('Origin',(144.615917770964,326.5279927312,317.27971275768));
#54464=CARTESIAN_POINT('',(144.615917770964,330.5279927312,317.279712757677));
#54465=CARTESIAN_POINT('Origin',(144.615917770964,330.5279927312,317.279712757677));
#54466=CARTESIAN_POINT('',(144.615917770964,330.527992731182,285.279712757677));
#54467=CARTESIAN_POINT('Origin',(144.615917770964,326.527992731182,285.27971275768));
#54468=CARTESIAN_POINT('Origin',(483.61591777097,-299.972007268829,300.779712758591));
#54469=CARTESIAN_POINT('',(457.61591777097,-273.972007268858,280.779712758553));
#54470=CARTESIAN_POINT('',(489.61591777097,-305.972007268858,280.779712758599));
#54471=CARTESIAN_POINT('',(487.61591777097,-303.972007268858,280.779712758596));
#54472=CARTESIAN_POINT('',(453.61591777097,-269.972007268852,284.779712758547));
#54473=CARTESIAN_POINT('Origin',(457.61591777097,-273.972007268852,284.779712758553));
#54474=CARTESIAN_POINT('',(453.61591777097,-269.972007268806,316.779712758547));
#54475=CARTESIAN_POINT('',(453.61591777097,-269.972007268841,292.779712758547));
#54476=CARTESIAN_POINT('',(457.61591777097,-273.9720072688,320.779712758553));
#54477=CARTESIAN_POINT('Origin',(457.61591777097,-273.972007268806,316.779712758553));
#54478=CARTESIAN_POINT('',(489.61591777097,-305.9720072688,320.779712758599));
#54479=CARTESIAN_POINT('',(479.61591777097,-295.9720072688,320.779712758585));
#54480=CARTESIAN_POINT('',(493.61591777097,-309.972007268806,316.779712758605));
#54481=CARTESIAN_POINT('Origin',(489.61591777097,-305.972007268806,316.779712758599));
#54482=CARTESIAN_POINT('',(493.61591777097,-309.972007268852,284.779712758605));
#54483=CARTESIAN_POINT('',(493.61591777097,-309.972007268817,308.779712758605));
#54484=CARTESIAN_POINT('Origin',(489.61591777097,-305.972007268852,284.779712758599));
#54485=CARTESIAN_POINT('',(455.61591777097,-271.972007268852,284.77971275855));
#54486=CARTESIAN_POINT('',(455.61591777097,-271.972007268806,316.77971275855));
#54487=CARTESIAN_POINT('',(455.61591777097,-271.972007268841,292.77971275855));
#54488=CARTESIAN_POINT('',(457.61591777097,-273.972007268855,282.779712758553));
#54489=CARTESIAN_POINT('Origin',(457.61591777097,-273.972007268852,284.779712758553));
#54490=CARTESIAN_POINT('',(489.61591777097,-305.972007268855,282.779712758599));
#54491=CARTESIAN_POINT('',(487.61591777097,-303.972007268855,282.779712758596));
#54492=CARTESIAN_POINT('',(491.61591777097,-307.972007268852,284.779712758602));
#54493=CARTESIAN_POINT('Origin',(489.61591777097,-305.972007268852,284.779712758599));
#54494=CARTESIAN_POINT('',(491.61591777097,-307.972007268806,316.779712758602));
#54495=CARTESIAN_POINT('',(491.61591777097,-307.972007268817,308.779712758602));
#54496=CARTESIAN_POINT('',(489.61591777097,-305.972007268803,318.779712758599));
#54497=CARTESIAN_POINT('Origin',(489.61591777097,-305.972007268806,316.779712758599));
#54498=CARTESIAN_POINT('',(457.61591777097,-273.972007268803,318.779712758553));
#54499=CARTESIAN_POINT('',(479.61591777097,-295.972007268803,318.779712758585));
#54500=CARTESIAN_POINT('Origin',(457.61591777097,-273.972007268806,316.779712758553));
#54501=CARTESIAN_POINT('Origin',(493.61591777097,-307.972007268806,316.779712758602));
#54502=CARTESIAN_POINT('',(146.115917770963,-307.972007268852,284.779712758603));
#54503=CARTESIAN_POINT('',(493.61591777097,-307.972007268852,284.779712758602));
#54504=CARTESIAN_POINT('',(146.115917770963,-307.972007268806,316.779712758603));
#54505=CARTESIAN_POINT('',(146.115917770963,-307.972007268817,308.779712758603));
#54506=CARTESIAN_POINT('',(493.61591777097,-307.972007268806,316.779712758602));
#54507=CARTESIAN_POINT('Origin',(493.61591777097,-305.972007268852,284.779712758599));
#54508=CARTESIAN_POINT('',(148.115917770964,-305.972007268855,282.7797127586));
#54509=CARTESIAN_POINT('',(493.61591777097,-305.972007268855,282.779712758599));
#54510=CARTESIAN_POINT('Origin',(148.115917770964,-305.972007268852,284.7797127586));
#54511=CARTESIAN_POINT('Origin',(493.61591777097,-305.972007268855,282.779712758599));
#54512=CARTESIAN_POINT('',(180.115917770963,-273.972007268855,282.779712758554));
#54513=CARTESIAN_POINT('',(493.61591777097,-273.972007268855,282.779712758553));
#54514=CARTESIAN_POINT('',(324.865917770967,-129.222007268852,282.779712758343));
#54515=CARTESIAN_POINT('Origin',(493.61591777097,-273.972007268852,284.779712758553));
#54516=CARTESIAN_POINT('',(182.115917770964,-271.972007268852,284.779712758551));
#54517=CARTESIAN_POINT('',(493.61591777097,-271.972007268852,284.77971275855));
#54518=CARTESIAN_POINT('Origin',(180.115917770963,-273.972007268852,284.779712758554));
#54519=CARTESIAN_POINT('Origin',(493.61591777097,-273.9720072688,320.779712758553));
#54520=CARTESIAN_POINT('',(180.115917770964,-273.9720072688,320.779712758554));
#54521=CARTESIAN_POINT('',(493.61591777097,-273.9720072688,320.779712758553));
#54522=CARTESIAN_POINT('',(148.115917770964,-305.9720072688,320.7797127586));
#54523=CARTESIAN_POINT('',(332.865917770967,-121.222007268797,320.779712758332));
#54524=CARTESIAN_POINT('',(493.61591777097,-305.9720072688,320.779712758599));
#54525=CARTESIAN_POINT('Origin',(493.61591777097,-273.972007268806,316.779712758553));
#54526=CARTESIAN_POINT('',(184.115917770964,-269.972007268806,316.779712758548));
#54527=CARTESIAN_POINT('',(493.61591777097,-269.972007268806,316.779712758547));
#54528=CARTESIAN_POINT('Origin',(180.115917770964,-273.972007268806,316.779712758554));
#54529=CARTESIAN_POINT('Origin',(493.61591777097,-269.972007268852,284.779712758547));
#54530=CARTESIAN_POINT('',(184.115917770964,-269.972007268852,284.779712758548));
#54531=CARTESIAN_POINT('',(493.61591777097,-269.972007268852,284.779712758547));
#54532=CARTESIAN_POINT('',(184.115917770964,-269.97200726884,292.779712758548));
#54533=CARTESIAN_POINT('Origin',(493.61591777097,-273.972007268852,284.779712758553));
#54534=CARTESIAN_POINT('',(180.115917770963,-273.972007268858,280.779712758554));
#54535=CARTESIAN_POINT('',(493.61591777097,-273.972007268858,280.779712758553));
#54536=CARTESIAN_POINT('Origin',(180.115917770963,-273.972007268852,284.779712758554));
#54537=CARTESIAN_POINT('Origin',(328.865917770967,-125.222007268826,300.779712758337));
#54538=CARTESIAN_POINT('',(148.115917770964,-305.972007268858,280.7797127586));
#54539=CARTESIAN_POINT('',(324.865917770967,-129.222007268855,280.779712758343));
#54540=CARTESIAN_POINT('',(144.11591777097,-309.972007268852,284.779712758606));
#54541=CARTESIAN_POINT('Origin',(148.115917770964,-305.972007268852,284.7797127586));
#54542=CARTESIAN_POINT('',(144.11591777097,-309.972007268806,316.779712758606));
#54543=CARTESIAN_POINT('',(144.11591777097,-309.972007268817,308.779712758606));
#54544=CARTESIAN_POINT('Origin',(148.115917770964,-305.972007268806,316.7797127586));
#54545=CARTESIAN_POINT('',(182.115917770964,-271.972007268806,316.779712758551));
#54546=CARTESIAN_POINT('',(182.115917770963,-271.97200726884,292.779712758551));
#54547=CARTESIAN_POINT('',(180.115917770964,-273.972007268803,318.779712758554));
#54548=CARTESIAN_POINT('Origin',(180.115917770964,-273.972007268806,316.779712758554));
#54549=CARTESIAN_POINT('',(148.115917770964,-305.972007268803,318.7797127586));
#54550=CARTESIAN_POINT('',(332.865917770967,-121.2220072688,318.779712758332));
#54551=CARTESIAN_POINT('Origin',(148.115917770964,-305.972007268806,316.7797127586));
#54552=CARTESIAN_POINT('Origin',(493.61591777097,-271.972007268852,284.77971275855));
#54553=CARTESIAN_POINT('',(493.61591777097,-271.972007268806,316.77971275855));
#54554=CARTESIAN_POINT('Origin',(493.61591777097,-305.972007268858,280.779712758599));
#54555=CARTESIAN_POINT('',(493.61591777097,-305.972007268858,280.779712758599));
#54556=CARTESIAN_POINT('Origin',(493.61591777097,-305.972007268806,316.779712758599));
#54557=CARTESIAN_POINT('',(493.61591777097,-305.972007268803,318.779712758599));
#54558=CARTESIAN_POINT('Origin',(493.61591777097,-273.972007268803,318.779712758553));
#54559=CARTESIAN_POINT('',(493.61591777097,-273.972007268803,318.779712758553));
#54560=CARTESIAN_POINT('Origin',(493.61591777097,-273.972007268806,316.779712758553));
#54561=CARTESIAN_POINT('Origin',(493.61591777097,-305.972007268806,316.779712758599));
#54562=CARTESIAN_POINT('',(493.61591777097,-309.972007268806,316.779712758605));
#54563=CARTESIAN_POINT('Origin',(493.61591777097,-309.972007268806,316.779712758605));
#54564=CARTESIAN_POINT('',(493.61591777097,-309.972007268852,284.779712758605));
#54565=CARTESIAN_POINT('Origin',(493.61591777097,-305.972007268852,284.779712758599));
#54566=CARTESIAN_POINT('Origin',(144.115917770962,-307.972007269816,-250.999999448107));
#54567=CARTESIAN_POINT('',(453.615917770962,-307.972007269816,-218.999999448108));
#54568=CARTESIAN_POINT('',(453.615917770962,-307.972007269816,-250.999999448108));
#54569=CARTESIAN_POINT('',(453.615917770962,-307.972007269816,-242.999999448108));
#54570=CARTESIAN_POINT('',(184.115917770962,-307.972007269816,-250.999999448107));
#54571=CARTESIAN_POINT('',(144.115917770962,-307.972007269816,-250.999999448107));
#54572=CARTESIAN_POINT('',(184.115917770962,-307.972007269816,-218.999999448107));
#54573=CARTESIAN_POINT('',(184.115917770962,-307.972007269816,-242.999999448107));
#54574=CARTESIAN_POINT('',(144.115917770962,-307.972007269816,-218.999999448107));
#54575=CARTESIAN_POINT('Origin',(144.115917770962,-305.972007269816,-250.999999448107));
#54576=CARTESIAN_POINT('',(453.615917770962,-305.972007269816,-252.999999448108));
#54577=CARTESIAN_POINT('Origin',(453.615917770962,-305.972007269816,-250.999999448108));
#54578=CARTESIAN_POINT('',(184.115917770962,-305.972007269816,-252.999999448107));
#54579=CARTESIAN_POINT('',(144.115917770962,-305.972007269816,-252.999999448107));
#54580=CARTESIAN_POINT('Origin',(184.115917770962,-305.972007269816,-250.999999448107));
#54581=CARTESIAN_POINT('Origin',(144.115917770962,-273.972007269816,-252.999999448107));
#54582=CARTESIAN_POINT('',(453.615917770962,-273.972007269816,-252.999999448108));
#54583=CARTESIAN_POINT('',(453.615917770962,-281.972007269816,-252.999999448108));
#54584=CARTESIAN_POINT('',(184.115917770962,-273.972007269816,-252.999999448107));
#54585=CARTESIAN_POINT('',(144.115917770962,-273.972007269816,-252.999999448107));
#54586=CARTESIAN_POINT('',(184.115917770962,-281.972007269816,-252.999999448107));
#54587=CARTESIAN_POINT('Origin',(144.115917770962,-273.972007269816,-250.999999448107));
#54588=CARTESIAN_POINT('',(453.615917770962,-271.972007269816,-250.999999448108));
#54589=CARTESIAN_POINT('Origin',(453.615917770962,-273.972007269816,-250.999999448108));
#54590=CARTESIAN_POINT('',(184.115917770962,-271.972007269816,-250.999999448107));
#54591=CARTESIAN_POINT('',(144.115917770962,-271.972007269816,-250.999999448107));
#54592=CARTESIAN_POINT('Origin',(184.115917770962,-273.972007269816,-250.999999448107));
#54593=CARTESIAN_POINT('Origin',(144.115917770962,-273.972007269816,-254.999999448107));
#54594=CARTESIAN_POINT('',(453.615917770962,-273.972007269816,-254.999999448108));
#54595=CARTESIAN_POINT('',(453.615917770962,-305.972007269816,-254.999999448108));
#54596=CARTESIAN_POINT('',(453.615917770962,-281.972007269816,-254.999999448108));
#54597=CARTESIAN_POINT('',(184.115917770962,-305.972007269816,-254.999999448107));
#54598=CARTESIAN_POINT('',(144.115917770962,-305.972007269816,-254.999999448107));
#54599=CARTESIAN_POINT('',(184.115917770962,-273.972007269816,-254.999999448107));
#54600=CARTESIAN_POINT('',(184.115917770962,-281.972007269816,-254.999999448107));
#54601=CARTESIAN_POINT('',(144.115917770962,-273.972007269816,-254.999999448107));
#54602=CARTESIAN_POINT('Origin',(144.115917770962,-305.972007269816,-250.999999448107));
#54603=CARTESIAN_POINT('',(453.615917770962,-309.972007269816,-250.999999448108));
#54604=CARTESIAN_POINT('Origin',(453.615917770962,-305.972007269816,-250.999999448108));
#54605=CARTESIAN_POINT('',(184.115917770962,-309.972007269816,-250.999999448107));
#54606=CARTESIAN_POINT('',(144.115917770962,-309.972007269816,-250.999999448107));
#54607=CARTESIAN_POINT('Origin',(184.115917770962,-305.972007269816,-250.999999448107));
#54608=CARTESIAN_POINT('Origin',(144.115917770962,-309.972007269816,-250.999999448107));
#54609=CARTESIAN_POINT('',(453.615917770962,-309.972007269816,-218.999999448108));
#54610=CARTESIAN_POINT('',(453.615917770962,-309.972007269816,-242.999999448108));
#54611=CARTESIAN_POINT('',(184.115917770962,-309.972007269816,-218.999999448107));
#54612=CARTESIAN_POINT('',(144.115917770962,-309.972007269816,-218.999999448107));
#54613=CARTESIAN_POINT('',(184.115917770962,-309.972007269816,-242.999999448107));
#54614=CARTESIAN_POINT('Origin',(144.115917770962,-305.972007269816,-218.999999448107));
#54615=CARTESIAN_POINT('',(453.615917770962,-305.972007269816,-214.999999448108));
#54616=CARTESIAN_POINT('Origin',(453.615917770962,-305.972007269816,-218.999999448108));
#54617=CARTESIAN_POINT('',(184.115917770962,-305.972007269816,-214.999999448107));
#54618=CARTESIAN_POINT('',(144.115917770962,-305.972007269816,-214.999999448107));
#54619=CARTESIAN_POINT('Origin',(184.115917770962,-305.972007269816,-218.999999448107));
#54620=CARTESIAN_POINT('Origin',(144.115917770962,-271.972007269816,-218.999999448107));
#54621=CARTESIAN_POINT('',(453.615917770962,-271.972007269816,-218.999999448108));
#54622=CARTESIAN_POINT('',(453.615917770962,-271.972007269816,-226.999999448108));
#54623=CARTESIAN_POINT('',(184.115917770962,-271.972007269816,-218.999999448107));
#54624=CARTESIAN_POINT('',(144.115917770962,-271.972007269816,-218.999999448107));
#54625=CARTESIAN_POINT('',(184.115917770962,-271.972007269816,-226.999999448107));
#54626=CARTESIAN_POINT('Origin',(144.115917770962,-305.972007269816,-218.999999448107));
#54627=CARTESIAN_POINT('',(453.615917770962,-305.972007269816,-216.999999448108));
#54628=CARTESIAN_POINT('Origin',(453.615917770962,-305.972007269816,-218.999999448108));
#54629=CARTESIAN_POINT('',(184.115917770962,-305.972007269816,-216.999999448107));
#54630=CARTESIAN_POINT('Origin',(184.115917770962,-305.972007269816,-218.999999448107));
#54631=CARTESIAN_POINT('',(144.115917770962,-305.972007269816,-216.999999448107));
#54632=CARTESIAN_POINT('Origin',(144.115917770962,-305.972007269816,-216.999999448107));
#54633=CARTESIAN_POINT('',(453.615917770962,-273.972007269816,-216.999999448108));
#54634=CARTESIAN_POINT('',(453.615917770962,-297.972007269816,-216.999999448108));
#54635=CARTESIAN_POINT('',(184.115917770962,-273.972007269816,-216.999999448107));
#54636=CARTESIAN_POINT('',(184.115917770962,-297.972007269816,-216.999999448107));
#54637=CARTESIAN_POINT('',(144.115917770962,-273.972007269816,-216.999999448107));
#54638=CARTESIAN_POINT('Origin',(144.115917770962,-273.972007269816,-218.999999448107));
#54639=CARTESIAN_POINT('Origin',(453.615917770962,-273.972007269816,-218.999999448108));
#54640=CARTESIAN_POINT('Origin',(184.115917770962,-273.972007269816,-218.999999448107));
#54641=CARTESIAN_POINT('Origin',(144.115917770962,-305.972007269816,-214.999999448107));
#54642=CARTESIAN_POINT('',(453.615917770962,-273.972007269816,-214.999999448108));
#54643=CARTESIAN_POINT('',(453.615917770962,-297.972007269816,-214.999999448108));
#54644=CARTESIAN_POINT('',(184.115917770962,-273.972007269816,-214.999999448107));
#54645=CARTESIAN_POINT('',(144.115917770962,-273.972007269816,-214.999999448107));
#54646=CARTESIAN_POINT('',(184.115917770962,-297.972007269816,-214.999999448107));
#54647=CARTESIAN_POINT('Origin',(144.115917770962,-273.972007269816,-218.999999448107));
#54648=CARTESIAN_POINT('',(453.615917770962,-269.972007269816,-218.999999448108));
#54649=CARTESIAN_POINT('Origin',(453.615917770962,-273.972007269816,-218.999999448108));
#54650=CARTESIAN_POINT('',(184.115917770962,-269.972007269816,-218.999999448107));
#54651=CARTESIAN_POINT('',(144.115917770962,-269.972007269816,-218.999999448107));
#54652=CARTESIAN_POINT('Origin',(184.115917770962,-273.972007269816,-218.999999448107));
#54653=CARTESIAN_POINT('Origin',(144.115917770962,-269.972007269816,-218.999999448107));
#54654=CARTESIAN_POINT('',(453.615917770962,-269.972007269816,-250.999999448108));
#54655=CARTESIAN_POINT('',(453.615917770962,-269.972007269816,-226.999999448108));
#54656=CARTESIAN_POINT('',(184.115917770962,-269.972007269816,-250.999999448107));
#54657=CARTESIAN_POINT('',(144.115917770962,-269.972007269816,-250.999999448107));
#54658=CARTESIAN_POINT('',(184.115917770962,-269.972007269816,-226.999999448107));
#54659=CARTESIAN_POINT('Origin',(144.115917770962,-273.972007269816,-250.999999448107));
#54660=CARTESIAN_POINT('Origin',(453.615917770962,-273.972007269816,-250.999999448108));
#54661=CARTESIAN_POINT('Origin',(184.115917770962,-273.972007269816,-250.999999448107));
#54662=CARTESIAN_POINT('Origin',(184.115917770962,-289.972007269816,-234.999999448107));
#54663=CARTESIAN_POINT('Origin',(453.615917770962,-289.972007269816,-234.999999448108));
#54664=CARTESIAN_POINT('Origin',(144.115917770962,292.027992730186,-250.999999448106));
#54665=CARTESIAN_POINT('',(453.615917770962,292.027992730186,-218.999999448107));
#54666=CARTESIAN_POINT('',(453.615917770962,292.027992730186,-250.999999448107));
#54667=CARTESIAN_POINT('',(453.615917770962,292.027992730186,-242.999999448107));
#54668=CARTESIAN_POINT('',(184.115917770962,292.027992730186,-250.999999448106));
#54669=CARTESIAN_POINT('',(144.115917770962,292.027992730186,-250.999999448106));
#54670=CARTESIAN_POINT('',(184.115917770962,292.027992730186,-218.999999448106));
#54671=CARTESIAN_POINT('',(184.115917770962,292.027992730186,-242.999999448106));
#54672=CARTESIAN_POINT('',(144.115917770962,292.027992730186,-218.999999448106));
#54673=CARTESIAN_POINT('Origin',(144.115917770962,294.027992730186,-250.999999448106));
#54674=CARTESIAN_POINT('',(453.615917770962,294.027992730186,-252.999999448107));
#54675=CARTESIAN_POINT('Origin',(453.615917770962,294.027992730186,-250.999999448107));
#54676=CARTESIAN_POINT('',(184.115917770962,294.027992730186,-252.999999448106));
#54677=CARTESIAN_POINT('',(144.115917770962,294.027992730186,-252.999999448106));
#54678=CARTESIAN_POINT('Origin',(184.115917770962,294.027992730186,-250.999999448106));
#54679=CARTESIAN_POINT('Origin',(144.115917770962,326.027992730186,-252.999999448106));
#54680=CARTESIAN_POINT('',(453.615917770962,326.027992730186,-252.999999448107));
#54681=CARTESIAN_POINT('',(453.615917770962,318.027992730186,-252.999999448107));
#54682=CARTESIAN_POINT('',(184.115917770962,326.027992730186,-252.999999448106));
#54683=CARTESIAN_POINT('',(144.115917770962,326.027992730186,-252.999999448106));
#54684=CARTESIAN_POINT('',(184.115917770962,318.027992730186,-252.999999448106));
#54685=CARTESIAN_POINT('Origin',(144.115917770962,326.027992730186,-250.999999448106));
#54686=CARTESIAN_POINT('',(453.615917770962,328.027992730186,-250.999999448107));
#54687=CARTESIAN_POINT('Origin',(453.615917770962,326.027992730186,-250.999999448107));
#54688=CARTESIAN_POINT('',(184.115917770962,328.027992730186,-250.999999448106));
#54689=CARTESIAN_POINT('',(144.115917770962,328.027992730186,-250.999999448106));
#54690=CARTESIAN_POINT('Origin',(184.115917770962,326.027992730186,-250.999999448106));
#54691=CARTESIAN_POINT('Origin',(144.115917770962,326.027992730186,-254.999999448106));
#54692=CARTESIAN_POINT('',(453.615917770962,326.027992730186,-254.999999448107));
#54693=CARTESIAN_POINT('',(453.615917770962,294.027992730186,-254.999999448107));
#54694=CARTESIAN_POINT('',(453.615917770962,318.027992730186,-254.999999448107));
#54695=CARTESIAN_POINT('',(184.115917770962,294.027992730186,-254.999999448106));
#54696=CARTESIAN_POINT('',(144.115917770962,294.027992730186,-254.999999448106));
#54697=CARTESIAN_POINT('',(184.115917770962,326.027992730186,-254.999999448106));
#54698=CARTESIAN_POINT('',(184.115917770962,318.027992730186,-254.999999448106));
#54699=CARTESIAN_POINT('',(144.115917770962,326.027992730186,-254.999999448106));
#54700=CARTESIAN_POINT('Origin',(144.115917770962,294.027992730186,-250.999999448106));
#54701=CARTESIAN_POINT('',(453.615917770962,290.027992730186,-250.999999448107));
#54702=CARTESIAN_POINT('Origin',(453.615917770962,294.027992730186,-250.999999448107));
#54703=CARTESIAN_POINT('',(184.115917770962,290.027992730186,-250.999999448106));
#54704=CARTESIAN_POINT('',(144.115917770962,290.027992730186,-250.999999448106));
#54705=CARTESIAN_POINT('Origin',(184.115917770962,294.027992730186,-250.999999448106));
#54706=CARTESIAN_POINT('Origin',(144.115917770962,290.027992730186,-250.999999448106));
#54707=CARTESIAN_POINT('',(453.615917770962,290.027992730186,-218.999999448107));
#54708=CARTESIAN_POINT('',(453.615917770962,290.027992730186,-242.999999448107));
#54709=CARTESIAN_POINT('',(184.115917770962,290.027992730186,-218.999999448106));
#54710=CARTESIAN_POINT('',(144.115917770962,290.027992730186,-218.999999448106));
#54711=CARTESIAN_POINT('',(184.115917770962,290.027992730186,-242.999999448106));
#54712=CARTESIAN_POINT('Origin',(144.115917770962,294.027992730186,-218.999999448106));
#54713=CARTESIAN_POINT('',(453.615917770962,294.027992730186,-214.999999448107));
#54714=CARTESIAN_POINT('Origin',(453.615917770962,294.027992730186,-218.999999448107));
#54715=CARTESIAN_POINT('',(184.115917770962,294.027992730186,-214.999999448106));
#54716=CARTESIAN_POINT('',(144.115917770962,294.027992730186,-214.999999448106));
#54717=CARTESIAN_POINT('Origin',(184.115917770962,294.027992730186,-218.999999448106));
#54718=CARTESIAN_POINT('Origin',(144.115917770962,328.027992730186,-218.999999448106));
#54719=CARTESIAN_POINT('',(453.615917770962,328.027992730186,-218.999999448107));
#54720=CARTESIAN_POINT('',(453.615917770962,328.027992730186,-226.999999448107));
#54721=CARTESIAN_POINT('',(184.115917770962,328.027992730186,-218.999999448106));
#54722=CARTESIAN_POINT('',(144.115917770962,328.027992730186,-218.999999448106));
#54723=CARTESIAN_POINT('',(184.115917770962,328.027992730186,-226.999999448106));
#54724=CARTESIAN_POINT('Origin',(144.115917770962,294.027992730186,-218.999999448106));
#54725=CARTESIAN_POINT('',(453.615917770962,294.027992730186,-216.999999448107));
#54726=CARTESIAN_POINT('Origin',(453.615917770962,294.027992730186,-218.999999448107));
#54727=CARTESIAN_POINT('',(184.115917770962,294.027992730186,-216.999999448106));
#54728=CARTESIAN_POINT('Origin',(184.115917770962,294.027992730186,-218.999999448106));
#54729=CARTESIAN_POINT('',(144.115917770962,294.027992730186,-216.999999448106));
#54730=CARTESIAN_POINT('Origin',(144.115917770962,294.027992730186,-216.999999448106));
#54731=CARTESIAN_POINT('',(453.615917770962,326.027992730186,-216.999999448107));
#54732=CARTESIAN_POINT('',(453.615917770962,302.027992730186,-216.999999448107));
#54733=CARTESIAN_POINT('',(184.115917770962,326.027992730186,-216.999999448106));
#54734=CARTESIAN_POINT('',(184.115917770962,302.027992730186,-216.999999448106));
#54735=CARTESIAN_POINT('',(144.115917770962,326.027992730186,-216.999999448106));
#54736=CARTESIAN_POINT('Origin',(144.115917770962,326.027992730186,-218.999999448106));
#54737=CARTESIAN_POINT('Origin',(453.615917770962,326.027992730186,-218.999999448107));
#54738=CARTESIAN_POINT('Origin',(184.115917770962,326.027992730186,-218.999999448106));
#54739=CARTESIAN_POINT('Origin',(144.115917770962,294.027992730186,-214.999999448106));
#54740=CARTESIAN_POINT('',(453.615917770962,326.027992730186,-214.999999448107));
#54741=CARTESIAN_POINT('',(453.615917770962,302.027992730186,-214.999999448107));
#54742=CARTESIAN_POINT('',(184.115917770962,326.027992730186,-214.999999448106));
#54743=CARTESIAN_POINT('',(144.115917770962,326.027992730186,-214.999999448106));
#54744=CARTESIAN_POINT('',(184.115917770962,302.027992730186,-214.999999448106));
#54745=CARTESIAN_POINT('Origin',(144.115917770962,326.027992730186,-218.999999448106));
#54746=CARTESIAN_POINT('',(453.615917770962,330.027992730186,-218.999999448107));
#54747=CARTESIAN_POINT('Origin',(453.615917770962,326.027992730186,-218.999999448107));
#54748=CARTESIAN_POINT('',(184.115917770962,330.027992730186,-218.999999448106));
#54749=CARTESIAN_POINT('',(144.115917770962,330.027992730186,-218.999999448106));
#54750=CARTESIAN_POINT('Origin',(184.115917770962,326.027992730186,-218.999999448106));
#54751=CARTESIAN_POINT('Origin',(144.115917770962,330.027992730186,-218.999999448106));
#54752=CARTESIAN_POINT('',(453.615917770962,330.027992730186,-250.999999448107));
#54753=CARTESIAN_POINT('',(453.615917770962,330.027992730186,-226.999999448107));
#54754=CARTESIAN_POINT('',(184.115917770962,330.027992730186,-250.999999448106));
#54755=CARTESIAN_POINT('',(144.115917770962,330.027992730186,-250.999999448106));
#54756=CARTESIAN_POINT('',(184.115917770962,330.027992730186,-226.999999448106));
#54757=CARTESIAN_POINT('Origin',(144.115917770962,326.027992730186,-250.999999448106));
#54758=CARTESIAN_POINT('Origin',(453.615917770962,326.027992730186,-250.999999448107));
#54759=CARTESIAN_POINT('Origin',(184.115917770962,326.027992730186,-250.999999448106));
#54760=CARTESIAN_POINT('Origin',(184.115917770962,310.027992730186,-234.999999448106));
#54761=CARTESIAN_POINT('Origin',(453.615917770962,310.027992730186,-234.999999448107));
#54762=CARTESIAN_POINT('Origin',(302.865917770965,330.027992730186,-216.999999448107));
#54763=CARTESIAN_POINT('',(334.865917770965,-269.972007269814,-216.999999448108));
#54764=CARTESIAN_POINT('',(302.865917770965,-269.972007269814,-216.999999448108));
#54765=CARTESIAN_POINT('',(310.865917770965,-269.972007269814,-216.999999448108));
#54766=CARTESIAN_POINT('',(302.865917770965,290.027992730186,-216.999999448107));
#54767=CARTESIAN_POINT('',(302.865917770965,330.027992730186,-216.999999448107));
#54768=CARTESIAN_POINT('',(334.865917770965,290.027992730186,-216.999999448107));
#54769=CARTESIAN_POINT('',(310.865917770965,290.027992730186,-216.999999448107));
#54770=CARTESIAN_POINT('',(334.865917770965,330.027992730186,-216.999999448107));
#54771=CARTESIAN_POINT('Origin',(302.865917770965,330.027992730186,-218.999999448107));
#54772=CARTESIAN_POINT('',(300.865917770965,-269.972007269814,-218.999999448108));
#54773=CARTESIAN_POINT('Origin',(302.865917770965,-269.972007269814,-218.999999448108));
#54774=CARTESIAN_POINT('',(300.865917770965,290.027992730186,-218.999999448107));
#54775=CARTESIAN_POINT('',(300.865917770965,330.027992730186,-218.999999448107));
#54776=CARTESIAN_POINT('Origin',(302.865917770965,290.027992730186,-218.999999448107));
#54777=CARTESIAN_POINT('Origin',(300.865917770965,330.027992730186,-250.999999448107));
#54778=CARTESIAN_POINT('',(300.865917770965,-269.972007269814,-250.999999448108));
#54779=CARTESIAN_POINT('',(300.865917770965,-269.972007269814,-242.999999448108));
#54780=CARTESIAN_POINT('',(300.865917770965,290.027992730186,-250.999999448107));
#54781=CARTESIAN_POINT('',(300.865917770965,330.027992730186,-250.999999448107));
#54782=CARTESIAN_POINT('',(300.865917770965,290.027992730186,-242.999999448107));
#54783=CARTESIAN_POINT('Origin',(302.865917770965,330.027992730186,-250.999999448107));
#54784=CARTESIAN_POINT('',(302.865917770965,-269.972007269814,-252.999999448108));
#54785=CARTESIAN_POINT('Origin',(302.865917770965,-269.972007269814,-250.999999448108));
#54786=CARTESIAN_POINT('',(302.865917770965,290.027992730186,-252.999999448107));
#54787=CARTESIAN_POINT('',(302.865917770965,330.027992730186,-252.999999448107));
#54788=CARTESIAN_POINT('Origin',(302.865917770965,290.027992730186,-250.999999448107));
#54789=CARTESIAN_POINT('Origin',(298.865917770965,330.027992730186,-250.999999448107));
#54790=CARTESIAN_POINT('',(298.865917770965,-269.972007269814,-250.999999448108));
#54791=CARTESIAN_POINT('',(298.865917770965,-269.972007269814,-218.999999448108));
#54792=CARTESIAN_POINT('',(298.865917770965,-269.972007269814,-242.999999448108));
#54793=CARTESIAN_POINT('',(298.865917770965,290.027992730186,-218.999999448107));
#54794=CARTESIAN_POINT('',(298.865917770965,330.027992730186,-218.999999448107));
#54795=CARTESIAN_POINT('',(298.865917770965,290.027992730186,-250.999999448107));
#54796=CARTESIAN_POINT('',(298.865917770965,290.027992730186,-242.999999448107));
#54797=CARTESIAN_POINT('',(298.865917770965,330.027992730186,-250.999999448107));
#54798=CARTESIAN_POINT('Origin',(302.865917770965,330.027992730186,-218.999999448107));
#54799=CARTESIAN_POINT('',(302.865917770965,-269.972007269814,-214.999999448108));
#54800=CARTESIAN_POINT('Origin',(302.865917770965,-269.972007269814,-218.999999448108));
#54801=CARTESIAN_POINT('',(302.865917770965,290.027992730186,-214.999999448107));
#54802=CARTESIAN_POINT('',(302.865917770965,330.027992730186,-214.999999448107));
#54803=CARTESIAN_POINT('Origin',(302.865917770965,290.027992730186,-218.999999448107));
#54804=CARTESIAN_POINT('Origin',(302.865917770965,330.027992730186,-214.999999448107));
#54805=CARTESIAN_POINT('',(334.865917770965,-269.972007269814,-214.999999448108));
#54806=CARTESIAN_POINT('',(310.865917770965,-269.972007269814,-214.999999448108));
#54807=CARTESIAN_POINT('',(334.865917770965,290.027992730186,-214.999999448107));
#54808=CARTESIAN_POINT('',(334.865917770965,330.027992730186,-214.999999448107));
#54809=CARTESIAN_POINT('',(310.865917770965,290.027992730186,-214.999999448107));
#54810=CARTESIAN_POINT('Origin',(334.865917770965,330.027992730186,-218.999999448107));
#54811=CARTESIAN_POINT('',(338.865917770965,-269.972007269814,-218.999999448108));
#54812=CARTESIAN_POINT('Origin',(334.865917770965,-269.972007269814,-218.999999448108));
#54813=CARTESIAN_POINT('',(338.865917770965,290.027992730186,-218.999999448107));
#54814=CARTESIAN_POINT('',(338.865917770965,330.027992730186,-218.999999448107));
#54815=CARTESIAN_POINT('Origin',(334.865917770965,290.027992730186,-218.999999448107));
#54816=CARTESIAN_POINT('Origin',(334.865917770965,330.027992730186,-252.999999448107));
#54817=CARTESIAN_POINT('',(334.865917770965,-269.972007269814,-252.999999448108));
#54818=CARTESIAN_POINT('',(326.865917770965,-269.972007269814,-252.999999448108));
#54819=CARTESIAN_POINT('',(334.865917770965,290.027992730186,-252.999999448107));
#54820=CARTESIAN_POINT('',(334.865917770965,330.027992730186,-252.999999448107));
#54821=CARTESIAN_POINT('',(326.865917770965,290.027992730186,-252.999999448107));
#54822=CARTESIAN_POINT('Origin',(334.865917770965,330.027992730186,-218.999999448107));
#54823=CARTESIAN_POINT('',(336.865917770965,-269.972007269814,-218.999999448108));
#54824=CARTESIAN_POINT('Origin',(334.865917770965,-269.972007269814,-218.999999448108));
#54825=CARTESIAN_POINT('',(336.865917770965,290.027992730186,-218.999999448107));
#54826=CARTESIAN_POINT('Origin',(334.865917770965,290.027992730186,-218.999999448107));
#54827=CARTESIAN_POINT('',(336.865917770965,330.027992730186,-218.999999448107));
#54828=CARTESIAN_POINT('Origin',(336.865917770965,330.027992730186,-218.999999448107));
#54829=CARTESIAN_POINT('',(336.865917770965,-269.972007269814,-250.999999448108));
#54830=CARTESIAN_POINT('',(336.865917770965,-269.972007269814,-226.999999448108));
#54831=CARTESIAN_POINT('',(336.865917770965,290.027992730186,-250.999999448107));
#54832=CARTESIAN_POINT('',(336.865917770965,290.027992730186,-226.999999448107));
#54833=CARTESIAN_POINT('',(336.865917770965,330.027992730186,-250.999999448107));
#54834=CARTESIAN_POINT('Origin',(334.865917770965,330.027992730186,-250.999999448107));
#54835=CARTESIAN_POINT('Origin',(334.865917770965,-269.972007269814,-250.999999448108));
#54836=CARTESIAN_POINT('Origin',(334.865917770965,290.027992730186,-250.999999448107));
#54837=CARTESIAN_POINT('Origin',(338.865917770965,330.027992730186,-218.999999448107));
#54838=CARTESIAN_POINT('',(338.865917770965,-269.972007269814,-250.999999448108));
#54839=CARTESIAN_POINT('',(338.865917770965,-269.972007269814,-226.999999448108));
#54840=CARTESIAN_POINT('',(338.865917770965,290.027992730186,-250.999999448107));
#54841=CARTESIAN_POINT('',(338.865917770965,330.027992730186,-250.999999448107));
#54842=CARTESIAN_POINT('',(338.865917770965,290.027992730186,-226.999999448107));
#54843=CARTESIAN_POINT('Origin',(334.865917770965,330.027992730186,-250.999999448107));
#54844=CARTESIAN_POINT('',(334.865917770965,-269.972007269814,-254.999999448108));
#54845=CARTESIAN_POINT('Origin',(334.865917770965,-269.972007269814,-250.999999448108));
#54846=CARTESIAN_POINT('',(334.865917770965,290.027992730186,-254.999999448107));
#54847=CARTESIAN_POINT('',(334.865917770965,330.027992730186,-254.999999448107));
#54848=CARTESIAN_POINT('Origin',(334.865917770965,290.027992730186,-250.999999448107));
#54849=CARTESIAN_POINT('Origin',(334.865917770965,330.027992730186,-254.999999448107));
#54850=CARTESIAN_POINT('',(302.865917770965,-269.972007269814,-254.999999448108));
#54851=CARTESIAN_POINT('',(326.865917770965,-269.972007269814,-254.999999448108));
#54852=CARTESIAN_POINT('',(302.865917770965,290.027992730186,-254.999999448107));
#54853=CARTESIAN_POINT('',(302.865917770965,330.027992730186,-254.999999448107));
#54854=CARTESIAN_POINT('',(326.865917770965,290.027992730186,-254.999999448107));
#54855=CARTESIAN_POINT('Origin',(302.865917770965,330.027992730186,-250.999999448107));
#54856=CARTESIAN_POINT('Origin',(302.865917770965,-269.972007269814,-250.999999448108));
#54857=CARTESIAN_POINT('Origin',(302.865917770965,290.027992730186,-250.999999448107));
#54858=CARTESIAN_POINT('Origin',(318.865917770965,290.027992730186,-234.999999448107));
#54859=CARTESIAN_POINT('Origin',(318.865917770965,-269.972007269814,-234.999999448108));
#54860=CARTESIAN_POINT('Origin',(148.115917770962,-305.972007269816,-379.2202872414));
#54861=CARTESIAN_POINT('',(148.115917770962,-309.972007269816,-379.220287241394));
#54862=CARTESIAN_POINT('',(144.115917770962,-305.972007269816,-379.2202872414));
#54863=CARTESIAN_POINT('Origin',(148.115917770962,-305.972007269816,-379.2202872414));
#54864=CARTESIAN_POINT('',(148.115917770962,-309.972007269823,-384.220287241394));
#54865=CARTESIAN_POINT('',(148.115917770962,-309.972007269816,-379.220287241394));
#54866=CARTESIAN_POINT('',(144.115917770962,-305.972007269823,-384.2202872414));
#54867=CARTESIAN_POINT('Origin',(148.115917770962,-305.972007269823,-384.2202872414));
#54868=CARTESIAN_POINT('',(144.115917770962,-305.972007269816,-379.2202872414));
#54869=CARTESIAN_POINT('Origin',(180.115917770962,-309.972007269816,-379.220287241394));
#54870=CARTESIAN_POINT('',(180.115917770962,-309.972007269816,-379.220287241394));
#54871=CARTESIAN_POINT('',(172.11591777096,-309.972007269816,-379.220287241394));
#54872=CARTESIAN_POINT('',(180.115917770962,-309.972007269823,-384.220287241394));
#54873=CARTESIAN_POINT('',(180.115917770962,-309.972007269816,-379.220287241394));
#54874=CARTESIAN_POINT('',(172.11591777096,-309.972007269823,-384.220287241394));
#54875=CARTESIAN_POINT('Origin',(180.115917770962,-305.972007269816,-379.2202872414));
#54876=CARTESIAN_POINT('',(184.115917770962,-305.972007269816,-379.2202872414));
#54877=CARTESIAN_POINT('Origin',(180.115917770962,-305.972007269816,-379.2202872414));
#54878=CARTESIAN_POINT('',(184.115917770962,-305.972007269823,-384.2202872414));
#54879=CARTESIAN_POINT('',(184.115917770962,-305.972007269816,-379.2202872414));
#54880=CARTESIAN_POINT('Origin',(180.115917770962,-305.972007269823,-384.2202872414));
#54881=CARTESIAN_POINT('Origin',(184.115917770962,-273.972007269816,-379.220287241446));
#54882=CARTESIAN_POINT('',(184.115917770962,-273.972007269816,-379.220287241446));
#54883=CARTESIAN_POINT('',(184.115917770962,-281.972007269816,-379.220287241435));
#54884=CARTESIAN_POINT('',(184.115917770962,-273.972007269823,-384.220287241446));
#54885=CARTESIAN_POINT('',(184.115917770962,-273.972007269816,-379.220287241446));
#54886=CARTESIAN_POINT('',(184.115917770962,-281.972007269823,-384.220287241435));
#54887=CARTESIAN_POINT('Origin',(180.115917770962,-273.972007269816,-379.220287241446));
#54888=CARTESIAN_POINT('',(180.115917770961,-269.972007269816,-379.220287241452));
#54889=CARTESIAN_POINT('Origin',(180.115917770962,-273.972007269816,-379.220287241446));
#54890=CARTESIAN_POINT('',(180.115917770961,-269.972007269823,-384.220287241452));
#54891=CARTESIAN_POINT('',(180.115917770961,-269.972007269816,-379.220287241452));
#54892=CARTESIAN_POINT('Origin',(180.115917770962,-273.972007269823,-384.220287241446));
#54893=CARTESIAN_POINT('Origin',(148.115917770962,-269.972007269816,-379.220287241452));
#54894=CARTESIAN_POINT('',(148.115917770962,-269.972007269816,-379.220287241452));
#54895=CARTESIAN_POINT('',(156.11591777096,-269.972007269816,-379.220287241452));
#54896=CARTESIAN_POINT('',(148.115917770962,-269.972007269823,-384.220287241452));
#54897=CARTESIAN_POINT('',(148.115917770962,-269.972007269816,-379.220287241452));
#54898=CARTESIAN_POINT('',(156.11591777096,-269.972007269823,-384.220287241452));
#54899=CARTESIAN_POINT('Origin',(148.115917770962,-273.972007269816,-379.220287241446));
#54900=CARTESIAN_POINT('',(144.115917770962,-273.972007269816,-379.220287241446));
#54901=CARTESIAN_POINT('Origin',(148.115917770962,-273.972007269816,-379.220287241446));
#54902=CARTESIAN_POINT('',(144.115917770962,-273.972007269823,-384.220287241446));
#54903=CARTESIAN_POINT('',(144.115917770962,-273.972007269816,-379.220287241446));
#54904=CARTESIAN_POINT('Origin',(148.115917770962,-273.972007269823,-384.220287241446));
#54905=CARTESIAN_POINT('Origin',(144.115917770962,-305.972007269816,-379.2202872414));
#54906=CARTESIAN_POINT('',(144.115917770962,-297.972007269816,-379.220287241412));
#54907=CARTESIAN_POINT('',(144.115917770962,-297.972007269823,-384.220287241412));
#54908=CARTESIAN_POINT('Origin',(148.115917770962,-273.972007269816,-379.220287241446));
#54909=CARTESIAN_POINT('',(148.115917770939,-249.972007269814,-379.220287241481));
#54910=CARTESIAN_POINT('',(124.11591777096,-273.972007269756,-379.220287241446));
#54911=CARTESIAN_POINT('Origin',(148.115917770962,-273.972007269816,-379.220287241446));
#54912=CARTESIAN_POINT('',(148.115917770939,-249.972007269821,-384.220287241481));
#54913=CARTESIAN_POINT('',(148.115917770939,-249.972007269814,-379.220287241481));
#54914=CARTESIAN_POINT('',(124.11591777096,-273.972007269763,-384.220287241446));
#54915=CARTESIAN_POINT('Origin',(148.115917770962,-273.972007269823,-384.220287241446));
#54916=CARTESIAN_POINT('',(124.11591777096,-273.972007269756,-379.220287241446));
#54917=CARTESIAN_POINT('Origin',(124.11591777096,-305.972007269872,-379.2202872414));
#54918=CARTESIAN_POINT('',(124.11591777096,-305.972007269872,-379.2202872414));
#54919=CARTESIAN_POINT('',(124.11591777096,-273.972007269756,-379.220287241446));
#54920=CARTESIAN_POINT('',(124.11591777096,-305.972007269879,-384.2202872414));
#54921=CARTESIAN_POINT('',(124.11591777096,-273.972007269763,-384.220287241446));
#54922=CARTESIAN_POINT('',(124.11591777096,-305.972007269872,-379.2202872414));
#54923=CARTESIAN_POINT('Origin',(148.115917770962,-305.972007269816,-379.2202872414));
#54924=CARTESIAN_POINT('',(148.115917770939,-329.972007269817,-379.220287241365));
#54925=CARTESIAN_POINT('Origin',(148.115917770962,-305.972007269816,-379.2202872414));
#54926=CARTESIAN_POINT('',(148.115917770939,-329.972007269824,-384.220287241365));
#54927=CARTESIAN_POINT('Origin',(148.115917770962,-305.972007269823,-384.2202872414));
#54928=CARTESIAN_POINT('',(148.115917770939,-329.972007269817,-379.220287241365));
#54929=CARTESIAN_POINT('Origin',(180.11591777091,-329.972007269817,-379.220287241365));
#54930=CARTESIAN_POINT('',(180.11591777091,-329.972007269817,-379.220287241365));
#54931=CARTESIAN_POINT('',(148.115917770939,-329.972007269817,-379.220287241365));
#54932=CARTESIAN_POINT('',(180.11591777091,-329.972007269824,-384.220287241365));
#54933=CARTESIAN_POINT('',(148.115917770939,-329.972007269824,-384.220287241365));
#54934=CARTESIAN_POINT('',(180.11591777091,-329.972007269817,-379.220287241365));
#54935=CARTESIAN_POINT('Origin',(180.115917770962,-305.972007269816,-379.2202872414));
#54936=CARTESIAN_POINT('',(204.115917770963,-305.972007269872,-379.2202872414));
#54937=CARTESIAN_POINT('Origin',(180.115917770962,-305.972007269816,-379.2202872414));
#54938=CARTESIAN_POINT('',(204.115917770963,-305.972007269879,-384.2202872414));
#54939=CARTESIAN_POINT('Origin',(180.115917770962,-305.972007269823,-384.2202872414));
#54940=CARTESIAN_POINT('',(204.115917770963,-305.972007269872,-379.2202872414));
#54941=CARTESIAN_POINT('Origin',(204.115917770963,-273.972007269756,-379.220287241447));
#54942=CARTESIAN_POINT('',(204.115917770963,-273.972007269756,-379.220287241447));
#54943=CARTESIAN_POINT('',(204.115917770963,-305.972007269872,-379.2202872414));
#54944=CARTESIAN_POINT('',(204.115917770963,-273.972007269763,-384.220287241447));
#54945=CARTESIAN_POINT('',(204.115917770963,-305.972007269879,-384.2202872414));
#54946=CARTESIAN_POINT('',(204.115917770963,-273.972007269756,-379.220287241447));
#54947=CARTESIAN_POINT('Origin',(180.115917770962,-273.972007269816,-379.220287241446));
#54948=CARTESIAN_POINT('',(180.11591777091,-249.972007269814,-379.220287241481));
#54949=CARTESIAN_POINT('Origin',(180.115917770962,-273.972007269816,-379.220287241446));
#54950=CARTESIAN_POINT('',(180.11591777091,-249.972007269821,-384.220287241481));
#54951=CARTESIAN_POINT('Origin',(180.115917770962,-273.972007269823,-384.220287241446));
#54952=CARTESIAN_POINT('',(180.11591777091,-249.972007269814,-379.220287241481));
#54953=CARTESIAN_POINT('Origin',(148.115917770939,-249.972007269814,-379.220287241481));
#54954=CARTESIAN_POINT('',(180.11591777091,-249.972007269814,-379.220287241481));
#54955=CARTESIAN_POINT('',(180.11591777091,-249.972007269821,-384.220287241481));
#54956=CARTESIAN_POINT('Origin',(164.115917770959,-289.972007269816,-379.220287241423));
#54957=CARTESIAN_POINT('Origin',(164.115917770959,-289.972007269823,-384.220287241423));
#54958=CARTESIAN_POINT('Origin',(457.615917770968,294.027992730186,-379.220287242272));
#54959=CARTESIAN_POINT('',(457.615917770968,290.027992730186,-379.220287242266));
#54960=CARTESIAN_POINT('',(453.615917770968,294.027992730186,-379.220287242272));
#54961=CARTESIAN_POINT('Origin',(457.615917770968,294.027992730186,-379.220287242272));
#54962=CARTESIAN_POINT('',(457.615917770968,290.027992730179,-384.220287242266));
#54963=CARTESIAN_POINT('',(457.615917770968,290.027992730186,-379.220287242266));
#54964=CARTESIAN_POINT('',(453.615917770968,294.027992730179,-384.220287242272));
#54965=CARTESIAN_POINT('Origin',(457.615917770968,294.027992730179,-384.220287242272));
#54966=CARTESIAN_POINT('',(453.615917770968,294.027992730186,-379.220287242272));
#54967=CARTESIAN_POINT('Origin',(489.615917770968,290.027992730186,-379.220287242266));
#54968=CARTESIAN_POINT('',(489.615917770968,290.027992730186,-379.220287242266));
#54969=CARTESIAN_POINT('',(481.615917770966,290.027992730186,-379.220287242266));
#54970=CARTESIAN_POINT('',(489.615917770968,290.027992730179,-384.220287242266));
#54971=CARTESIAN_POINT('',(489.615917770968,290.027992730186,-379.220287242266));
#54972=CARTESIAN_POINT('',(481.615917770966,290.027992730179,-384.220287242266));
#54973=CARTESIAN_POINT('Origin',(489.615917770968,294.027992730186,-379.220287242272));
#54974=CARTESIAN_POINT('',(493.615917770968,294.027992730186,-379.220287242272));
#54975=CARTESIAN_POINT('Origin',(489.615917770968,294.027992730186,-379.220287242272));
#54976=CARTESIAN_POINT('',(493.615917770968,294.027992730179,-384.220287242272));
#54977=CARTESIAN_POINT('',(493.615917770968,294.027992730186,-379.220287242272));
#54978=CARTESIAN_POINT('Origin',(489.615917770968,294.027992730179,-384.220287242272));
#54979=CARTESIAN_POINT('Origin',(493.615917770968,326.027992730186,-379.220287242318));
#54980=CARTESIAN_POINT('',(493.615917770968,326.027992730186,-379.220287242318));
#54981=CARTESIAN_POINT('',(493.615917770968,318.027992730186,-379.220287242307));
#54982=CARTESIAN_POINT('',(493.615917770968,326.027992730179,-384.220287242318));
#54983=CARTESIAN_POINT('',(493.615917770968,326.027992730186,-379.220287242318));
#54984=CARTESIAN_POINT('',(493.615917770968,318.027992730179,-384.220287242307));
#54985=CARTESIAN_POINT('Origin',(489.615917770968,326.027992730186,-379.220287242318));
#54986=CARTESIAN_POINT('',(489.615917770967,330.027992730186,-379.220287242324));
#54987=CARTESIAN_POINT('Origin',(489.615917770968,326.027992730186,-379.220287242318));
#54988=CARTESIAN_POINT('',(489.615917770967,330.027992730179,-384.220287242324));
#54989=CARTESIAN_POINT('',(489.615917770967,330.027992730186,-379.220287242324));
#54990=CARTESIAN_POINT('Origin',(489.615917770968,326.027992730179,-384.220287242318));
#54991=CARTESIAN_POINT('Origin',(457.615917770968,330.027992730186,-379.220287242324));
#54992=CARTESIAN_POINT('',(457.615917770968,330.027992730186,-379.220287242324));
#54993=CARTESIAN_POINT('',(465.615917770966,330.027992730186,-379.220287242324));
#54994=CARTESIAN_POINT('',(457.615917770968,330.027992730179,-384.220287242324));
#54995=CARTESIAN_POINT('',(457.615917770968,330.027992730186,-379.220287242324));
#54996=CARTESIAN_POINT('',(465.615917770966,330.027992730179,-384.220287242324));
#54997=CARTESIAN_POINT('Origin',(457.615917770968,326.027992730186,-379.220287242318));
#54998=CARTESIAN_POINT('',(453.615917770968,326.027992730186,-379.220287242318));
#54999=CARTESIAN_POINT('Origin',(457.615917770968,326.027992730186,-379.220287242318));
#55000=CARTESIAN_POINT('',(453.615917770968,326.027992730179,-384.220287242318));
#55001=CARTESIAN_POINT('',(453.615917770968,326.027992730186,-379.220287242318));
#55002=CARTESIAN_POINT('Origin',(457.615917770968,326.027992730179,-384.220287242318));
#55003=CARTESIAN_POINT('Origin',(453.615917770968,294.027992730186,-379.220287242272));
#55004=CARTESIAN_POINT('',(453.615917770968,302.027992730186,-379.220287242283));
#55005=CARTESIAN_POINT('',(453.615917770968,302.027992730179,-384.220287242283));
#55006=CARTESIAN_POINT('Origin',(457.615917770968,326.027992730186,-379.220287242318));
#55007=CARTESIAN_POINT('',(457.615917770945,350.027992730188,-379.220287242353));
#55008=CARTESIAN_POINT('',(433.615917770966,326.027992730246,-379.220287242318));
#55009=CARTESIAN_POINT('Origin',(457.615917770968,326.027992730186,-379.220287242318));
#55010=CARTESIAN_POINT('',(457.615917770945,350.027992730181,-384.220287242353));
#55011=CARTESIAN_POINT('',(457.615917770945,350.027992730188,-379.220287242353));
#55012=CARTESIAN_POINT('',(433.615917770966,326.027992730239,-384.220287242318));
#55013=CARTESIAN_POINT('Origin',(457.615917770968,326.027992730179,-384.220287242318));
#55014=CARTESIAN_POINT('',(433.615917770966,326.027992730246,-379.220287242318));
#55015=CARTESIAN_POINT('Origin',(433.615917770966,294.02799273013,-379.220287242272));
#55016=CARTESIAN_POINT('',(433.615917770966,294.02799273013,-379.220287242272));
#55017=CARTESIAN_POINT('',(433.615917770966,326.027992730246,-379.220287242318));
#55018=CARTESIAN_POINT('',(433.615917770966,294.027992730123,-384.220287242272));
#55019=CARTESIAN_POINT('',(433.615917770966,326.027992730239,-384.220287242318));
#55020=CARTESIAN_POINT('',(433.615917770966,294.02799273013,-379.220287242272));
#55021=CARTESIAN_POINT('Origin',(457.615917770968,294.027992730186,-379.220287242272));
#55022=CARTESIAN_POINT('',(457.615917770945,270.027992730185,-379.220287242237));
#55023=CARTESIAN_POINT('Origin',(457.615917770968,294.027992730186,-379.220287242272));
#55024=CARTESIAN_POINT('',(457.615917770945,270.027992730178,-384.220287242237));
#55025=CARTESIAN_POINT('Origin',(457.615917770968,294.027992730179,-384.220287242272));
#55026=CARTESIAN_POINT('',(457.615917770945,270.027992730185,-379.220287242237));
#55027=CARTESIAN_POINT('Origin',(489.615917770916,270.027992730185,-379.220287242237));
#55028=CARTESIAN_POINT('',(489.615917770916,270.027992730185,-379.220287242237));
#55029=CARTESIAN_POINT('',(457.615917770945,270.027992730185,-379.220287242237));
#55030=CARTESIAN_POINT('',(489.615917770916,270.027992730178,-384.220287242237));
#55031=CARTESIAN_POINT('',(457.615917770945,270.027992730178,-384.220287242237));
#55032=CARTESIAN_POINT('',(489.615917770916,270.027992730185,-379.220287242237));
#55033=CARTESIAN_POINT('Origin',(489.615917770968,294.027992730186,-379.220287242272));
#55034=CARTESIAN_POINT('',(513.615917770969,294.02799273013,-379.220287242272));
#55035=CARTESIAN_POINT('Origin',(489.615917770968,294.027992730186,-379.220287242272));
#55036=CARTESIAN_POINT('',(513.615917770969,294.027992730123,-384.220287242272));
#55037=CARTESIAN_POINT('Origin',(489.615917770968,294.027992730179,-384.220287242272));
#55038=CARTESIAN_POINT('',(513.615917770969,294.02799273013,-379.220287242272));
#55039=CARTESIAN_POINT('Origin',(513.615917770969,326.027992730246,-379.220287242318));
#55040=CARTESIAN_POINT('',(513.615917770969,326.027992730246,-379.220287242318));
#55041=CARTESIAN_POINT('',(513.615917770969,294.02799273013,-379.220287242272));
#55042=CARTESIAN_POINT('',(513.615917770969,326.027992730239,-384.220287242318));
#55043=CARTESIAN_POINT('',(513.615917770969,294.027992730123,-384.220287242272));
#55044=CARTESIAN_POINT('',(513.615917770969,326.027992730246,-379.220287242318));
#55045=CARTESIAN_POINT('Origin',(489.615917770968,326.027992730186,-379.220287242318));
#55046=CARTESIAN_POINT('',(489.615917770916,350.027992730188,-379.220287242353));
#55047=CARTESIAN_POINT('Origin',(489.615917770968,326.027992730186,-379.220287242318));
#55048=CARTESIAN_POINT('',(489.615917770916,350.027992730181,-384.220287242353));
#55049=CARTESIAN_POINT('Origin',(489.615917770968,326.027992730179,-384.220287242318));
#55050=CARTESIAN_POINT('',(489.615917770916,350.027992730188,-379.220287242353));
#55051=CARTESIAN_POINT('Origin',(457.615917770945,350.027992730188,-379.220287242353));
#55052=CARTESIAN_POINT('',(489.615917770916,350.027992730188,-379.220287242353));
#55053=CARTESIAN_POINT('',(489.615917770916,350.027992730181,-384.220287242353));
#55054=CARTESIAN_POINT('Origin',(473.615917770965,310.027992730186,-379.220287242295));
#55055=CARTESIAN_POINT('Origin',(473.615917770965,310.027992730179,-384.220287242295));
#55056=CARTESIAN_POINT('Origin',(148.115917770962,294.027992730186,-379.220287242271));
#55057=CARTESIAN_POINT('',(148.115917770962,290.027992730186,-379.220287242265));
#55058=CARTESIAN_POINT('',(144.115917770962,294.027992730186,-379.220287242271));
#55059=CARTESIAN_POINT('Origin',(148.115917770962,294.027992730186,-379.220287242271));
#55060=CARTESIAN_POINT('',(148.115917770962,290.027992730179,-384.220287242265));
#55061=CARTESIAN_POINT('',(148.115917770962,290.027992730186,-379.220287242265));
#55062=CARTESIAN_POINT('',(144.115917770962,294.027992730179,-384.220287242271));
#55063=CARTESIAN_POINT('Origin',(148.115917770962,294.027992730179,-384.220287242271));
#55064=CARTESIAN_POINT('',(144.115917770962,294.027992730186,-379.220287242271));
#55065=CARTESIAN_POINT('Origin',(180.115917770962,290.027992730186,-379.220287242265));
#55066=CARTESIAN_POINT('',(180.115917770962,290.027992730186,-379.220287242265));
#55067=CARTESIAN_POINT('',(172.11591777096,290.027992730186,-379.220287242265));
#55068=CARTESIAN_POINT('',(180.115917770962,290.027992730179,-384.220287242265));
#55069=CARTESIAN_POINT('',(180.115917770962,290.027992730186,-379.220287242265));
#55070=CARTESIAN_POINT('',(172.11591777096,290.027992730179,-384.220287242265));
#55071=CARTESIAN_POINT('Origin',(180.115917770962,294.027992730186,-379.220287242271));
#55072=CARTESIAN_POINT('',(184.115917770962,294.027992730186,-379.220287242271));
#55073=CARTESIAN_POINT('Origin',(180.115917770962,294.027992730186,-379.220287242271));
#55074=CARTESIAN_POINT('',(184.115917770962,294.027992730179,-384.220287242271));
#55075=CARTESIAN_POINT('',(184.115917770962,294.027992730186,-379.220287242271));
#55076=CARTESIAN_POINT('Origin',(180.115917770962,294.027992730179,-384.220287242271));
#55077=CARTESIAN_POINT('Origin',(184.115917770962,326.027992730186,-379.220287242317));
#55078=CARTESIAN_POINT('',(184.115917770962,326.027992730186,-379.220287242317));
#55079=CARTESIAN_POINT('',(184.115917770962,318.027992730186,-379.220287242306));
#55080=CARTESIAN_POINT('',(184.115917770962,326.027992730179,-384.220287242317));
#55081=CARTESIAN_POINT('',(184.115917770962,326.027992730186,-379.220287242317));
#55082=CARTESIAN_POINT('',(184.115917770962,318.027992730179,-384.220287242306));
#55083=CARTESIAN_POINT('Origin',(180.115917770962,326.027992730186,-379.220287242317));
#55084=CARTESIAN_POINT('',(180.115917770961,330.027992730186,-379.220287242323));
#55085=CARTESIAN_POINT('Origin',(180.115917770962,326.027992730186,-379.220287242317));
#55086=CARTESIAN_POINT('',(180.115917770961,330.027992730179,-384.220287242323));
#55087=CARTESIAN_POINT('',(180.115917770961,330.027992730186,-379.220287242323));
#55088=CARTESIAN_POINT('Origin',(180.115917770962,326.027992730179,-384.220287242317));
#55089=CARTESIAN_POINT('Origin',(148.115917770962,330.027992730186,-379.220287242323));
#55090=CARTESIAN_POINT('',(148.115917770962,330.027992730186,-379.220287242323));
#55091=CARTESIAN_POINT('',(156.11591777096,330.027992730186,-379.220287242323));
#55092=CARTESIAN_POINT('',(148.115917770962,330.027992730179,-384.220287242323));
#55093=CARTESIAN_POINT('',(148.115917770962,330.027992730186,-379.220287242323));
#55094=CARTESIAN_POINT('',(156.11591777096,330.027992730179,-384.220287242323));
#55095=CARTESIAN_POINT('Origin',(148.115917770962,326.027992730186,-379.220287242317));
#55096=CARTESIAN_POINT('',(144.115917770962,326.027992730186,-379.220287242317));
#55097=CARTESIAN_POINT('Origin',(148.115917770962,326.027992730186,-379.220287242317));
#55098=CARTESIAN_POINT('',(144.115917770962,326.027992730179,-384.220287242317));
#55099=CARTESIAN_POINT('',(144.115917770962,326.027992730186,-379.220287242317));
#55100=CARTESIAN_POINT('Origin',(148.115917770962,326.027992730179,-384.220287242317));
#55101=CARTESIAN_POINT('Origin',(144.115917770962,294.027992730186,-379.220287242271));
#55102=CARTESIAN_POINT('',(144.115917770962,302.027992730186,-379.220287242282));
#55103=CARTESIAN_POINT('',(144.115917770962,302.027992730179,-384.220287242282));
#55104=CARTESIAN_POINT('Origin',(148.115917770962,326.027992730186,-379.220287242317));
#55105=CARTESIAN_POINT('',(148.115917770939,350.027992730188,-379.220287242352));
#55106=CARTESIAN_POINT('',(124.11591777096,326.027992730246,-379.220287242317));
#55107=CARTESIAN_POINT('Origin',(148.115917770962,326.027992730186,-379.220287242317));
#55108=CARTESIAN_POINT('',(148.115917770939,350.027992730181,-384.220287242352));
#55109=CARTESIAN_POINT('',(148.115917770939,350.027992730188,-379.220287242352));
#55110=CARTESIAN_POINT('',(124.11591777096,326.027992730239,-384.220287242317));
#55111=CARTESIAN_POINT('Origin',(148.115917770962,326.027992730179,-384.220287242317));
#55112=CARTESIAN_POINT('',(124.11591777096,326.027992730246,-379.220287242317));
#55113=CARTESIAN_POINT('Origin',(124.11591777096,294.02799273013,-379.220287242271));
#55114=CARTESIAN_POINT('',(124.11591777096,294.02799273013,-379.220287242271));
#55115=CARTESIAN_POINT('',(124.11591777096,326.027992730246,-379.220287242317));
#55116=CARTESIAN_POINT('',(124.11591777096,294.027992730123,-384.220287242271));
#55117=CARTESIAN_POINT('',(124.11591777096,326.027992730239,-384.220287242317));
#55118=CARTESIAN_POINT('',(124.11591777096,294.02799273013,-379.220287242271));
#55119=CARTESIAN_POINT('Origin',(148.115917770962,294.027992730186,-379.220287242271));
#55120=CARTESIAN_POINT('',(148.115917770939,270.027992730185,-379.220287242236));
#55121=CARTESIAN_POINT('Origin',(148.115917770962,294.027992730186,-379.220287242271));
#55122=CARTESIAN_POINT('',(148.115917770939,270.027992730178,-384.220287242236));
#55123=CARTESIAN_POINT('Origin',(148.115917770962,294.027992730179,-384.220287242271));
#55124=CARTESIAN_POINT('',(148.115917770939,270.027992730185,-379.220287242236));
#55125=CARTESIAN_POINT('Origin',(180.11591777091,270.027992730185,-379.220287242236));
#55126=CARTESIAN_POINT('',(180.11591777091,270.027992730185,-379.220287242236));
#55127=CARTESIAN_POINT('',(148.115917770939,270.027992730185,-379.220287242236));
#55128=CARTESIAN_POINT('',(180.11591777091,270.027992730178,-384.220287242236));
#55129=CARTESIAN_POINT('',(148.115917770939,270.027992730178,-384.220287242236));
#55130=CARTESIAN_POINT('',(180.11591777091,270.027992730185,-379.220287242236));
#55131=CARTESIAN_POINT('Origin',(180.115917770962,294.027992730186,-379.220287242271));
#55132=CARTESIAN_POINT('',(204.115917770963,294.02799273013,-379.220287242271));
#55133=CARTESIAN_POINT('Origin',(180.115917770962,294.027992730186,-379.220287242271));
#55134=CARTESIAN_POINT('',(204.115917770963,294.027992730123,-384.220287242271));
#55135=CARTESIAN_POINT('Origin',(180.115917770962,294.027992730179,-384.220287242271));
#55136=CARTESIAN_POINT('',(204.115917770963,294.02799273013,-379.220287242271));
#55137=CARTESIAN_POINT('Origin',(204.115917770963,326.027992730246,-379.220287242317));
#55138=CARTESIAN_POINT('',(204.115917770963,326.027992730246,-379.220287242317));
#55139=CARTESIAN_POINT('',(204.115917770963,294.02799273013,-379.220287242271));
#55140=CARTESIAN_POINT('',(204.115917770963,326.027992730239,-384.220287242317));
#55141=CARTESIAN_POINT('',(204.115917770963,294.027992730123,-384.220287242271));
#55142=CARTESIAN_POINT('',(204.115917770963,326.027992730246,-379.220287242317));
#55143=CARTESIAN_POINT('Origin',(180.115917770962,326.027992730186,-379.220287242317));
#55144=CARTESIAN_POINT('',(180.11591777091,350.027992730188,-379.220287242352));
#55145=CARTESIAN_POINT('Origin',(180.115917770962,326.027992730186,-379.220287242317));
#55146=CARTESIAN_POINT('',(180.11591777091,350.027992730181,-384.220287242352));
#55147=CARTESIAN_POINT('Origin',(180.115917770962,326.027992730179,-384.220287242317));
#55148=CARTESIAN_POINT('',(180.11591777091,350.027992730188,-379.220287242352));
#55149=CARTESIAN_POINT('Origin',(148.115917770939,350.027992730188,-379.220287242352));
#55150=CARTESIAN_POINT('',(180.11591777091,350.027992730188,-379.220287242352));
#55151=CARTESIAN_POINT('',(180.11591777091,350.027992730181,-384.220287242352));
#55152=CARTESIAN_POINT('Origin',(164.115917770959,310.027992730186,-379.220287242294));
#55153=CARTESIAN_POINT('Origin',(164.115917770959,310.027992730179,-384.220287242294));
#55154=CARTESIAN_POINT('Origin',(457.615917770968,-305.972007269816,-379.220287241401));
#55155=CARTESIAN_POINT('',(457.615917770968,-309.972007269816,-379.220287241395));
#55156=CARTESIAN_POINT('',(453.615917770968,-305.972007269816,-379.220287241401));
#55157=CARTESIAN_POINT('Origin',(457.615917770968,-305.972007269816,-379.220287241401));
#55158=CARTESIAN_POINT('',(457.615917770968,-309.972007269823,-384.220287241395));
#55159=CARTESIAN_POINT('',(457.615917770968,-309.972007269816,-379.220287241395));
#55160=CARTESIAN_POINT('',(453.615917770968,-305.972007269823,-384.220287241401));
#55161=CARTESIAN_POINT('Origin',(457.615917770968,-305.972007269823,-384.220287241401));
#55162=CARTESIAN_POINT('',(453.615917770968,-305.972007269816,-379.220287241401));
#55163=CARTESIAN_POINT('Origin',(489.615917770968,-309.972007269816,-379.220287241395));
#55164=CARTESIAN_POINT('',(489.615917770968,-309.972007269816,-379.220287241395));
#55165=CARTESIAN_POINT('',(481.615917770966,-309.972007269816,-379.220287241395));
#55166=CARTESIAN_POINT('',(489.615917770968,-309.972007269823,-384.220287241395));
#55167=CARTESIAN_POINT('',(489.615917770968,-309.972007269816,-379.220287241395));
#55168=CARTESIAN_POINT('',(481.615917770966,-309.972007269823,-384.220287241395));
#55169=CARTESIAN_POINT('Origin',(489.615917770968,-305.972007269816,-379.220287241401));
#55170=CARTESIAN_POINT('',(493.615917770968,-305.972007269816,-379.220287241401));
#55171=CARTESIAN_POINT('Origin',(489.615917770968,-305.972007269816,-379.220287241401));
#55172=CARTESIAN_POINT('',(493.615917770968,-305.972007269823,-384.220287241401));
#55173=CARTESIAN_POINT('',(493.615917770968,-305.972007269816,-379.220287241401));
#55174=CARTESIAN_POINT('Origin',(489.615917770968,-305.972007269823,-384.220287241401));
#55175=CARTESIAN_POINT('Origin',(493.615917770968,-273.972007269816,-379.220287241448));
#55176=CARTESIAN_POINT('',(493.615917770968,-273.972007269816,-379.220287241448));
#55177=CARTESIAN_POINT('',(493.615917770968,-281.972007269816,-379.220287241436));
#55178=CARTESIAN_POINT('',(493.615917770968,-273.972007269823,-384.220287241448));
#55179=CARTESIAN_POINT('',(493.615917770968,-273.972007269816,-379.220287241448));
#55180=CARTESIAN_POINT('',(493.615917770968,-281.972007269823,-384.220287241436));
#55181=CARTESIAN_POINT('Origin',(489.615917770968,-273.972007269816,-379.220287241448));
#55182=CARTESIAN_POINT('',(489.615917770967,-269.972007269816,-379.220287241453));
#55183=CARTESIAN_POINT('Origin',(489.615917770968,-273.972007269816,-379.220287241448));
#55184=CARTESIAN_POINT('',(489.615917770967,-269.972007269823,-384.220287241453));
#55185=CARTESIAN_POINT('',(489.615917770967,-269.972007269816,-379.220287241453));
#55186=CARTESIAN_POINT('Origin',(489.615917770968,-273.972007269823,-384.220287241448));
#55187=CARTESIAN_POINT('Origin',(457.615917770968,-269.972007269816,-379.220287241453));
#55188=CARTESIAN_POINT('',(457.615917770968,-269.972007269816,-379.220287241453));
#55189=CARTESIAN_POINT('',(465.615917770966,-269.972007269816,-379.220287241453));
#55190=CARTESIAN_POINT('',(457.615917770968,-269.972007269823,-384.220287241453));
#55191=CARTESIAN_POINT('',(457.615917770968,-269.972007269816,-379.220287241453));
#55192=CARTESIAN_POINT('',(465.615917770966,-269.972007269823,-384.220287241453));
#55193=CARTESIAN_POINT('Origin',(457.615917770968,-273.972007269816,-379.220287241447));
#55194=CARTESIAN_POINT('',(453.615917770968,-273.972007269816,-379.220287241447));
#55195=CARTESIAN_POINT('Origin',(457.615917770968,-273.972007269816,-379.220287241447));
#55196=CARTESIAN_POINT('',(453.615917770968,-273.972007269823,-384.220287241447));
#55197=CARTESIAN_POINT('',(453.615917770968,-273.972007269816,-379.220287241447));
#55198=CARTESIAN_POINT('Origin',(457.615917770968,-273.972007269823,-384.220287241447));
#55199=CARTESIAN_POINT('Origin',(453.615917770968,-305.972007269816,-379.220287241401));
#55200=CARTESIAN_POINT('',(453.615917770968,-297.972007269816,-379.220287241413));
#55201=CARTESIAN_POINT('',(453.615917770968,-297.972007269823,-384.220287241413));
#55202=CARTESIAN_POINT('Origin',(457.615917770968,-273.972007269816,-379.220287241447));
#55203=CARTESIAN_POINT('',(457.615917770945,-249.972007269814,-379.220287241482));
#55204=CARTESIAN_POINT('',(433.615917770966,-273.972007269756,-379.220287241447));
#55205=CARTESIAN_POINT('Origin',(457.615917770968,-273.972007269816,-379.220287241447));
#55206=CARTESIAN_POINT('',(457.615917770945,-249.972007269821,-384.220287241482));
#55207=CARTESIAN_POINT('',(457.615917770945,-249.972007269814,-379.220287241482));
#55208=CARTESIAN_POINT('',(433.615917770966,-273.972007269763,-384.220287241447));
#55209=CARTESIAN_POINT('Origin',(457.615917770968,-273.972007269823,-384.220287241447));
#55210=CARTESIAN_POINT('',(433.615917770966,-273.972007269756,-379.220287241447));
#55211=CARTESIAN_POINT('Origin',(433.615917770966,-305.972007269872,-379.220287241401));
#55212=CARTESIAN_POINT('',(433.615917770966,-305.972007269872,-379.220287241401));
#55213=CARTESIAN_POINT('',(433.615917770966,-273.972007269756,-379.220287241447));
#55214=CARTESIAN_POINT('',(433.615917770966,-305.972007269879,-384.220287241401));
#55215=CARTESIAN_POINT('',(433.615917770966,-273.972007269763,-384.220287241447));
#55216=CARTESIAN_POINT('',(433.615917770966,-305.972007269872,-379.220287241401));
#55217=CARTESIAN_POINT('Origin',(457.615917770968,-305.972007269816,-379.220287241401));
#55218=CARTESIAN_POINT('',(457.615917770945,-329.972007269817,-379.220287241366));
#55219=CARTESIAN_POINT('Origin',(457.615917770968,-305.972007269816,-379.220287241401));
#55220=CARTESIAN_POINT('',(457.615917770945,-329.972007269824,-384.220287241366));
#55221=CARTESIAN_POINT('Origin',(457.615917770968,-305.972007269823,-384.220287241401));
#55222=CARTESIAN_POINT('',(457.615917770945,-329.972007269817,-379.220287241366));
#55223=CARTESIAN_POINT('Origin',(489.615917770916,-329.972007269817,-379.220287241366));
#55224=CARTESIAN_POINT('',(489.615917770916,-329.972007269817,-379.220287241366));
#55225=CARTESIAN_POINT('',(457.615917770945,-329.972007269817,-379.220287241366));
#55226=CARTESIAN_POINT('',(489.615917770916,-329.972007269824,-384.220287241366));
#55227=CARTESIAN_POINT('',(457.615917770945,-329.972007269824,-384.220287241366));
#55228=CARTESIAN_POINT('',(489.615917770916,-329.972007269817,-379.220287241366));
#55229=CARTESIAN_POINT('Origin',(489.615917770968,-305.972007269816,-379.220287241401));
#55230=CARTESIAN_POINT('',(513.615917770969,-305.972007269872,-379.220287241401));
#55231=CARTESIAN_POINT('Origin',(489.615917770968,-305.972007269816,-379.220287241401));
#55232=CARTESIAN_POINT('',(513.615917770969,-305.972007269879,-384.220287241401));
#55233=CARTESIAN_POINT('Origin',(489.615917770968,-305.972007269823,-384.220287241401));
#55234=CARTESIAN_POINT('',(513.615917770969,-305.972007269872,-379.220287241401));
#55235=CARTESIAN_POINT('Origin',(513.615917770969,-273.972007269756,-379.220287241448));
#55236=CARTESIAN_POINT('',(513.615917770969,-273.972007269756,-379.220287241448));
#55237=CARTESIAN_POINT('',(513.615917770969,-305.972007269872,-379.220287241401));
#55238=CARTESIAN_POINT('',(513.615917770969,-273.972007269763,-384.220287241448));
#55239=CARTESIAN_POINT('',(513.615917770969,-305.972007269879,-384.220287241401));
#55240=CARTESIAN_POINT('',(513.615917770969,-273.972007269756,-379.220287241448));
#55241=CARTESIAN_POINT('Origin',(489.615917770968,-273.972007269816,-379.220287241448));
#55242=CARTESIAN_POINT('',(489.615917770916,-249.972007269814,-379.220287241482));
#55243=CARTESIAN_POINT('Origin',(489.615917770968,-273.972007269816,-379.220287241448));
#55244=CARTESIAN_POINT('',(489.615917770916,-249.972007269821,-384.220287241482));
#55245=CARTESIAN_POINT('Origin',(489.615917770968,-273.972007269823,-384.220287241448));
#55246=CARTESIAN_POINT('',(489.615917770916,-249.972007269814,-379.220287241482));
#55247=CARTESIAN_POINT('Origin',(457.615917770945,-249.972007269814,-379.220287241482));
#55248=CARTESIAN_POINT('',(489.615917770916,-249.972007269814,-379.220287241482));
#55249=CARTESIAN_POINT('',(489.615917770916,-249.972007269821,-384.220287241482));
#55250=CARTESIAN_POINT('Origin',(473.615917770965,-289.972007269816,-379.220287241424));
#55251=CARTESIAN_POINT('Origin',(473.615917770965,-289.972007269823,-384.220287241424));
#61761=UNCERTAINTY_MEASURE_WITH_UNIT(LENGTH_MEASURE(0.01),#61812,
'DISTANCE_ACCURACY_VALUE',
'Maximum model space distance between geometric entities at asserted c
onnectivities');
#61780=UNCERTAINTY_MEASURE_WITH_UNIT(LENGTH_MEASURE(0.01),#61812,
'DISTANCE_ACCURACY_VALUE',
'Maximum model space distance between geometric entities at asserted c
onnectivities');
#61792=(
GEOMETRIC_REPRESENTATION_CONTEXT(3)
GLOBAL_UNCERTAINTY_ASSIGNED_CONTEXT((#61761))
GLOBAL_UNIT_ASSIGNED_CONTEXT((#61812,#61814,#61815))
REPRESENTATION_CONTEXT('','3D')
);
#61811=(
GEOMETRIC_REPRESENTATION_CONTEXT(3)
GLOBAL_UNCERTAINTY_ASSIGNED_CONTEXT((#61780))
GLOBAL_UNIT_ASSIGNED_CONTEXT((#61812,#61814,#61815))
REPRESENTATION_CONTEXT('','3D')
);
#61812=(
LENGTH_UNIT()
NAMED_UNIT(*)
SI_UNIT(.MILLI.,.METRE.)
);
#61814=(
NAMED_UNIT(*)
PLANE_ANGLE_UNIT()
SI_UNIT($,.RADIAN.)
);
#61815=(
NAMED_UNIT(*)
SI_UNIT($,.STERADIAN.)
SOLID_ANGLE_UNIT()
);
#61827=SHAPE_DEFINITION_REPRESENTATION(#61857,#61979);
#61857=PRODUCT_DEFINITION_SHAPE('',$,#62010);
#61979=SHAPE_REPRESENTATION('',(#35191),#61792);
#61998=PRODUCT_DEFINITION_CONTEXT('part definition',#62090,'design');
#62010=PRODUCT_DEFINITION('Machine Frame Stand','Machine Frame Stand',#62040,
#61998);
#62040=PRODUCT_DEFINITION_FORMATION('',$,#62103);
#62090=APPLICATION_CONTEXT('Managed model based 3d engineering');
#62091=PRODUCT_CONTEXT('part definition',#62090,'mechanical');
#62103=PRODUCT('Machine Frame Stand','Machine Frame Stand',$,(#62091));
#62129=COLOUR_RGB('Dark Blue',0.08,0.2,0.34);
#62130=FILL_AREA_STYLE_COLOUR('',#62129);
#62131=FILL_AREA_STYLE('',(#62130));
#62132=SURFACE_STYLE_FILL_AREA(#62131);
#62133=SURFACE_SIDE_STYLE('',(#62132));
#62134=SURFACE_STYLE_USAGE(.BOTH.,#62133);
#62135=PRESENTATION_STYLE_ASSIGNMENT((#62134));
ENDSEC;
END-ISO-10303-21;
